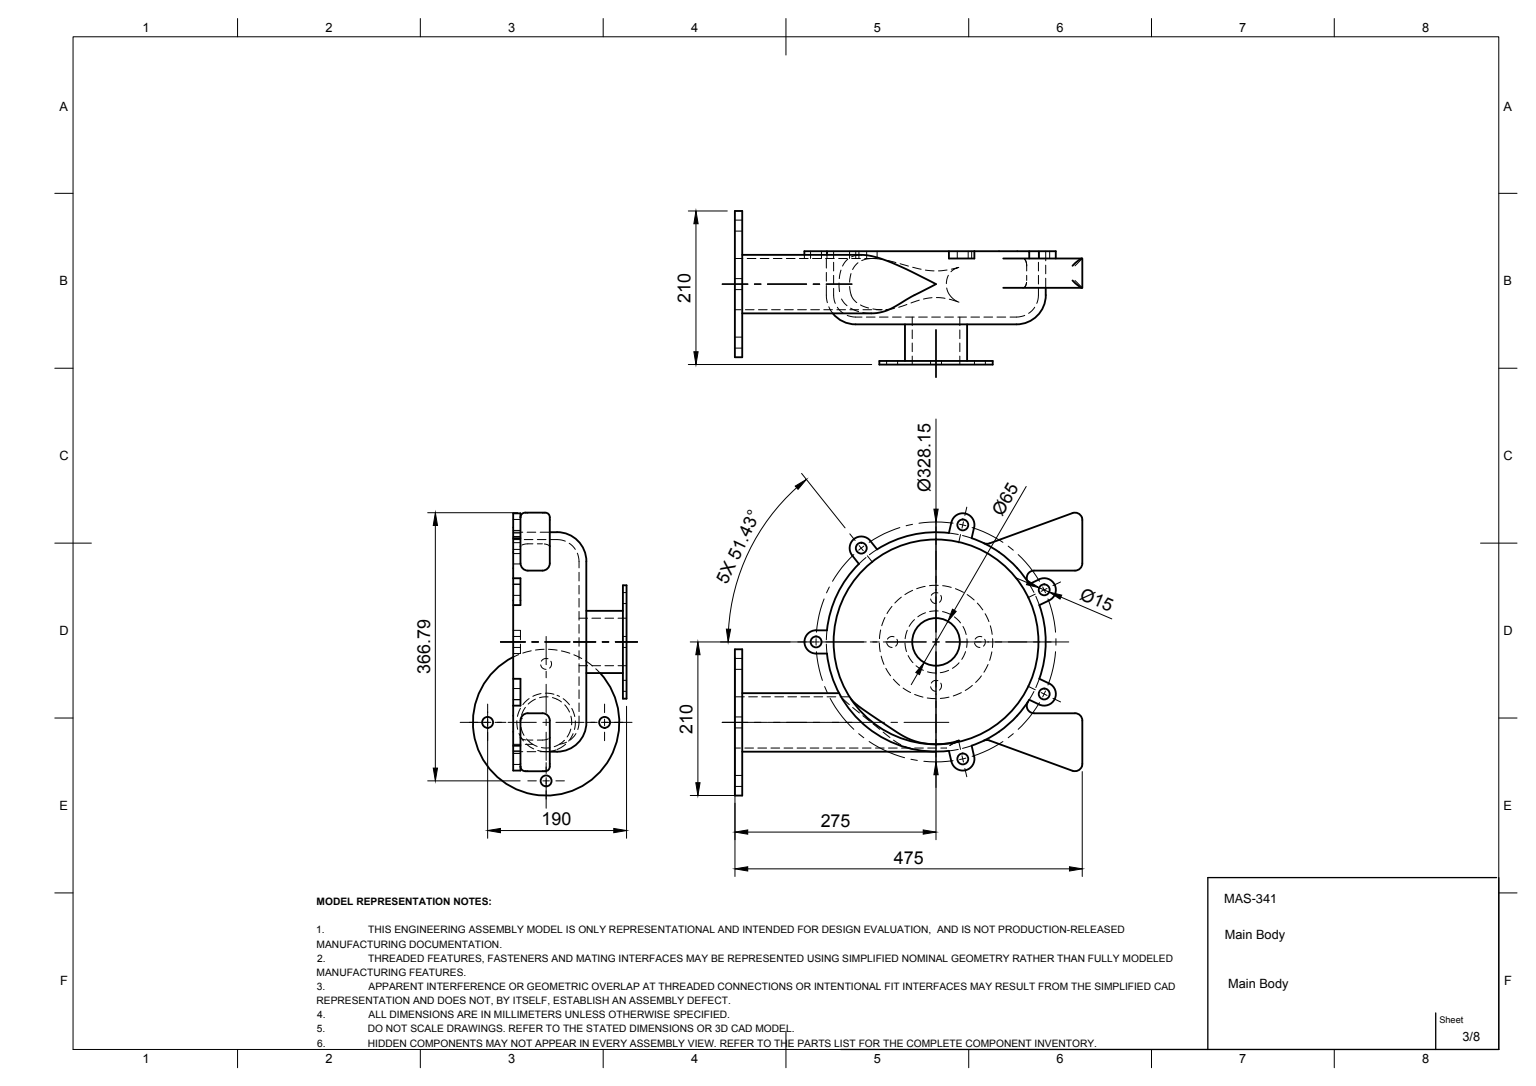
ISO-10303-21;
HEADER;
FILE_DESCRIPTION (('STEP AP214'),
    '1' );
FILE_NAME ('Main Body.step',
    '2026-10-08T00:39:10',
    ( '' ),
    ( '' ),
    'SwSTEP 2.0',
    'SolidWorks 2025',
    '' );
FILE_SCHEMA (( 'AUTOMOTIVE_DESIGN' ));
ENDSEC;

DATA;
#2=CARTESIAN_POINT ( 'NONE',  ( 97.60910239587762760, -133.8115172545202540, 8.514989709614523505 ) ) ;
#5=EDGE_CURVE ( 'NONE', #5734, #13358, #17540, .T. ) ;
#7=DIRECTION ( 'NONE',  ( 0.000000000000000000, 0.000000000000000000, 1.000000000000000000 ) ) ;
#9=CARTESIAN_POINT ( 'NONE',  ( 0.000000000000000000, 0.000000000000000000, 49.99999999999999289 ) ) ;
#16=CARTESIAN_POINT ( 'NONE',  ( 95.93567628220807819, -116.0760901523964179, 30.45195958925782520 ) ) ;
#22=VERTEX_POINT ( 'NONE', #7636 ) ;
#26=CARTESIAN_POINT ( 'NONE',  ( 78.68887634719571622, -147.8252249328912740, 39.99999999999999289 ) ) ;
#29=VECTOR ( 'NONE', #19093, 1000.000000000000000 ) ;
#30=DIRECTION ( 'NONE',  ( 0.000000000000000000, 0.000000000000000000, 1.000000000000000000 ) ) ;
#31=FACE_OUTER_BOUND ( 'NONE', #4493, .T. ) ;
#32=CARTESIAN_POINT ( 'NONE',  ( 130.7934332354521132, -73.44669674648567081, 45.54261232719608188 ) ) ;
#33=CARTESIAN_POINT ( 'NONE',  ( -84.44661573609343463, -123.9709896190455680, 39.82577217277482617 ) ) ;
#38=CARTESIAN_POINT ( 'NONE',  ( -139.9569363493348249, 3.997132000652560802, 23.09995224052206453 ) ) ;
#42=CARTESIAN_POINT ( 'NONE',  ( -133.8587666923834547, -78.85012038918891619, 37.00472930354037260 ) ) ;
#44=ORIENTED_EDGE ( 'NONE', *, *, #7876, .F. ) ;
#51=CARTESIAN_POINT ( 'NONE',  ( -144.9440567817290741, -14.18564734370175628, 2.776575249912347054 ) ) ;
#56=CARTESIAN_POINT ( 'NONE',  ( -95.11181282143326143, 95.73178764297979626, -26.71222966351301409 ) ) ;
#58=DIRECTION ( 'NONE',  ( -0.000000000000000000, -0.000000000000000000, -1.000000000000000000 ) ) ;
#63=CARTESIAN_POINT ( 'NONE',  ( 134.0645693066686874, -77.56608579646832879, 36.26849213499117042 ) ) ;
#64=CARTESIAN_POINT ( 'NONE',  ( -109.9999999999983515, 275.0000000000000000, 92.50000000000004263 ) ) ;
#65=VERTEX_POINT ( 'NONE', #17476 ) ;
#68=ORIENTED_EDGE ( 'NONE', *, *, #8619, .T. ) ;
#70=VECTOR ( 'NONE', #7904, 1000.000000000000000 ) ;
#76=CARTESIAN_POINT ( 'NONE',  ( 152.4599531637113330, -36.50981547336952104, 49.99999999999999289 ) ) ;
#82=CARTESIAN_POINT ( 'NONE',  ( -82.22709333324932857, 122.5189358644918656, -23.80566512433226833 ) ) ;
#83=CARTESIAN_POINT ( 'NONE',  ( -110.0000000000000142, 275.0000000000000000, 5.000000000000000888 ) ) ;
#84=EDGE_CURVE ( 'NONE', #13974, #7495, #15567, .T. ) ;
#86=VECTOR ( 'NONE', #18456, 1000.000000000000000 ) ;
#87=AXIS2_PLACEMENT_3D ( 'NONE', #5255, #2475, #14657 ) ;
#88=LINE ( 'NONE', #6338, #12972 ) ;
#90=CARTESIAN_POINT ( 'NONE',  ( -56.84754764479025368, -154.7316448359455308, 49.99999999999999289 ) ) ;
#102=CARTESIAN_POINT ( 'NONE',  ( 100.3336596192663990, -130.0766330735003180, 3.023488127333376685 ) ) ;
#112=CARTESIAN_POINT ( 'NONE',  ( 96.87131796860539623, -115.7364764686970489, 29.66028648393937317 ) ) ;
#114=DIRECTION ( 'NONE',  ( -3.129754055707530415E-16, 1.000000000000000000, 0.000000000000000000 ) ) ;
#115=CARTESIAN_POINT ( 'NONE',  ( -70.46379820184749576, 132.4194400891323653, -1.343775461033565932 ) ) ;
#117=ORIENTED_EDGE ( 'NONE', *, *, #11334, .T. ) ;
#127=VECTOR ( 'NONE', #6121, 1000.000000000000000 ) ;
#128=ORIENTED_EDGE ( 'NONE', *, *, #9739, .T. ) ;
#130=DIRECTION ( 'NONE',  ( 0.000000000000000000, 1.000000000000000000, 0.000000000000000000 ) ) ;
#132=CARTESIAN_POINT ( 'NONE',  ( -95.59344839194261567, -116.1516065318577233, 31.25619608454541165 ) ) ;
#134=CARTESIAN_POINT ( 'NONE',  ( -140.0000000000000284, 1.714505518806295230E-14, 23.02775637731986436 ) ) ;
#140=CARTESIAN_POINT ( 'NONE',  ( -123.8565975624213849, -84.62454961663081576, 40.61527585688936881 ) ) ;
#147=EDGE_LOOP ( 'NONE', ( #10880, #3979, #3844, #3785, #18936 ) ) ;
#152=CARTESIAN_POINT ( 'NONE',  ( -144.3459975433503359, -14.90824844061875432, 11.80575795572019437 ) ) ;
#156=CARTESIAN_POINT ( 'NONE',  ( -77.50000000000000000, 9.491012693391988181E-15, -105.0000000000000142 ) ) ;
#160=CARTESIAN_POINT ( 'NONE',  ( 104.3997176008718668, -123.8500140569468897, 39.51069475786240304 ) ) ;
#164=CARTESIAN_POINT ( 'NONE',  ( 131.4393841463105730, -72.38802639019482399, 37.47509838629414247 ) ) ;
#165=CARTESIAN_POINT ( 'NONE',  ( -97.49999999999997158, -195.8578643762690206, 4.142135623730952787 ) ) ;
#178=CARTESIAN_POINT ( 'NONE',  ( -85.53020504959707182, -140.9188050298390067, 49.99999999999999289 ) ) ;
#180=CARTESIAN_POINT ( 'NONE',  ( 125.6254798881099362, -81.96796683352708612, -9.529669441935290308 ) ) ;
#183=DIRECTION ( 'NONE',  ( -0.000000000000000000, -1.000000000000000000, -0.000000000000000000 ) ) ;
#189=CARTESIAN_POINT ( 'NONE',  ( 89.20186311087663000, -120.5960167300875980, 45.74363724982469392 ) ) ;
#190=ORIENTED_EDGE ( 'NONE', *, *, #18942, .F. ) ;
#191=CARTESIAN_POINT ( 'NONE',  ( -7.500000000000006217, 164.0736214083062805, 49.99999999999999289 ) ) ;
#196=VECTOR ( 'NONE', #6508, 1000.000000000000000 ) ;
#206=LINE ( 'NONE', #17312, #2056 ) ;
#213=CARTESIAN_POINT ( 'NONE',  ( -71.48370871149657546, 131.8717905529093173, 15.83076793550482542 ) ) ;
#220=EDGE_CURVE ( 'NONE', #5955, #14128, #18233, .T. ) ;
#222=CARTESIAN_POINT ( 'NONE',  ( -139.5020293846663435, 55.14116363050599290, 32.01918336342640004 ) ) ;
#224=FACE_OUTER_BOUND ( 'NONE', #2485, .T. ) ;
#225=LINE ( 'NONE', #20072, #5672 ) ;
#226=CARTESIAN_POINT ( 'NONE',  ( 134.9252074077220129, -65.53799637400003064, 33.62285034463288724 ) ) ;
#228=CARTESIAN_POINT ( 'NONE',  ( -96.81625497257122959, -114.6298681929799557, 36.57121525224014391 ) ) ;
#230=CARTESIAN_POINT ( 'NONE',  ( -90.17913298585699522, -119.8669913176027961, -6.508363994189858559 ) ) ;
#231=DIRECTION ( 'NONE',  ( 0.000000000000000000, 0.000000000000000000, 1.000000000000000000 ) ) ;
#237=EDGE_CURVE ( 'NONE', #5955, #1847, #14266, .T. ) ;
#240=CARTESIAN_POINT ( 'NONE',  ( -133.3512892972259749, -81.69145041113908690, 38.21234876929968038 ) ) ;
#242=EDGE_CURVE ( 'NONE', #7766, #5287, #5764, .T. ) ;
#245=AXIS2_PLACEMENT_3D ( 'NONE', #14497, #6431, #6630 ) ;
#251=CARTESIAN_POINT ( 'NONE',  ( -142.2837698990419710, -17.71062413665211466, 18.52607103759555685 ) ) ;
#260=FACE_OUTER_BOUND ( 'NONE', #11432, .T. ) ;
#265=CARTESIAN_POINT ( 'NONE',  ( 134.2531151303012109, -76.34772591579755385, 35.47645838411665409 ) ) ;
#266=CARTESIAN_POINT ( 'NONE',  ( 132.1955596402976596, -87.17962382538661359, 39.63083459970911804 ) ) ;
#267=ORIENTED_EDGE ( 'NONE', *, *, #4626, .T. ) ;
#269=VERTEX_POINT ( 'NONE', #14956 ) ;
#272=EDGE_CURVE ( 'NONE', #301, #10908, #19490, .T. ) ;
#278=CIRCLE ( 'NONE', #5508, 7.500000000000020428 ) ;
#284=ORIENTED_EDGE ( 'NONE', *, *, #8836, .T. ) ;
#287=EDGE_CURVE ( 'NONE', #13667, #5147, #20127, .T. ) ;
#291=DIRECTION ( 'NONE',  ( -1.000000000000000000, 0.000000000000000000, 0.000000000000000000 ) ) ;
#293=AXIS2_PLACEMENT_3D ( 'NONE', #9235, #1570, #18553 ) ;
#301=VERTEX_POINT ( 'NONE', #13513 ) ;
#303=CARTESIAN_POINT ( 'NONE',  ( 15.91767397667354800, 164.0736214083062805, 39.99999999999999289 ) ) ;
#307=AXIS2_PLACEMENT_3D ( 'NONE', #2543, #16563, #13781 ) ;
#308=CARTESIAN_POINT ( 'NONE',  ( -109.9999999999983515, 275.0000000000000000, 92.50000000000004263 ) ) ;
#309=CARTESIAN_POINT ( 'NONE',  ( -97.49999999999997158, -190.0000000000000000, 10.00000000000000178 ) ) ;
#310=ORIENTED_EDGE ( 'NONE', *, *, #14972, .F. ) ;
#314=CARTESIAN_POINT ( 'NONE',  ( 106.3852469178137170, -120.5001569748608432, 39.95380131650621536 ) ) ;
#317=CARTESIAN_POINT ( 'NONE',  ( -85.08865936083807924, 123.5409191676841374, 36.33575822748944972 ) ) ;
#318=EDGE_LOOP ( 'NONE', ( #10849, #15517, #10410, #10745 ) ) ;
#324=ORIENTED_EDGE ( 'NONE', *, *, #14683, .T. ) ;
#326=CARTESIAN_POINT ( 'NONE',  ( -149.9999999999999716, 1.115331095350416746, 5.575954458838749517 ) ) ;
#330=CARTESIAN_POINT ( 'NONE',  ( 132.6585078626522716, -70.01400725886476550, 42.31265725997803884 ) ) ;
#331=VECTOR ( 'NONE', #5545, 1000.000000000000000 ) ;
#333=CARTESIAN_POINT ( 'NONE',  ( -89.20186311087657316, -120.5960167300876407, -5.743637249824701918 ) ) ;
#346=EDGE_CURVE ( 'NONE', #17320, #3067, #19461, .T. ) ;
#353=CARTESIAN_POINT ( 'NONE',  ( -29.99999999999887379, 265.0000000000000000, 12.49999999999916511 ) ) ;
#356=FACE_OUTER_BOUND ( 'NONE', #14079, .T. ) ;
#358=AXIS2_PLACEMENT_3D ( 'NONE', #19876, #8929, #1155 ) ;
#365=CIRCLE ( 'NONE', #11782, 77.50000000000000000 ) ;
#375=B_SPLINE_CURVE_WITH_KNOTS ( 'NONE', 3,
 ( #12809, #14142, #6181, #4742, #226, #1768, #17536, #3410, #17117, #330, #12398, #9642, #6588, #32, #9545, #19072, #8099, #14247, #3103, #15890, #18860, #4637, #17333, #1869 ),
 .UNSPECIFIED., .F., .F.,
 ( 4, 2, 2, 2, 2, 2, 2, 2, 2, 2, 2, 4 ),
 ( 0.000000000000000000, 0.002185557465519395465, 0.004371114931038790931, 0.008742229862077573188, 0.01311334479311635458, 0.01529890225863574441, 0.01748445972415513250, 0.02185557465519396420, 0.02404113212071339739, 0.02622668958623283059, 0.03059780451727174902, 0.03496891944831063970 ),
 .UNSPECIFIED. ) ;
#380=VERTEX_POINT ( 'NONE', #4526 ) ;
#381=CARTESIAN_POINT ( 'NONE',  ( 133.7324673749508577, -67.93981414779143790, 0.4927691020655204368 ) ) ;
#383=VERTEX_POINT ( 'NONE', #14037 ) ;
#388=EDGE_CURVE ( 'NONE', #16701, #14351, #10960, .T. ) ;
#393=CARTESIAN_POINT ( 'NONE',  ( -141.8714406926361278, -48.70825716237272474, 39.99999999999999289 ) ) ;
#394=VECTOR ( 'NONE', #11693, 1000.000000000000114 ) ;
#395=ORIENTED_EDGE ( 'NONE', *, *, #3158, .T. ) ;
#397=CARTESIAN_POINT ( 'NONE',  ( 0.000000000000000000, 0.000000000000000000, 49.99999999999999289 ) ) ;
#398=EDGE_CURVE ( 'NONE', #9612, #14697, #17220, .T. ) ;
#406=DIRECTION ( 'NONE',  ( -1.000000000000000000, 0.000000000000000000, 0.000000000000000000 ) ) ;
#409=AXIS2_PLACEMENT_3D ( 'NONE', #4331, #19177, #450 ) ;
#410=VECTOR ( 'NONE', #17095, 1000.000000000000000 ) ;
#415=ADVANCED_FACE ( 'NONE', ( #433 ), #17632, .T. ) ;
#418=CARTESIAN_POINT ( 'NONE',  ( -107.4999999999999716, -200.0000000000000000, 40.00000000000000000 ) ) ;
#424=ORIENTED_EDGE ( 'NONE', *, *, #11382, .F. ) ;
#433=FACE_OUTER_BOUND ( 'NONE', #9062, .T. ) ;
#436=FACE_OUTER_BOUND ( 'NONE', #18488, .T. ) ;
#437=CARTESIAN_POINT ( 'NONE',  ( -98.17258311761709422, -133.0662226711790197, 6.375986368445647479 ) ) ;
#438=EDGE_CURVE ( 'NONE', #5218, #9870, #5431, .T. ) ;
#440=CARTESIAN_POINT ( 'NONE',  ( -122.1025966345561073, 68.49760859473882135, 37.84499468909948661 ) ) ;
#447=DIRECTION ( 'NONE',  ( -1.000000000000000000, 0.000000000000000000, 0.000000000000000000 ) ) ;
#450=DIRECTION ( 'NONE',  ( 0.000000000000000000, 0.000000000000000000, -1.000000000000000000 ) ) ;
#455=ORIENTED_EDGE ( 'NONE', *, *, #13971, .F. ) ;
#458=CARTESIAN_POINT ( 'NONE',  ( -189.9999999999988916, 275.0000000000000000, 5.000000000000268230 ) ) ;
#464=CARTESIAN_POINT ( 'NONE',  ( 0.000000000000000000, 0.000000000000000000, -10.00000000000000178 ) ) ;
#471=ORIENTED_EDGE ( 'NONE', *, *, #8214, .T. ) ;
#476=EDGE_LOOP ( 'NONE', ( #2456, #12768 ) ) ;
#483=ORIENTED_EDGE ( 'NONE', *, *, #16283, .F. ) ;
#484=CARTESIAN_POINT ( 'NONE',  ( 134.7540465048387546, -65.88919983460813512, 5.016205221822248816 ) ) ;
#489=AXIS2_PLACEMENT_3D ( 'NONE', #7649, #18713, #18610 ) ;
#494=CARTESIAN_POINT ( 'NONE',  ( -135.7837464099825695, -28.85345328491248651, -18.68477101865893175 ) ) ;
#496=CARTESIAN_POINT ( 'NONE',  ( 93.27226090021298432, -117.4765369300808402, 48.33671567152951098 ) ) ;
#497=ORIENTED_EDGE ( 'NONE', *, *, #17432, .F. ) ;
#505=EDGE_LOOP ( 'NONE', ( #8299, #8837, #2752, #9090 ) ) ;
#510=DIRECTION ( 'NONE',  ( -0.000000000000000000, -0.000000000000000000, -1.000000000000000000 ) ) ;
#513=PRODUCT ( 'Main Body', 'Main Body', '', ( #19350 ) ) ;
#514=DIRECTION ( 'NONE',  ( 1.000000000000000000, 0.000000000000000000, 0.000000000000000000 ) ) ;
#519=CARTESIAN_POINT ( 'NONE',  ( 0.000000000000000000, 164.0736214083062805, 39.99999999999999289 ) ) ;
#527=CARTESIAN_POINT ( 'NONE',  ( -88.95069649744878859, 120.7914063265062055, 39.04816013673605113 ) ) ;
#532=ORIENTED_EDGE ( 'NONE', *, *, #2284, .F. ) ;
#536=CARTESIAN_POINT ( 'NONE',  ( -113.3498877299711864, 98.27513227905838278, 44.89206021334695862 ) ) ;
#540=CARTESIAN_POINT ( 'NONE',  ( -97.52847697650713599, -113.9950050385133693, 2.467650561764177741 ) ) ;
#546=CARTESIAN_POINT ( 'NONE',  ( 159.9599531637113330, -36.50981547336952104, 39.99999999999999289 ) ) ;
#548=EDGE_CURVE ( 'NONE', #12640, #16017, #8706, .T. ) ;
#566=CARTESIAN_POINT ( 'NONE',  ( 140.0000000000000284, 0.000000000000000000, -115.0000000000000142 ) ) ;
#567=PLANE ( 'NONE',  #6525 ) ;
#571=ORIENTED_EDGE ( 'NONE', *, *, #2295, .T. ) ;
#573=VERTEX_POINT ( 'NONE', #17823 ) ;
#575=ORIENTED_EDGE ( 'NONE', *, *, #4277, .F. ) ;
#578=DIRECTION ( 'NONE',  ( 0.9749279121818257288, -0.2225209339563047339, 0.000000000000000000 ) ) ;
#583=ORIENTED_EDGE ( 'NONE', *, *, #19634, .T. ) ;
#584=CARTESIAN_POINT ( 'NONE',  ( -93.38451287766530129, 109.3625709609712544, -31.42891559531335588 ) ) ;
#588=CARTESIAN_POINT ( 'NONE',  ( -136.9468171063203101, -26.51361207507547491, -17.34057338814886862 ) ) ;
#590=CARTESIAN_POINT ( 'NONE',  ( 99.70727046260189752, -112.0668231182905572, 49.97544513886636963 ) ) ;
#592=EDGE_CURVE ( 'NONE', #9122, #5287, #632, .T. ) ;
#602=CARTESIAN_POINT ( 'NONE',  ( -82.33470881469955316, -125.3834122142802272, 33.60191280747055487 ) ) ;
#608=CARTESIAN_POINT ( 'NONE',  ( 104.1558342746901928, -124.2522228486704421, 0.5619391425930568840 ) ) ;
#614=AXIS2_PLACEMENT_3D ( 'NONE', #2103, #14577, #4975 ) ;
#616=DIRECTION ( 'NONE',  ( 0.000000000000000000, 0.000000000000000000, 1.000000000000000000 ) ) ;
#618=CARTESIAN_POINT ( 'NONE',  ( 93.45568245711652366, -117.3306176392091373, 48.42050290853573102 ) ) ;
#620=ADVANCED_FACE ( 'NONE', ( #10231 ), #2366, .T. ) ;
#622=FACE_OUTER_BOUND ( 'NONE', #12847, .T. ) ;
#632=LINE ( 'NONE', #19353, #1191 ) ;
#637=CARTESIAN_POINT ( 'NONE',  ( -95.49560220037844260, -115.9193184531315381, 6.561900623234592445 ) ) ;
#645=AXIS2_PLACEMENT_3D ( 'NONE', #919, #2868, #2668 ) ;
#649=EDGE_CURVE ( 'NONE', #11180, #14061, #3174, .T. ) ;
#654=ADVANCED_FACE ( 'NONE', ( #7666 ), #12466, .F. ) ;
#655=DIRECTION ( 'NONE',  ( -0.000000000000000000, -1.000000000000000000, -0.000000000000000000 ) ) ;
#657=CARTESIAN_POINT ( 'NONE',  ( -126.0064496073183591, -81.39031533630314641, -9.417289231373237257 ) ) ;
#659=CARTESIAN_POINT ( 'NONE',  ( -136.4994460260996902, -31.11111111111110006, -10.83394172763413899 ) ) ;
#663=CARTESIAN_POINT ( 'NONE',  ( -129.0037046021669767, -76.61892870327682203, -0.1306340574592130821 ) ) ;
#664=CARTESIAN_POINT ( 'NONE',  ( 134.6385828715892217, -73.56429320930371318, 7.599106732516738738 ) ) ;
#666=CARTESIAN_POINT ( 'NONE',  ( -176.7850001792984358, -194.3449193228699414, 2.490758961397592675 ) ) ;
#669=ORIENTED_EDGE ( 'NONE', *, *, #5124, .F. ) ;
#672=VECTOR ( 'NONE', #9418, 1000.000000000000000 ) ;
#674=ORIENTED_EDGE ( 'NONE', *, *, #4626, .F. ) ;
#679=LINE ( 'NONE', #6924, #9296 ) ;
#681=ORIENTED_EDGE ( 'NONE', *, *, #13967, .F. ) ;
#686=EDGE_LOOP ( 'NONE', ( #4759, #20168, #5378, #19082, #13161, #7782, #5172, #267, #1533, #7449, #5941, #583, #3735, #5761, #17193, #6714, #16858, #15007, #1728, #12781, #8037, #18671, #16578, #19251, #1715, #18339, #12228, #4895, #11794, #7815, #748, #14906, #395 ) ) ;
#696=DIRECTION ( 'NONE',  ( 0.7818314824680220321, 0.6234898018587433643, 0.000000000000000000 ) ) ;
#700=ORIENTED_EDGE ( 'NONE', *, *, #19231, .F. ) ;
#701=LINE ( 'NONE', #8276, #10766 ) ;
#708=CARTESIAN_POINT ( 'NONE',  ( 103.6579813550140017, -125.0534741538843235, 0.7510394427105699933 ) ) ;
#713=CARTESIAN_POINT ( 'NONE',  ( 97.50000000000001421, -133.9542832461881119, 30.00000000000000000 ) ) ;
#714=CARTESIAN_POINT ( 'NONE',  ( 82.22461745850688430, -125.4556360547411344, 7.112305957179646754 ) ) ;
#722=CARTESIAN_POINT ( 'NONE',  ( 101.0196388379316659, 100.9199429146863167, 49.99999999999999289 ) ) ;
#727=CARTESIAN_POINT ( 'NONE',  ( 96.59911734864401467, -114.8254675080909095, 3.766286132638113848 ) ) ;
#729=CARTESIAN_POINT ( 'NONE',  ( -95.77047472624724378, -116.1200526047209394, 9.227179618507987513 ) ) ;
#733=DIRECTION ( 'NONE',  ( -0.000000000000000000, -0.000000000000000000, -1.000000000000000000 ) ) ;
#737=CARTESIAN_POINT ( 'NONE',  ( -15.91767397667354800, 141.9028892025177413, 49.99999999999999289 ) ) ;
#740=EDGE_CURVE ( 'NONE', #961, #7600, #11543, .T. ) ;
#748=ORIENTED_EDGE ( 'NONE', *, *, #13971, .T. ) ;
#751=CARTESIAN_POINT ( 'NONE',  ( -126.7590367374602494, -80.21250349114244216, -9.076491356015703005 ) ) ;
#752=DIRECTION ( 'NONE',  ( 0.000000000000000000, 0.000000000000000000, 1.000000000000000000 ) ) ;
#753=CIRCLE ( 'NONE', #11206, 7.500000000000006217 ) ;
#755=DIRECTION ( 'NONE',  ( 0.3427509529624095941, 0.9394263059140722794, 0.000000000000000000 ) ) ;
#757=CARTESIAN_POINT ( 'NONE',  ( -77.50000000000000000, 9.491012693391988181E-15, -100.0000000000000000 ) ) ;
#762=EDGE_CURVE ( 'NONE', #18014, #5623, #16769, .T. ) ;
#766=CIRCLE ( 'NONE', #13818, 7.500000000000000000 ) ;
#768=ORIENTED_EDGE ( 'NONE', *, *, #10405, .F. ) ;
#771=AXIS2_PLACEMENT_3D ( 'NONE', #14466, #6901, #11492 ) ;
#776=DIRECTION ( 'NONE',  ( -0.000000000000000000, -0.000000000000000000, -1.000000000000000000 ) ) ;
#777=ORIENTED_EDGE ( 'NONE', *, *, #9922, .T. ) ;
#780=ORIENTED_EDGE ( 'NONE', *, *, #16980, .F. ) ;
#781=PLANE ( 'NONE',  #11393 ) ;
#789=ORIENTED_EDGE ( 'NONE', *, *, #13137, .T. ) ;
#796=VERTEX_POINT ( 'NONE', #3075 ) ;
#799=AXIS2_PLACEMENT_3D ( 'NONE', #5132, #17310, #9715 ) ;
#801=DIRECTION ( 'NONE',  ( -0.000000000000000000, -1.000000000000000000, -0.000000000000000000 ) ) ;
#803=CARTESIAN_POINT ( 'NONE',  ( -130.1901167961280521, -74.50443780700842922, 46.26218360866808865 ) ) ;
#804=CARTESIAN_POINT ( 'NONE',  ( 63.68887634719570912, -147.8252249328912740, 39.99999999999999289 ) ) ;
#808=CARTESIAN_POINT ( 'NONE',  ( -144.1130761623740568, -69.50842595698578918, 49.99999999999999289 ) ) ;
#810=CARTESIAN_POINT ( 'NONE',  ( 82.03125000000005684, -125.5821405433014064, 9.272053618398000907 ) ) ;
#817=VECTOR ( 'NONE', #13786, 999.9999999999998863 ) ;
#823=VECTOR ( 'NONE', #11548, 1000.000000000000000 ) ;
#824=CARTESIAN_POINT ( 'NONE',  ( 95.45795901651801785, -116.1130648478386007, 7.867509371635869719 ) ) ;
#825=CARTESIAN_POINT ( 'NONE',  ( -100.4426743477017965, -129.9257371803582259, 2.884579890773657507 ) ) ;
#827=CARTESIAN_POINT ( 'NONE',  ( -150.0000000000000284, 0.000000000000000000, 49.99999999999999289 ) ) ;
#830=DIRECTION ( 'NONE',  ( 0.000000000000000000, 0.000000000000000000, -1.000000000000000000 ) ) ;
#834=EDGE_LOOP ( 'NONE', ( #11102, #16029, #13341, #7575, #11239, #15936 ) ) ;
#836=DIRECTION ( 'NONE',  ( -0.000000000000000000, -0.000000000000000000, 1.000000000000000000 ) ) ;
#853=CARTESIAN_POINT ( 'NONE',  ( -130.9868171408399462, -91.88282611735539263, 3.469446951953614189E-15 ) ) ;
#855=CARTESIAN_POINT ( 'NONE',  ( 134.6061912685151754, -66.19056267105210623, 4.133867502762946344 ) ) ;
#866=EDGE_LOOP ( 'NONE', ( #10462, #13743, #13664, #7998 ) ) ;
#870=VERTEX_POINT ( 'NONE', #12780 ) ;
#871=ADVANCED_FACE ( 'NONE', ( #15659 ), #3279, .F. ) ;
#881=CARTESIAN_POINT ( 'NONE',  ( 4.189777606611760026E-13, -60.00000000000000000, -105.0000000000000142 ) ) ;
#886=ORIENTED_EDGE ( 'NONE', *, *, #1081, .F. ) ;
#888=DIRECTION ( 'NONE',  ( -0.000000000000000000, -1.000000000000000000, -0.000000000000000000 ) ) ;
#894=CARTESIAN_POINT ( 'NONE',  ( -84.48076729319791411, -123.9477347680102639, 39.88981094656359971 ) ) ;
#897=FACE_OUTER_BOUND ( 'NONE', #6117, .T. ) ;
#899=EDGE_CURVE ( 'NONE', #15648, #18566, #9811, .T. ) ;
#902=CARTESIAN_POINT ( 'NONE',  ( -134.6444961603440618, -66.11310837778573557, 35.67578572572296025 ) ) ;
#909=CARTESIAN_POINT ( 'NONE',  ( 82.17872144123518297, -125.4856950968007396, 7.470559115686841167 ) ) ;
#913=CIRCLE ( 'NONE', #9421, 99.99999999999997158 ) ;
#919=CARTESIAN_POINT ( 'NONE',  ( -107.4999999999999716, -190.0000000000000000, 40.00000000000000000 ) ) ;
#923=CARTESIAN_POINT ( 'NONE',  ( 96.59339607700708541, -114.7676973381603887, -9.527748193600634963 ) ) ;
#928=CARTESIAN_POINT ( 'NONE',  ( -86.48208760716207166, -122.5631135004756658, -3.009211076429890053 ) ) ;
#929=CARTESIAN_POINT ( 'NONE',  ( 107.5000000000000284, -199.9999999999999716, 40.00000000000000000 ) ) ;
#933=CARTESIAN_POINT ( 'NONE',  ( -139.8142396999972163, 1.712230611238718486E-14, -13.33333333333329307 ) ) ;
#935=DIRECTION ( 'NONE',  ( 0.000000000000000000, 0.000000000000000000, -1.000000000000000000 ) ) ;
#949=CIRCLE ( 'NONE', #5870, 15.91767397667354444 ) ;
#953=DIRECTION ( 'NONE',  ( 0.000000000000000000, 0.000000000000000000, 1.000000000000000000 ) ) ;
#954=CARTESIAN_POINT ( 'NONE',  ( 134.5971911056711292, -73.88063391573085426, 7.066933751406428321 ) ) ;
#956=CYLINDRICAL_SURFACE ( 'NONE', #3822, 7.500000000000006217 ) ;
#960=EDGE_CURVE ( 'NONE', #4825, #18093, #17397, .T. ) ;
#961=VERTEX_POINT ( 'NONE', #17797 ) ;
#962=AXIS2_PLACEMENT_3D ( 'NONE', #18141, #4121, #10352 ) ;
#969=ORIENTED_EDGE ( 'NONE', *, *, #14026, .F. ) ;
#970=CARTESIAN_POINT ( 'NONE',  ( 7.500000000000006217, 164.0736214083062805, 49.99999999999999289 ) ) ;
#973=ORIENTED_EDGE ( 'NONE', *, *, #19651, .F. ) ;
#975=CIRCLE ( 'NONE', #5896, 150.0000000000000284 ) ;
#977=CARTESIAN_POINT ( 'NONE',  ( 71.18887634719571622, -147.8252249328912740, 39.99999999999999289 ) ) ;
#983=ORIENTED_EDGE ( 'NONE', *, *, #5166, .F. ) ;
#986=ORIENTED_EDGE ( 'NONE', *, *, #13979, .T. ) ;
#1002=CARTESIAN_POINT ( 'NONE',  ( 77.50000000000000000, 0.000000000000000000, -105.0000000000000142 ) ) ;
#1010=LINE ( 'NONE', #19448, #1921 ) ;
#1015=EDGE_CURVE ( 'NONE', #3673, #7332, #3053, .T. ) ;
#1028=DIRECTION ( 'NONE',  ( -0.000000000000000000, -0.000000000000000000, 1.000000000000000000 ) ) ;
#1032=DIRECTION ( 'NONE',  ( 0.000000000000000000, 0.000000000000000000, 1.000000000000000000 ) ) ;
#1033=EDGE_CURVE ( 'NONE', #6085, #5634, #4169, .T. ) ;
#1038=ADVANCED_FACE ( 'NONE', ( #10705 ), #15108, .T. ) ;
#1039=DIRECTION ( 'NONE',  ( -1.000000000000000000, 0.000000000000000000, 0.000000000000000000 ) ) ;
#1040=ORIENTED_EDGE ( 'NONE', *, *, #237, .F. ) ;
#1041=CARTESIAN_POINT ( 'NONE',  ( 0.000000000000000000, 0.000000000000000000, -49.99999999999999289 ) ) ;
#1047=CARTESIAN_POINT ( 'NONE',  ( -127.6186898578139477, -78.88112642940109254, -0.7766205772862178058 ) ) ;
#1048=CARTESIAN_POINT ( 'NONE',  ( 131.2702496982006153, -90.86622748989321963, -2.335466277633964500E-16 ) ) ;
#1052=CARTESIAN_POINT ( 'NONE',  ( -133.2712073786778433, -68.96827650415615096, 31.07541976963426578 ) ) ;
#1054=MANIFOLD_SOLID_BREP ( 'Fillet3', #7080 ) ;
#1061=ORIENTED_EDGE ( 'NONE', *, *, #13864, .F. ) ;
#1069=LINE ( 'NONE', #4050, #15986 ) ;
#1070=CARTESIAN_POINT ( 'NONE',  ( 120.7779226595531128, 102.2982297021113141, 39.99999999999999289 ) ) ;
#1071=CARTESIAN_POINT ( 'NONE',  ( -42.50000000000000000, 5.204748896376250896E-15, -100.0000000000000000 ) ) ;
#1073=UNCERTAINTY_MEASURE_WITH_UNIT (LENGTH_MEASURE( 1.000000000000000082E-05 ), #7638, 'distance_accuracy_value', 'NONE');
#1074=VECTOR ( 'NONE', #12151, 1000.000000000000114 ) ;
#1075=CARTESIAN_POINT ( 'NONE',  ( 130.6671641404130639, -73.67117004795007063, 45.70932628007447107 ) ) ;
#1081=EDGE_CURVE ( 'NONE', #5634, #13285, #6344, .T. ) ;
#1091=CARTESIAN_POINT ( 'NONE',  ( -42.50000000000000000, 5.204748896376250896E-15, -100.0000000000000000 ) ) ;
#1100=CARTESIAN_POINT ( 'NONE',  ( 0.000000000000000000, 0.000000000000000000, -10.00000000000000178 ) ) ;
#1104=CARTESIAN_POINT ( 'NONE',  ( -133.3655458879726723, -81.62736142943097661, 38.20259313401145107 ) ) ;
#1108=CARTESIAN_POINT ( 'NONE',  ( 133.2435246741110006, -68.89240257401093004, 10.00000000000000178 ) ) ;
#1121=EDGE_CURVE ( 'NONE', #19010, #5530, #7843, .T. ) ;
#1124=CARTESIAN_POINT ( 'NONE',  ( -138.0190090189069849, -24.44405553796960717, -9.999999999999987566 ) ) ;
#1129=TOROIDAL_SURFACE ( 'NONE', #3753, 160.0000000000000284, 10.00000000000000000 ) ;
#1131=CARTESIAN_POINT ( 'NONE',  ( -141.8714406926361278, -48.70825716237271763, 49.99999999999999289 ) ) ;
#1138=EDGE_CURVE ( 'NONE', #15303, #5586, #6629, .T. ) ;
#1140=AXIS2_PLACEMENT_3D ( 'NONE', #7543, #13678, #10302 ) ;
#1144=CARTESIAN_POINT ( 'NONE',  ( 131.4993367897275220, -89.99660315853893167, 0.04843323613514682879 ) ) ;
#1147=EDGE_CURVE ( 'NONE', #16478, #13051, #12872, .T. ) ;
#1151=VERTEX_POINT ( 'NONE', #3451 ) ;
#1152=DIRECTION ( 'NONE',  ( -0.000000000000000000, -1.000000000000000000, -0.000000000000000000 ) ) ;
#1153=CARTESIAN_POINT ( 'NONE',  ( -130.7712900376313598, -73.57687123476972602, 1.577274671842293197 ) ) ;
#1154=CARTESIAN_POINT ( 'NONE',  ( 129.2715203052800632, -76.16417937455307197, 0.08780702205603270472 ) ) ;
#1155=DIRECTION ( 'NONE',  ( -1.000000000000000000, 0.000000000000000000, 0.000000000000000000 ) ) ;
#1157=LINE ( 'NONE', #7207, #5085 ) ;
#1164=ORIENTED_EDGE ( 'NONE', *, *, #4048, .F. ) ;
#1165=ORIENTED_EDGE ( 'NONE', *, *, #5833, .F. ) ;
#1168=EDGE_LOOP ( 'NONE', ( #17349, #1613 ) ) ;
#1172=CARTESIAN_POINT ( 'NONE',  ( -79.44021699520564539, 115.2109178599716017, -12.09771328782125899 ) ) ;
#1173=DIRECTION ( 'NONE',  ( 0.000000000000000000, 0.000000000000000000, -1.000000000000000000 ) ) ;
#1175=LINE ( 'NONE', #14995, #6259 ) ;
#1178=CARTESIAN_POINT ( 'NONE',  ( 125.5756761630927372, -82.07265954316353884, 41.04722885697084678 ) ) ;
#1179=CARTESIAN_POINT ( 'NONE',  ( -176.7850001792985495, -194.3449193228699698, 37.50924103860242553 ) ) ;
#1180=ORIENTED_EDGE ( 'NONE', *, *, #18056, .F. ) ;
#1182=CARTESIAN_POINT ( 'NONE',  ( 166.7850001792985495, -189.9999999999999432, 40.00000000000000000 ) ) ;
#1191=VECTOR ( 'NONE', #16387, 1000.000000000000000 ) ;
#1192=FILL_AREA_STYLE ('',( #15207 ) ) ;
#1193=CARTESIAN_POINT ( 'NONE',  ( -29.99999999999887379, 275.0000000000000000, 4.999999999999158007 ) ) ;
#1194=ORIENTED_EDGE ( 'NONE', *, *, #4603, .T. ) ;
#1197=ORIENTED_EDGE ( 'NONE', *, *, #7928, .T. ) ;
#1199=CARTESIAN_POINT ( 'NONE',  ( -81.46657151846173406, 123.3484521904389339, -23.05424169220087904 ) ) ;
#1203=VERTEX_POINT ( 'NONE', #13139 ) ;
#1206=CARTESIAN_POINT ( 'NONE',  ( -85.14505921096956342, 111.1339209219067925, 29.65373415551709968 ) ) ;
#1208=B_SPLINE_CURVE_WITH_KNOTS ( 'NONE', 3,
 ( #15433, #8979, #12353, #15220, #7254, #3065, #19929, #18612, #6135, #18505, #13892, #20036, #16866, #10412, #12250, #4486, #5722, #2657, #1317, #1104, #19826, #11936, #15026, #9189, #5822, #7653, #1424, #19726 ),
 .UNSPECIFIED., .F., .F.,
 ( 4, 2, 2, 2, 2, 2, 2, 2, 2, 2, 2, 2, 2, 4 ),
 ( 0.000000000000000000, 0.001466376146900913230, 0.002199564220351372772, 0.002932752293801832531, 0.004399128440702757686, 0.005865504587603682408, 0.007331880734504607131, 0.008798256881405530985, 0.01026463302830645831, 0.01173100917520738216, 0.01466376146900919344, 0.01759651376281100299, 0.02052926605661281600, 0.02346201835041462902 ),
 .UNSPECIFIED. ) ;
#1214=CARTESIAN_POINT ( 'NONE',  ( -82.18707601317574074, -125.4802243595265736, 32.59999595717800247 ) ) ;
#1217=CIRCLE ( 'NONE', #4496, 7.500000000000002665 ) ;
#1220=ADVANCED_FACE ( 'NONE', ( #16437, #9987, #19404, #7021, #5198, #11707 ), #5387, .T. ) ;
#1223=ORIENTED_EDGE ( 'NONE', *, *, #14398, .T. ) ;
#1224=CARTESIAN_POINT ( 'NONE',  ( 97.50000000000000000, -115.4778303846449887, 10.00000000000000355 ) ) ;
#1228=CARTESIAN_POINT ( 'NONE',  ( -134.7445384735268590, -31.41486127453163490, -19.78846255602397619 ) ) ;
#1229=PLANE ( 'NONE',  #2766 ) ;
#1230=CIRCLE ( 'NONE', #13637, 7.500000000000001776 ) ;
#1234=CARTESIAN_POINT ( 'NONE',  ( 95.87737486567891665, -116.0928213521003727, 30.55387713521830761 ) ) ;
#1242=CIRCLE ( 'NONE', #18624, 15.91767397667355510 ) ;
#1249=EDGE_LOOP ( 'NONE', ( #14006, #18841 ) ) ;
#1253=CARTESIAN_POINT ( 'NONE',  ( -100.0290433905560974, -111.7820284657242951, 39.61898166952727962 ) ) ;
#1255=FACE_OUTER_BOUND ( 'NONE', #10175, .T. ) ;
#1256=ORIENTED_EDGE ( 'NONE', *, *, #7505, .F. ) ;
#1258=CARTESIAN_POINT ( 'NONE',  ( -134.4925794577901002, -74.66012650512811888, 6.056824688956695013 ) ) ;
#1260=CARTESIAN_POINT ( 'NONE',  ( 133.6471402512195255, -68.10643054410130048, 0.2438139681274874293 ) ) ;
#1262=DIRECTION ( 'NONE',  ( 1.000000000000000000, 0.000000000000000000, 0.000000000000000000 ) ) ;
#1263=CARTESIAN_POINT ( 'NONE',  ( -110.0000000000000142, 0.000000000000000000, 5.000000000000000888 ) ) ;
#1265=DIRECTION ( 'NONE',  ( -1.613511099790691498E-16, 1.000000000000000000, 0.000000000000000000 ) ) ;
#1266=VECTOR ( 'NONE', #16070, 1000.000000000000000 ) ;
#1271=EDGE_CURVE ( 'NONE', #7556, #3875, #679, .T. ) ;
#1275=AXIS2_PLACEMENT_3D ( 'NONE', #8417, #2288, #19366 ) ;
#1277=EDGE_LOOP ( 'NONE', ( #20096, #14289, #14387, #19517 ) ) ;
#1279=DIRECTION ( 'NONE',  ( -0.6718749999999997780, 0.7406645559057084549, 0.000000000000000000 ) ) ;
#1284=CARTESIAN_POINT ( 'NONE',  ( 170.2125097089226244, -199.3942630591406839, 0.000000000000000000 ) ) ;
#1286=EDGE_LOOP ( 'NONE', ( #9182, #2764 ) ) ;
#1294=CIRCLE ( 'NONE', #12387, 15.91767397667355510 ) ;
#1296=ORIENTED_EDGE ( 'NONE', *, *, #6018, .F. ) ;
#1299=ORIENTED_EDGE ( 'NONE', *, *, #10082, .F. ) ;
#1300=VERTEX_POINT ( 'NONE', #5580 ) ;
#1313=CARTESIAN_POINT ( 'NONE',  ( -75.15677698908424986, 129.5154647000477723, -14.68683001631521989 ) ) ;
#1317=CARTESIAN_POINT ( 'NONE',  ( -133.6084294554693770, -80.28749220512220575, 37.65825502569592942 ) ) ;
#1321=DIRECTION ( 'NONE',  ( 0.000000000000000000, 1.000000000000000000, 0.000000000000000000 ) ) ;
#1323=VERTEX_POINT ( 'NONE', #7411 ) ;
#1324=AXIS2_PLACEMENT_3D ( 'NONE', #8681, #14918, #2449 ) ;
#1327=ORIENTED_EDGE ( 'NONE', *, *, #11278, .T. ) ;
#1328=EDGE_CURVE ( 'NONE', #2667, #5218, #13434, .T. ) ;
#1329=DIRECTION ( 'NONE',  ( 0.000000000000000000, 0.000000000000000000, 1.000000000000000000 ) ) ;
#1332=CARTESIAN_POINT ( 'NONE',  ( 96.32595581636887516, -115.9457815549181277, 10.03375122140240627 ) ) ;
#1334=AXIS2_PLACEMENT_3D ( 'NONE', #17984, #8559, #2430 ) ;
#1335=CIRCLE ( 'NONE', #15384, 150.0000000000000284 ) ;
#1336=CARTESIAN_POINT ( 'NONE',  ( -137.6995083356076464, -24.48653385596119847, -14.37849102350654817 ) ) ;
#1339=ADVANCED_FACE ( 'NONE', ( #11901, #13646, #18364, #1378, #7216, #13540 ), #6094, .T. ) ;
#1343=CARTESIAN_POINT ( 'NONE',  ( 82.57283217324942370, -125.2267376009776285, 34.78646775464058294 ) ) ;
#1358=CYLINDRICAL_SURFACE ( 'NONE', #9937, 7.500000000000020428 ) ;
#1366=CARTESIAN_POINT ( 'NONE',  ( 134.4035813917316489, -75.29664220372379191, 5.426846287067242258 ) ) ;
#1367=DIRECTION ( 'NONE',  ( 0.000000000000000000, 0.000000000000000000, 1.000000000000000000 ) ) ;
#1368=FACE_OUTER_BOUND ( 'NONE', #18180, .T. ) ;
#1369=CARTESIAN_POINT ( 'NONE',  ( -134.5311723999394928, -74.37598470588039845, 33.61633749600996879 ) ) ;
#1377=ORIENTED_EDGE ( 'NONE', *, *, #8468, .F. ) ;
#1378=FACE_BOUND ( 'NONE', #16104, .T. ) ;
#1386=CARTESIAN_POINT ( 'NONE',  ( -83.06695335563966864, 111.5579632196524500, -17.35780129461798538 ) ) ;
#1388=CYLINDRICAL_SURFACE ( 'NONE', #4552, 32.50000000000000000 ) ;
#1394=CARTESIAN_POINT ( 'NONE',  ( 131.2732777714562076, -90.85536658133244714, 40.00000000000000000 ) ) ;
#1395=DIRECTION ( 'NONE',  ( -1.000000000000000000, 0.000000000000000000, 0.000000000000000000 ) ) ;
#1399=AXIS2_PLACEMENT_3D ( 'NONE', #2989, #13922, #17212 ) ;
#1415=( BOUNDED_CURVE ( )  B_SPLINE_CURVE ( 3, ( #2820, #16725, #13854, #16632 ),
 .UNSPECIFIED., .F., .F. ) 
 B_SPLINE_CURVE_WITH_KNOTS ( ( 4, 4 ),
 ( 3.141592653589793116, 4.712388980384689674 ),
 .UNSPECIFIED. ) 
 CURVE ( )  GEOMETRIC_REPRESENTATION_ITEM ( )  RATIONAL_B_SPLINE_CURVE ( ( 1.000000000000000000, 0.8047378541243649375, 0.8047378541243649375, 1.000000000000000000 ) ) 
 REPRESENTATION_ITEM ( '' )  );
#1424=CARTESIAN_POINT ( 'NONE',  ( -131.2498835542439508, -90.93927553429134036, 39.99999999999999289 ) ) ;
#1425=CARTESIAN_POINT ( 'NONE',  ( -83.58825350932089293, 112.3093012886738933, 27.97855158061992498 ) ) ;
#1428=FACE_OUTER_BOUND ( 'NONE', #19658, .T. ) ;
#1437=AXIS2_PLACEMENT_3D ( 'NONE', #7897, #130, #6381 ) ;
#1438=CARTESIAN_POINT ( 'NONE',  ( 97.49999999995861799, -115.4778303846967020, 10.07710907076146256 ) ) ;
#1440=VECTOR ( 'NONE', #14395, 1000.000000000000000 ) ;
#1441=CARTESIAN_POINT ( 'NONE',  ( -140.2567302494690011, -18.79374017066554359, -19.65745941995908552 ) ) ;
#1447=CARTESIAN_POINT ( 'NONE',  ( 97.99247315425165539, -133.3057953413762391, 33.10491197978900857 ) ) ;
#1450=DIRECTION ( 'NONE',  ( -0.000000000000000000, -1.000000000000000000, -0.000000000000000000 ) ) ;
#1457=CARTESIAN_POINT ( 'NONE',  ( -97.63534213009850760, -133.7771032679720236, 8.343656291551381443 ) ) ;
#1462=CARTESIAN_POINT ( 'NONE',  ( -100.8144812491492672, -129.3825068912777567, 37.43847687706861649 ) ) ;
#1464=DIRECTION ( 'NONE',  ( 1.000000000000000000, 0.000000000000000000, 0.000000000000000000 ) ) ;
#1467=CARTESIAN_POINT ( 'NONE',  ( -132.5536774537036990, -70.21235394457674772, -2.536984270055062662 ) ) ;
#1468=CARTESIAN_POINT ( 'NONE',  ( 126.7459963399620335, -80.26907437896497299, -1.007255671578283662 ) ) ;
#1471=CARTESIAN_POINT ( 'NONE',  ( -134.4035813917338373, -75.29664220372494299, 34.57315371292968109 ) ) ;
#1483=CARTESIAN_POINT ( 'NONE',  ( -141.8038962792965378, -18.44224925282824756, -9.618166193112273277 ) ) ;
#1489=CARTESIAN_POINT ( 'NONE',  ( -139.8142396999973585, -2.751439320878092509, -13.33333333333314918 ) ) ;
#1492=CARTESIAN_POINT ( 'NONE',  ( -102.5322778132580623, 84.80111478313182261, -29.20113617578324394 ) ) ;
#1498=CARTESIAN_POINT ( 'NONE',  ( 133.2542153457914367, -68.87904111072916180, 40.95291676807742220 ) ) ;
#1500=VECTOR ( 'NONE', #13438, 1000.000000000000000 ) ;
#1502=EDGE_LOOP ( 'NONE', ( #6929, #6599, #13042, #17266 ) ) ;
#1511=DIRECTION ( 'NONE',  ( -1.000000000000000000, 0.000000000000000000, 0.000000000000000000 ) ) ;
#1512=ORIENTED_EDGE ( 'NONE', *, *, #899, .F. ) ;
#1525=CARTESIAN_POINT ( 'NONE',  ( -77.73583826812294717, 116.4358402608469731, 18.59053902802946112 ) ) ;
#1533=ORIENTED_EDGE ( 'NONE', *, *, #12349, .T. ) ;
#1536=CARTESIAN_POINT ( 'NONE',  ( -119.9704660726194447, 76.33180017260909267, -33.75105398353568376 ) ) ;
#1540=CARTESIAN_POINT ( 'NONE',  ( 98.15405843558612276, -133.0926928925950108, 6.371349999020706534 ) ) ;
#1544=CARTESIAN_POINT ( 'NONE',  ( -148.9554720520392834, -17.67108784863415494, 49.99999999999999289 ) ) ;
#1545=FACE_BOUND ( 'NONE', #8932, .T. ) ;
#1550=CARTESIAN_POINT ( 'NONE',  ( 101.9588377999792925, -127.6928792353687641, 38.34752785143055576 ) ) ;
#1561=CARTESIAN_POINT ( 'NONE',  ( 79.05640494598115708, -127.4758205975433043, 49.99999999999999289 ) ) ;
#1562=VERTEX_POINT ( 'NONE', #10884 ) ;
#1568=CARTESIAN_POINT ( 'NONE',  ( -99.15486248080428311, -131.7338018236256119, 35.52123310008073531 ) ) ;
#1570=DIRECTION ( 'NONE',  ( 0.000000000000000000, 0.000000000000000000, -1.000000000000000000 ) ) ;
#1572=FACE_BOUND ( 'NONE', #10667, .T. ) ;
#1573=LINE ( 'NONE', #17231, #70 ) ;
#1576=CARTESIAN_POINT ( 'NONE',  ( -130.0531662534324653, -74.83651286710070849, 39.27204895968475284 ) ) ;
#1577=ORIENTED_EDGE ( 'NONE', *, *, #4142, .T. ) ;
#1578=CARTESIAN_POINT ( 'NONE',  ( 97.50000000000001421, -133.9542832461881119, 10.00000000000000178 ) ) ;
#1582=ORIENTED_EDGE ( 'NONE', *, *, #17137, .F. ) ;
#1583=CARTESIAN_POINT ( 'NONE',  ( -144.0486063771584213, -15.28376807748173682, -3.119549641089998548 ) ) ;
#1589=CARTESIAN_POINT ( 'NONE',  ( -67.50000000000000000, -2.085703952312275003E-13, -100.0000000000000000 ) ) ;
#1590=DIRECTION ( 'NONE',  ( 1.000000000000000000, -0.000000000000000000, -0.000000000000000000 ) ) ;
#1593=ORIENTED_EDGE ( 'NONE', *, *, #649, .T. ) ;
#1594=CARTESIAN_POINT ( 'NONE',  ( -80.58504095603038309, 114.1753459096158565, -13.99979793087933366 ) ) ;
#1597=DIRECTION ( 'NONE',  ( 1.000000000000000000, 0.000000000000000000, 0.000000000000000000 ) ) ;
#1598=DIRECTION ( 'NONE',  ( 0.000000000000000000, 0.000000000000000000, -1.000000000000000000 ) ) ;
#1603=CARTESIAN_POINT ( 'NONE',  ( -122.8001410695374602, -86.14014948502067170, -10.00000000000000178 ) ) ;
#1611=CARTESIAN_POINT ( 'NONE',  ( 107.5000000000000284, -199.9999999999999716, 0.000000000000000000 ) ) ;
#1613=ORIENTED_EDGE ( 'NONE', *, *, #3498, .F. ) ;
#1616=CARTESIAN_POINT ( 'NONE',  ( -97.49999999999995737, -133.9542832461881687, 30.48494313689572977 ) ) ;
#1622=LINE ( 'NONE', #17175, #2585 ) ;
#1624=CARTESIAN_POINT ( 'NONE',  ( -79.97569708437522706, 124.9326907832373053, -21.45256608093599127 ) ) ;
#1626=AXIS2_PLACEMENT_3D ( 'NONE', #11664, #11570, #6779 ) ;
#1627=VECTOR ( 'NONE', #18990, 1000.000000000000000 ) ;
#1628=LINE ( 'NONE', #6639, #7663 ) ;
#1640=ORIENTED_EDGE ( 'NONE', *, *, #7107, .T. ) ;
#1642=EDGE_CURVE ( 'NONE', #3721, #2271, #16487, .T. ) ;
#1645=CARTESIAN_POINT ( 'NONE',  ( 97.50000000000000000, -133.9542832461674777, 9.627394560795542233 ) ) ;
#1651=CARTESIAN_POINT ( 'NONE',  ( -145.8139347833763111, 34.97575719557632823, -12.90182706766672105 ) ) ;
#1655=AXIS2_PLACEMENT_3D ( 'NONE', #6154, #13497, #5743 ) ;
#1656=CARTESIAN_POINT ( 'NONE',  ( 95.64785785032829324, -115.7351073148938099, 34.14437575866686103 ) ) ;
#1661=CARTESIAN_POINT ( 'NONE',  ( -70.66508887821294138, 132.3119617713222738, 12.27828551785295019 ) ) ;
#1664=EDGE_LOOP ( 'NONE', ( #700, #9748, #5019, #14210 ) ) ;
#1666=CARTESIAN_POINT ( 'NONE',  ( -99.75239863728833711, -130.9022835076664819, 3.666872587888030832 ) ) ;
#1673=CARTESIAN_POINT ( 'NONE',  ( -96.05623471149394277, -115.3294058443304522, 35.20016690035954809 ) ) ;
#1675=CARTESIAN_POINT ( 'NONE',  ( -100.7812499999999716, -111.0996833858562809, -10.00000000000000178 ) ) ;
#1680=CARTESIAN_POINT ( 'NONE',  ( -127.3242258594542875, -79.35722205890316161, 40.89109837179960039 ) ) ;
#1683=LINE ( 'NONE', #7814, #9557 ) ;
#1686=ORIENTED_EDGE ( 'NONE', *, *, #17649, .F. ) ;
#1687=EDGE_LOOP ( 'NONE', ( #10284, #14904, #13754, #3544 ) ) ;
#1699=CARTESIAN_POINT ( 'NONE',  ( 132.3557670345053907, -70.70247614045412377, 35.47327301125541510 ) ) ;
#1700=CARTESIAN_POINT ( 'NONE',  ( 132.6188226329610984, -85.30892464212138293, 39.27175784426802352 ) ) ;
#1702=VERTEX_POINT ( 'NONE', #16317 ) ;
#1704=ORIENTED_EDGE ( 'NONE', *, *, #3413, .T. ) ;
#1707=ORIENTED_EDGE ( 'NONE', *, *, #14056, .F. ) ;
#1715=ORIENTED_EDGE ( 'NONE', *, *, #18056, .T. ) ;
#1716=CYLINDRICAL_SURFACE ( 'NONE', #20141, 9.999999999999994671 ) ;
#1721=CARTESIAN_POINT ( 'NONE',  ( 56.84754764479240663, -154.7316448359447634, 49.99999999999999289 ) ) ;
#1722=CARTESIAN_POINT ( 'NONE',  ( -75.72815543956944850, 117.7508209023505970, -2.114875207142446367 ) ) ;
#1728=ORIENTED_EDGE ( 'NONE', *, *, #16609, .T. ) ;
#1730=EDGE_LOOP ( 'NONE', ( #1704, #11388 ) ) ;
#1736=AXIS2_PLACEMENT_3D ( 'NONE', #12948, #13138, #19497 ) ;
#1741=FACE_OUTER_BOUND ( 'NONE', #834, .T. ) ;
#1752=EDGE_CURVE ( 'NONE', #19819, #16530, #16152, .T. ) ;
#1754=CARTESIAN_POINT ( 'NONE',  ( -96.99644974731859293, 114.4709739857757285, 42.93971707143836625 ) ) ;
#1756=ORIENTED_EDGE ( 'NONE', *, *, #272, .T. ) ;
#1761=CARTESIAN_POINT ( 'NONE',  ( -97.77474281578803073, -133.5937942518638124, 7.660502963261819787 ) ) ;
#1762=CARTESIAN_POINT ( 'NONE',  ( -111.7004912049619492, 100.1461745756109138, 44.99999999999997868 ) ) ;
#1768=CARTESIAN_POINT ( 'NONE',  ( 134.6604885881914129, -66.08112487034739502, 35.71876651910825728 ) ) ;
#1771=CARTESIAN_POINT ( 'NONE',  ( -98.78819505924192867, -132.2357222602873605, 34.91288608638632951 ) ) ;
#1774=CARTESIAN_POINT ( 'NONE',  ( 0.000000000000000000, 0.000000000000000000, 0.000000000000000000 ) ) ;
#1780=CARTESIAN_POINT ( 'NONE',  ( -131.4291603288542944, -72.40192386451013817, 37.44902174672004946 ) ) ;
#1788=EDGE_CURVE ( 'NONE', #12640, #10824, #16909, .T. ) ;
#1795=EDGE_CURVE ( 'NONE', #11036, #13843, #13283, .T. ) ;
#1798=CARTESIAN_POINT ( 'NONE',  ( 0.000000000000000000, 0.000000000000000000, 49.99999999999999289 ) ) ;
#1803=CARTESIAN_POINT ( 'NONE',  ( 130.5346569920086779, -73.99347627470881150, 38.71596122396615414 ) ) ;
#1805=CARTESIAN_POINT ( 'NONE',  ( 134.4445132543468446, -75.00751837915895237, 34.30968946414332521 ) ) ;
#1809=ORIENTED_EDGE ( 'NONE', *, *, #3158, .F. ) ;
#1810=LINE ( 'NONE', #8042, #15122 ) ;
#1816=LINE ( 'NONE', #178, #9053 ) ;
#1817=ORIENTED_EDGE ( 'NONE', *, *, #17387, .F. ) ;
#1827=CARTESIAN_POINT ( 'NONE',  ( 0.000000000000000000, 0.000000000000000000, 49.99999999999999289 ) ) ;
#1829=CARTESIAN_POINT ( 'NONE',  ( -134.8030718230775449, -47.09494809331346232, 39.99999999999999289 ) ) ;
#1846=LINE ( 'NONE', #16072, #18111 ) ;
#1847=VERTEX_POINT ( 'NONE', #13622 ) ;
#1851=CARTESIAN_POINT ( 'NONE',  ( -60.00000000000000000, -2.094888803305880013E-13, -105.0000000000000142 ) ) ;
#1852=DIRECTION ( 'NONE',  ( 0.000000000000000000, 0.000000000000000000, 1.000000000000000000 ) ) ;
#1856=PLANE ( 'NONE',  #9087 ) ;
#1857=CARTESIAN_POINT ( 'NONE',  ( -90.95160660477870351, 119.2832880936750399, 40.18161886156921270 ) ) ;
#1858=ORIENTED_EDGE ( 'NONE', *, *, #14026, .T. ) ;
#1859=ORIENTED_EDGE ( 'NONE', *, *, #13152, .T. ) ;
#1867=CARTESIAN_POINT ( 'NONE',  ( -189.9999999999988916, 275.0000000000000000, 5.000000000000268230 ) ) ;
#1869=CARTESIAN_POINT ( 'NONE',  ( 122.8001410695374744, -86.14014948502065749, 49.99999999999999289 ) ) ;
#1871=CARTESIAN_POINT ( 'NONE',  ( -93.27226090021295590, -117.4765369300808828, -8.336715671529505656 ) ) ;
#1878=CARTESIAN_POINT ( 'NONE',  ( -122.8001410695374886, -86.14014948502064328, 50.00000000000000000 ) ) ;
#1881=CARTESIAN_POINT ( 'NONE',  ( -138.9607784057693323, 13.84518047783050321, -14.65874628096230836 ) ) ;
#1904=CARTESIAN_POINT ( 'NONE',  ( 133.7753978164260786, -79.32938232249655641, 37.22355218228292273 ) ) ;
#1914=ADVANCED_FACE ( 'NONE', ( #6459 ), #9617, .F. ) ;
#1917=CARTESIAN_POINT ( 'NONE',  ( -110.0000000000000142, 275.0000000000000000, 5.000000000000000888 ) ) ;
#1921=VECTOR ( 'NONE', #5432, 1000.000000000000000 ) ;
#1925=CARTESIAN_POINT ( 'NONE',  ( 128.2293354902420788, -77.84035270136641316, -8.157851372385163558 ) ) ;
#1928=CARTESIAN_POINT ( 'NONE',  ( -108.3191475787680957, 90.65673307763522359, -34.99999999999998579 ) ) ;
#1955=CARTESIAN_POINT ( 'NONE',  ( 0.000000000000000000, 0.000000000000000000, 50.00000000000000000 ) ) ;
#1963=DIRECTION ( 'NONE',  ( 0.000000000000000000, 1.000000000000000000, 0.000000000000000000 ) ) ;
#1964=CARTESIAN_POINT ( 'NONE',  ( -74.41710797946193168, 130.2395184813107960, 23.29328984172064310 ) ) ;
#1966=AXIS2_PLACEMENT_3D ( 'NONE', #4709, #2970, #9200 ) ;
#1967=VECTOR ( 'NONE', #4023, 1000.000000000000000 ) ;
#1979=EDGE_CURVE ( 'NONE', #16478, #7342, #8378, .T. ) ;
#1981=CARTESIAN_POINT ( 'NONE',  ( -121.1286015293791394, 70.20561501501187252, 38.18765959548887423 ) ) ;
#1987=CARTESIAN_POINT ( 'NONE',  ( -110.0000000000000142, 0.000000000000000000, 39.99999999999997868 ) ) ;
#1989=CARTESIAN_POINT ( 'NONE',  ( 60.00000000000000711, 6.284666409917639535E-13, -105.0000000000000142 ) ) ;
#1991=ADVANCED_FACE ( 'NONE', ( #1741 ), #3380, .T. ) ;
#2000=DIRECTION ( 'NONE',  ( 0.000000000000000000, 0.000000000000000000, 1.000000000000000000 ) ) ;
#2006=CARTESIAN_POINT ( 'NONE',  ( 103.6585128263305222, -125.0478522927852225, 39.23652335784740330 ) ) ;
#2022=LINE ( 'NONE', #8150, #9900 ) ;
#2026=DIRECTION ( 'NONE',  ( -1.000000000000000000, 2.775557561562888984E-15, 0.000000000000000000 ) ) ;
#2029=VERTEX_POINT ( 'NONE', #929 ) ;
#2042=ORIENTED_EDGE ( 'NONE', *, *, #19006, .T. ) ;
#2043=EDGE_LOOP ( 'NONE', ( #19758, #18949 ) ) ;
#2054=FACE_OUTER_BOUND ( 'NONE', #10517, .T. ) ;
#2055=CIRCLE ( 'NONE', #9879, 7.500000000000008882 ) ;
#2056=VECTOR ( 'NONE', #6463, 1000.000000000000000 ) ;
#2061=CARTESIAN_POINT ( 'NONE',  ( 63.68887634719570912, -147.8252249328912740, 39.99999999999999289 ) ) ;
#2064=CARTESIAN_POINT ( 'NONE',  ( 0.000000000000000000, 0.000000000000000000, -39.99999999999999289 ) ) ;
#2068=CARTESIAN_POINT ( 'NONE',  ( -70.79267019417842732, 132.2446714760112059, -3.125962082761043703 ) ) ;
#2081=CARTESIAN_POINT ( 'NONE',  ( -85.14104117559512019, -123.4951580371804170, -1.036462382361432288 ) ) ;
#2083=CARTESIAN_POINT ( 'NONE',  ( -140.0000000000000284, 1.714505518806295230E-14, 23.02775637731986436 ) ) ;
#2084=SHAPE_REPRESENTATION ( 'Main Body', ( #18639 ), #15396 ) ;
#2085=DIRECTION ( 'NONE',  ( 0.000000000000000000, 0.000000000000000000, -1.000000000000000000 ) ) ;
#2087=CARTESIAN_POINT ( 'NONE',  ( -163.5019688434124419, -20.99123081650240863, 39.99999999999999289 ) ) ;
#2088=DIRECTION ( 'NONE',  ( 0.000000000000000000, 0.000000000000000000, -1.000000000000000000 ) ) ;
#2091=CARTESIAN_POINT ( 'NONE',  ( -139.1660152614074093, 12.14097363381727668, -14.35026434167516918 ) ) ;
#2092=AXIS2_PLACEMENT_3D ( 'NONE', #19183, #655, #3920 ) ;
#2096=ORIENTED_EDGE ( 'NONE', *, *, #8530, .T. ) ;
#2097=DIRECTION ( 'NONE',  ( 0.000000000000000000, 0.000000000000000000, 1.000000000000000000 ) ) ;
#2098=CARTESIAN_POINT ( 'NONE',  ( -132.4160198941376336, -70.47193775266624982, -2.820813203610496700 ) ) ;
#2100=AXIS2_PLACEMENT_3D ( 'NONE', #5154, #16091, #11379 ) ;
#2101=DIRECTION ( 'NONE',  ( 0.000000000000000000, 0.000000000000000000, 1.000000000000000000 ) ) ;
#2103=CARTESIAN_POINT ( 'NONE',  ( 0.000000000000000000, 164.0736214083062805, 39.99999999999999289 ) ) ;
#2105=CARTESIAN_POINT ( 'NONE',  ( 67.50000000000000000, 6.284666409917639535E-13, -105.0000000000000142 ) ) ;
#2107=CARTESIAN_POINT ( 'NONE',  ( 98.50852301078391804, -132.6154683359945352, 34.39645643909215522 ) ) ;
#2108=CARTESIAN_POINT ( 'NONE',  ( 7.500000000000001776, 60.00000000000000000, -105.0000000000000142 ) ) ;
#2111=ORIENTED_EDGE ( 'NONE', *, *, #17400, .F. ) ;
#2126=CIRCLE ( 'NONE', #16820, 10.00000000000000178 ) ;
#2127=CARTESIAN_POINT ( 'NONE',  ( -56.84754764479025368, -154.7316448359455308, 39.99999999999999289 ) ) ;
#2130=DIRECTION ( 'NONE',  ( 0.000000000000000000, 0.000000000000000000, 1.000000000000000000 ) ) ;
#2135=DIRECTION ( 'NONE',  ( -1.000000000000000000, 8.881784197001250351E-16, 0.000000000000000000 ) ) ;
#2137=CARTESIAN_POINT ( 'NONE',  ( 93.80830170559224257, -117.0490297264385191, 48.57545654425775439 ) ) ;
#2139=ADVANCED_FACE ( 'NONE', ( #9996, #6542 ), #12763, .T. ) ;
#2150=CARTESIAN_POINT ( 'NONE',  ( -82.03124999999995737, -125.5821405433014348, 30.72794638160199554 ) ) ;
#2152=DIRECTION ( 'NONE',  ( -1.000000000000000000, 0.000000000000000000, 0.000000000000000000 ) ) ;
#2157=CARTESIAN_POINT ( 'NONE',  ( 98.17567701213377518, -133.0624052623788316, 6.362069460218656936 ) ) ;
#2158=VECTOR ( 'NONE', #8073, 1000.000000000000000 ) ;
#2161=ORIENTED_EDGE ( 'NONE', *, *, #5553, .T. ) ;
#2164=CARTESIAN_POINT ( 'NONE',  ( 87.50000000000004263, -133.9542832461881119, 49.99999999999999289 ) ) ;
#2167=DIRECTION ( 'NONE',  ( 0.000000000000000000, 0.000000000000000000, 1.000000000000000000 ) ) ;
#2173=VERTEX_POINT ( 'NONE', #6834 ) ;
#2179=CARTESIAN_POINT ( 'NONE',  ( -120.3490144071938346, 89.54138470860034715, 43.64576342102566286 ) ) ;
#2181=FACE_OUTER_BOUND ( 'NONE', #2915, .T. ) ;
#2183=CARTESIAN_POINT ( 'NONE',  ( -83.29234334534424988, -124.7495837542614225, 2.751972736812206222 ) ) ;
#2186=CARTESIAN_POINT ( 'NONE',  ( -82.17818763663338189, -125.4865065810072622, 7.120596377982462144 ) ) ;
#2188=FACE_OUTER_BOUND ( 'NONE', #14598, .T. ) ;
#2190=CARTESIAN_POINT ( 'NONE',  ( -122.8001410695374886, -86.14014948502065749, 39.99999999999999289 ) ) ;
#2191=ORIENTED_EDGE ( 'NONE', *, *, #5529, .T. ) ;
#2193=CARTESIAN_POINT ( 'NONE',  ( -137.1282911591921732, 23.88247324827570139, -17.14358333410968882 ) ) ;
#2194=EDGE_LOOP ( 'NONE', ( #1180, #7572, #11325, #1194, #10826, #17173, #5243, #19202, #7135, #18239, #14187, #9679, #17719, #19543 ) ) ;
#2218=ORIENTED_EDGE ( 'NONE', *, *, #5166, .T. ) ;
#2233=CARTESIAN_POINT ( 'NONE',  ( -137.5516093427428359, -25.39430756190310845, -16.59029861066365541 ) ) ;
#2235=CARTESIAN_POINT ( 'NONE',  ( 0.000000000000000000, 0.000000000000000000, -10.00000000000000178 ) ) ;
#2237=CARTESIAN_POINT ( 'NONE',  ( 0.000000000000000000, 0.000000000000000000, -100.0000000000000000 ) ) ;
#2238=ORIENTED_EDGE ( 'NONE', *, *, #13967, .T. ) ;
#2242=VECTOR ( 'NONE', #4721, 1000.000000000000000 ) ;
#2243=CYLINDRICAL_SURFACE ( 'NONE', #12165, 99.99999999999997158 ) ;
#2247=CARTESIAN_POINT ( 'NONE',  ( -87.35350281426663344, -121.9411179691607146, 43.97512093379468467 ) ) ;
#2250=ORIENTED_EDGE ( 'NONE', *, *, #5654, .F. ) ;
#2253=CARTESIAN_POINT ( 'NONE',  ( 105.6231002115457329, -121.8324894761443886, 0.1248293295803034469 ) ) ;
#2270=B_SPLINE_CURVE_WITH_KNOTS ( 'NONE', 3,
 ( #6853, #3585, #2253, #608, #708, #9817, #6950, #5319, #12981, #5229, #11454, #19336, #16172, #7054, #13171, #2157, #19438, #8381, #5420, #2448, #11647, #3877, #10122, #16369 ),
 .UNSPECIFIED., .F., .F.,
 ( 4, 2, 2, 2, 2, 2, 2, 2, 2, 2, 2, 4 ),
 ( 0.000000000000000000, 0.005718059174761300212, 0.008577088762141958991, 0.01143611834952262124, 0.01286563314321295150, 0.01429514793690328175, 0.01715417752428397696, 0.01858369231797430202, 0.02001320711166462707, 0.02072796450850978092, 0.02144272190535493477, 0.02287223669904524595 ),
 .UNSPECIFIED. ) ;
#2271=VERTEX_POINT ( 'NONE', #15194 ) ;
#2274=CIRCLE ( 'NONE', #9114, 32.50000000000000000 ) ;
#2280=CARTESIAN_POINT ( 'NONE',  ( -96.05955731895396355, -115.3262050113649906, 4.792200876788737851 ) ) ;
#2284=EDGE_CURVE ( 'NONE', #7600, #961, #10802, .T. ) ;
#2288=DIRECTION ( 'NONE',  ( 0.000000000000000000, 0.000000000000000000, -1.000000000000000000 ) ) ;
#2295=EDGE_CURVE ( 'NONE', #12285, #13478, #18672, .T. ) ;
#2298=CIRCLE ( 'NONE', #4922, 160.0000000000000284 ) ;
#2300=CARTESIAN_POINT ( 'NONE',  ( -134.4038851132261527, -66.60439670040145188, 2.956331823707739836 ) ) ;
#2306=CARTESIAN_POINT ( 'NONE',  ( -125.9311142016074427, -81.50627728740086297, -9.445171272693709597 ) ) ;
#2307=CARTESIAN_POINT ( 'NONE',  ( 132.8875376985348851, -69.70168330571937076, 6.384740227332618367 ) ) ;
#2311=ORIENTED_EDGE ( 'NONE', *, *, #8527, .F. ) ;
#2312=AXIS2_PLACEMENT_3D ( 'NONE', #2757, #13686, #18408 ) ;
#2319=CARTESIAN_POINT ( 'NONE',  ( 156.4179374840099683, -52.02840013023883614, 39.99999999999999289 ) ) ;
#2324=CIRCLE ( 'NONE', #3933, 150.0000000000000284 ) ;
#2328=DIRECTION ( 'NONE',  ( -0.000000000000000000, 0.000000000000000000, -1.000000000000000000 ) ) ;
#2333=CARTESIAN_POINT ( 'NONE',  ( 138.2024300533213932, 89.85329105948596862, 49.99999999999999289 ) ) ;
#2336=CARTESIAN_POINT ( 'NONE',  ( -110.0000000000000142, 265.0000000000000000, -94.99999999999997158 ) ) ;
#2337=ORIENTED_EDGE ( 'NONE', *, *, #2535, .T. ) ;
#2339=ORIENTED_EDGE ( 'NONE', *, *, #17111, .T. ) ;
#2340=DIRECTION ( 'NONE',  ( 0.000000000000000000, 0.000000000000000000, -1.000000000000000000 ) ) ;
#2342=DIRECTION ( 'NONE',  ( -0.6234898018587431423, 0.7818314824680221431, 0.000000000000000000 ) ) ;
#2344=CARTESIAN_POINT ( 'NONE',  ( 0.000000000000000000, 0.000000000000000000, -9.999999999999994671 ) ) ;
#2345=LINE ( 'NONE', #8576, #18466 ) ;
#2357=ORIENTED_EDGE ( 'NONE', *, *, #10357, .F. ) ;
#2361=EDGE_CURVE ( 'NONE', #5750, #5755, #1175, .T. ) ;
#2366=PLANE ( 'NONE',  #7726 ) ;
#2370=CARTESIAN_POINT ( 'NONE',  ( 95.44734317237649179, -116.0775604631400881, 7.549685134005517106 ) ) ;
#2371=CARTESIAN_POINT ( 'NONE',  ( -96.60517994341971360, -114.8199649187100562, 3.756337634281994742 ) ) ;
#2379=FACE_OUTER_BOUND ( 'NONE', #18234, .T. ) ;
#2384=AXIS2_PLACEMENT_3D ( 'NONE', #19470, #1032, #13817 ) ;
#2401=CARTESIAN_POINT ( 'NONE',  ( -122.8001410695374886, -86.14014948502065749, -9.999999999999998224 ) ) ;
#2403=CARTESIAN_POINT ( 'NONE',  ( 132.5080654097352237, -70.41765848030621555, 4.966168250035042142 ) ) ;
#2404=VECTOR ( 'NONE', #8646, 1000.000000000000000 ) ;
#2410=CIRCLE ( 'NONE', #7623, 30.00000000000000000 ) ;
#2421=DIRECTION ( 'NONE',  ( -0.2225209339563047617, -0.9749279121818258398, 0.000000000000000000 ) ) ;
#2424=DIRECTION ( 'NONE',  ( -0.000000000000000000, -0.000000000000000000, 1.000000000000000000 ) ) ;
#2430=DIRECTION ( 'NONE',  ( 1.000000000000000000, 0.000000000000000000, 0.000000000000000000 ) ) ;
#2431=DIRECTION ( 'NONE',  ( -0.000000000000000000, -0.000000000000000000, -1.000000000000000000 ) ) ;
#2444=CARTESIAN_POINT ( 'NONE',  ( -110.0000000000000142, 165.0000000000000000, 5.000000000000000888 ) ) ;
#2448=CARTESIAN_POINT ( 'NONE',  ( 97.67856431661355998, -133.7203759155860894, 8.104337610931111158 ) ) ;
#2449=DIRECTION ( 'NONE',  ( -1.000000000000000000, 0.000000000000000000, 0.000000000000000000 ) ) ;
#2450=LINE ( 'NONE', #7249, #2780 ) ;
#2456=ORIENTED_EDGE ( 'NONE', *, *, #3733, .T. ) ;
#2457=CARTESIAN_POINT ( 'NONE',  ( 150.0000000000000284, 1.836970198721029747E-14, 49.99999999999999289 ) ) ;
#2458=PLANE ( 'NONE',  #6966 ) ;
#2471=CARTESIAN_POINT ( 'NONE',  ( -137.5777631771917413, -26.05850252028229264, 26.56366211542366784 ) ) ;
#2475=DIRECTION ( 'NONE',  ( 0.000000000000000000, 0.000000000000000000, 1.000000000000000000 ) ) ;
#2481=LINE ( 'NONE', #16309, #16284 ) ;
#2485=EDGE_LOOP ( 'NONE', ( #17362, #1686, #13782, #10159 ) ) ;
#2490=CIRCLE ( 'NONE', #13918, 7.500000000000006217 ) ;
#2492=CARTESIAN_POINT ( 'NONE',  ( -97.49999999999997158, -200.0000000000000000, 40.00000000000000000 ) ) ;
#2495=FACE_OUTER_BOUND ( 'NONE', #15231, .T. ) ;
#2502=CARTESIAN_POINT ( 'NONE',  ( -134.7221128596263782, -65.95429948960607192, 35.15983169740453462 ) ) ;
#2503=VERTEX_POINT ( 'NONE', #4455 ) ;
#2505=EDGE_LOOP ( 'NONE', ( #15875, #17494, #284, #19923 ) ) ;
#2508=ORIENTED_EDGE ( 'NONE', *, *, #3271, .T. ) ;
#2512=CARTESIAN_POINT ( 'NONE',  ( -139.0134832045226290, -23.59969680251337820, 24.57866847611368755 ) ) ;
#2528=CARTESIAN_POINT ( 'NONE',  ( 123.3142212418662922, -85.40728428760859003, 40.34936862486454601 ) ) ;
#2535=EDGE_CURVE ( 'NONE', #14190, #3818, #13623, .T. ) ;
#2541=CARTESIAN_POINT ( 'NONE',  ( -86.50547518363038080, -122.5441694604242571, 42.98359700323086940 ) ) ;
#2542=CYLINDRICAL_SURFACE ( 'NONE', #15883, 39.99999999999997868 ) ;
#2543=CARTESIAN_POINT ( 'NONE',  ( -144.1130761623740568, -69.50842595698580340, 10.00000000000000178 ) ) ;
#2545=CARTESIAN_POINT ( 'NONE',  ( -130.7962991791398792, -73.43504534872147360, 45.49776675456224950 ) ) ;
#2547=EDGE_CURVE ( 'NONE', #3721, #8371, #3538, .T. ) ;
#2551=CARTESIAN_POINT ( 'NONE',  ( 82.03125000000004263, -125.5821405433013780, 10.00000000000000178 ) ) ;
#2558=FACE_BOUND ( 'NONE', #1286, .T. ) ;
#2565=CIRCLE ( 'NONE', #11390, 7.500000000000020428 ) ;
#2566=CARTESIAN_POINT ( 'NONE',  ( 103.5848300920814751, -125.1657093462233945, 0.7932558400431272139 ) ) ;
#2567=CARTESIAN_POINT ( 'NONE',  ( -99.73778183779744211, -112.0462389701484511, -10.00000000039103298 ) ) ;
#2569=AXIS2_PLACEMENT_3D ( 'NONE', #7492, #8182, #10554 ) ;
#2571=CARTESIAN_POINT ( 'NONE',  ( -135.3256110043510034, -31.31229190813938956, -18.21647407188902434 ) ) ;
#2576=LINE ( 'NONE', #8807, #10203 ) ;
#2579=ORIENTED_EDGE ( 'NONE', *, *, #3781, .T. ) ;
#2583=ORIENTED_EDGE ( 'NONE', *, *, #11704, .F. ) ;
#2585=VECTOR ( 'NONE', #18915, 1000.000000000000000 ) ;
#2587=ORIENTED_EDGE ( 'NONE', *, *, #5242, .T. ) ;
#2588=ORIENTED_EDGE ( 'NONE', *, *, #1138, .F. ) ;
#2595=CARTESIAN_POINT ( 'NONE',  ( -96.59339607701299713, -114.7676973381553296, 49.52774819360320890 ) ) ;
#2598=AXIS2_PLACEMENT_3D ( 'NONE', #15886, #17430, #3405 ) ;
#2601=FACE_OUTER_BOUND ( 'NONE', #13233, .T. ) ;
#2616=EDGE_CURVE ( 'NONE', #19796, #2833, #1217, .T. ) ;
#2619=VERTEX_POINT ( 'NONE', #2108 ) ;
#2626=CARTESIAN_POINT ( 'NONE',  ( -134.7188131032332876, -72.93593548660989256, 9.503886819007655973 ) ) ;
#2631=CARTESIAN_POINT ( 'NONE',  ( 132.7526696464367149, -84.67545766722484757, 39.11277240342198525 ) ) ;
#2643=ADVANCED_FACE ( 'NONE', ( #260 ), #14478, .F. ) ;
#2644=CARTESIAN_POINT ( 'NONE',  ( 166.7850001792985495, -189.9999999999999432, 0.000000000000000000 ) ) ;
#2645=PRESENTATION_STYLE_ASSIGNMENT (( #16656 ) ) ;
#2648=DIRECTION ( 'NONE',  ( 0.2225209339563044841, 0.9749279121818258398, 0.000000000000000000 ) ) ;
#2654=ORIENTED_EDGE ( 'NONE', *, *, #5991, .T. ) ;
#2657=CARTESIAN_POINT ( 'NONE',  ( -133.6865796038707117, -79.84358686291113827, 37.46324078528252954 ) ) ;
#2659=EDGE_LOOP ( 'NONE', ( #7483, #6678 ) ) ;
#2667=VERTEX_POINT ( 'NONE', #19679 ) ;
#2668=DIRECTION ( 'NONE',  ( -1.000000000000000000, 0.000000000000000000, 0.000000000000000000 ) ) ;
#2671=CARTESIAN_POINT ( 'NONE',  ( 93.44030642264493736, -117.3428525121075268, -8.413488319981127006 ) ) ;
#2672=CARTESIAN_POINT ( 'NONE',  ( -106.9434821670503339, -119.5159909196298997, -6.573008631163750622E-15 ) ) ;
#2674=CARTESIAN_POINT ( 'NONE',  ( -136.3130597734152047, -31.14279861364121871, -13.33873441683735983 ) ) ;
#2677=CARTESIAN_POINT ( 'NONE',  ( 128.2779226595531270, 102.2982297021113141, 39.99999999999999289 ) ) ;
#2678=CARTESIAN_POINT ( 'NONE',  ( 0.000000000000000000, 0.000000000000000000, 49.99999999999999289 ) ) ;
#2688=ORIENTED_EDGE ( 'NONE', *, *, #1121, .T. ) ;
#2689=CARTESIAN_POINT ( 'NONE',  ( 134.5348546532065654, -74.34984901039663896, 6.412720522032803849 ) ) ;
#2692=DIRECTION ( 'NONE',  ( 0.000000000000000000, 0.000000000000000000, 1.000000000000000000 ) ) ;
#2697=CARTESIAN_POINT ( 'NONE',  ( -135.0821395827941842, -65.21370709267439736, 8.503067959630589812 ) ) ;
#2698=CARTESIAN_POINT ( 'NONE',  ( 134.1895921339707911, -76.75826352744203973, 4.256527938263594990 ) ) ;
#2704=ORIENTED_EDGE ( 'NONE', *, *, #6449, .T. ) ;
#2708=ORIENTED_EDGE ( 'NONE', *, *, #9270, .T. ) ;
#2716=ORIENTED_EDGE ( 'NONE', *, *, #1795, .T. ) ;
#2717=AXIS2_PLACEMENT_3D ( 'NONE', #8569, #16157, #8370 ) ;
#2721=CARTESIAN_POINT ( 'NONE',  ( -78.89303534320342237, 115.6558536819018030, -11.08742706010982104 ) ) ;
#2735=VERTEX_POINT ( 'NONE', #18246 ) ;
#2739=VECTOR ( 'NONE', #13777, 1000.000000000000227 ) ;
#2741=ORIENTED_EDGE ( 'NONE', *, *, #11500, .F. ) ;
#2744=FACE_OUTER_BOUND ( 'NONE', #2969, .T. ) ;
#2747=CARTESIAN_POINT ( 'NONE',  ( -140.0000000000000284, 1.714505518806295230E-14, 23.02775637731986436 ) ) ;
#2749=CARTESIAN_POINT ( 'NONE',  ( -133.7324673749508577, -67.93981414779142369, 39.50723089793449816 ) ) ;
#2752=ORIENTED_EDGE ( 'NONE', *, *, #9416, .T. ) ;
#2753=EDGE_CURVE ( 'NONE', #11036, #9322, #8832, .T. ) ;
#2757=CARTESIAN_POINT ( 'NONE',  ( 71.18887634719571622, -147.8252249328912740, 39.99999999999999289 ) ) ;
#2760=ADVANCED_FACE ( 'NONE', ( #16619 ), #956, .F. ) ;
#2764=ORIENTED_EDGE ( 'NONE', *, *, #4402, .T. ) ;
#2765=CARTESIAN_POINT ( 'NONE',  ( -98.15405843558684751, -133.0926928925743198, 33.62865000098088331 ) ) ;
#2766=AXIS2_PLACEMENT_3D ( 'NONE', #9, #2980, #4405 ) ;
#2767=ORIENTED_EDGE ( 'NONE', *, *, #762, .F. ) ;
#2768=FACE_OUTER_BOUND ( 'NONE', #14640, .T. ) ;
#2780=VECTOR ( 'NONE', #11649, 999.9999999999998863 ) ;
#2791=EDGE_LOOP ( 'NONE', ( #11971, #10201, #5018, #8038 ) ) ;
#2805=CARTESIAN_POINT ( 'NONE',  ( -132.5095042660450986, -70.41495930836687478, 4.970722503819324345 ) ) ;
#2806=CARTESIAN_POINT ( 'NONE',  ( 131.8028587768798161, -71.61967917965999675, -4.009458607015777609 ) ) ;
#2809=DIRECTION ( 'NONE',  ( -0.000000000000000000, -1.000000000000000000, -0.000000000000000000 ) ) ;
#2810=DIRECTION ( 'NONE',  ( 1.000000000000000000, 0.000000000000000000, 0.000000000000000000 ) ) ;
#2815=AXIS2_PLACEMENT_3D ( 'NONE', #9154, #12110, #4345 ) ;
#2818=B_SPLINE_CURVE_WITH_KNOTS ( 'NONE', 3,
 ( #12812, #12606, #4854, #14149, #17339, #15996, #19171, #11283, #14254, #11385, #15895 ),
 .UNSPECIFIED., .F., .F.,
 ( 4, 2, 1, 2, 2, 4 ),
 ( -7.745966853365171458E-05, 0.001996111220376526555, 0.004069682109286705367, 0.008216823887107061256, 0.01651110744274777303, 0.03309967455402919312 ),
 .UNSPECIFIED. ) ;
#2820=CARTESIAN_POINT ( 'NONE',  ( -107.4999999999999716, -200.0000000000000000, 40.00000000000000000 ) ) ;
#2825=CARTESIAN_POINT ( 'NONE',  ( -83.39030327046282309, 111.1915035958187019, -17.74126483281444777 ) ) ;
#2827=CARTESIAN_POINT ( 'NONE',  ( -132.6188226329609847, -85.30892464212142556, 0.7282421557319730399 ) ) ;
#2831=CARTESIAN_POINT ( 'NONE',  ( 126.4587173007283667, -80.71184697945604114, 41.01728415539461992 ) ) ;
#2833=VERTEX_POINT ( 'NONE', #16816 ) ;
#2839=ORIENTED_EDGE ( 'NONE', *, *, #5666, .T. ) ;
#2847=VERTEX_POINT ( 'NONE', #16920 ) ;
#2851=VECTOR ( 'NONE', #13377, 1000.000000000000000 ) ;
#2852=FACE_BOUND ( 'NONE', #12231, .T. ) ;
#2858=ORIENTED_EDGE ( 'NONE', *, *, #10082, .T. ) ;
#2863=VERTEX_POINT ( 'NONE', #20083 ) ;
#2866=AXIS2_PLACEMENT_3D ( 'NONE', #5902, #18376, #15818 ) ;
#2868=DIRECTION ( 'NONE',  ( 0.000000000000000000, 0.000000000000000000, -1.000000000000000000 ) ) ;
#2872=CARTESIAN_POINT ( 'NONE',  ( 84.12762954502645130, -124.1876770196613222, 0.8036315111169505254 ) ) ;
#2873=CARTESIAN_POINT ( 'NONE',  ( -100.7812499999999716, -111.0996833858562951, -6.938893903907228378E-15 ) ) ;
#2876=CARTESIAN_POINT ( 'NONE',  ( -141.6670312114224828, -18.66040080199755380, -10.97841296083584517 ) ) ;
#2878=DIRECTION ( 'NONE',  ( -0.6718749999999991118, -0.7406645559057090100, -6.938893903907223447E-16 ) ) ;
#2879=CARTESIAN_POINT ( 'NONE',  ( 0.000000000000000000, 0.000000000000000000, 49.99999999999999289 ) ) ;
#2881=CARTESIAN_POINT ( 'NONE',  ( 84.96040761327756741, -123.6194689893705174, 40.73966003348574816 ) ) ;
#2883=EDGE_CURVE ( 'NONE', #14190, #3030, #20188, .T. ) ;
#2898=ADVANCED_FACE ( 'NONE', ( #12409 ), #15378, .F. ) ;
#2901=CARTESIAN_POINT ( 'NONE',  ( -77.50000000000000000, 9.491012693391988181E-15, -105.0000000000000142 ) ) ;
#2906=CARTESIAN_POINT ( 'NONE',  ( 132.3196846491737233, -70.65764850137227882, -3.065492718625203228 ) ) ;
#2907=LINE ( 'NONE', #15377, #10157 ) ;
#2910=CARTESIAN_POINT ( 'NONE',  ( -134.4924637689158260, -74.66092226662962617, 33.94378522399878761 ) ) ;
#2912=ORIENTED_EDGE ( 'NONE', *, *, #19137, .T. ) ;
#2914=DIRECTION ( 'NONE',  ( 0.000000000000000000, 0.000000000000000000, 1.000000000000000000 ) ) ;
#2915=EDGE_LOOP ( 'NONE', ( #4623, #8268, #6882, #17161 ) ) ;
#2919=ADVANCED_FACE ( 'NONE', ( #1368 ), #5979, .F. ) ;
#2920=CIRCLE ( 'NONE', #1626, 7.500000000000002665 ) ;
#2939=ORIENTED_EDGE ( 'NONE', *, *, #346, .F. ) ;
#2945=ORIENTED_EDGE ( 'NONE', *, *, #9252, .F. ) ;
#2952=VECTOR ( 'NONE', #733, 1000.000000000000000 ) ;
#2955=EDGE_LOOP ( 'NONE', ( #13923, #13203, #10488, #8012 ) ) ;
#2956=FACE_BOUND ( 'NONE', #2043, .T. ) ;
#2957=CARTESIAN_POINT ( 'NONE',  ( 0.000000000000000000, 0.000000000000000000, 39.99999999999999289 ) ) ;
#2958=FACE_OUTER_BOUND ( 'NONE', #18422, .T. ) ;
#2959=DIRECTION ( 'NONE',  ( 0.000000000000000000, 0.000000000000000000, 1.000000000000000000 ) ) ;
#2960=CARTESIAN_POINT ( 'NONE',  ( -134.8030718230775449, -47.09494809331346232, 39.99999999999999289 ) ) ;
#2961=CARTESIAN_POINT ( 'NONE',  ( -105.6803803075390107, 91.83969138069829796, 39.74985483127044006 ) ) ;
#2964=FACE_OUTER_BOUND ( 'NONE', #9152, .T. ) ;
#2966=CIRCLE ( 'NONE', #9823, 40.00000000000000000 ) ;
#2969=EDGE_LOOP ( 'NONE', ( #6399, #16106, #14925, #16093 ) ) ;
#2970=DIRECTION ( 'NONE',  ( -0.000000000000000000, -0.000000000000000000, -1.000000000000000000 ) ) ;
#2972=VERTEX_POINT ( 'NONE', #4436 ) ;
#2973=CARTESIAN_POINT ( 'NONE',  ( 86.28560748592117591, -122.6989046848860596, -2.704177608915436792 ) ) ;
#2978=DIRECTION ( 'NONE',  ( 0.000000000000000000, 0.000000000000000000, 1.000000000000000000 ) ) ;
#2980=DIRECTION ( 'NONE',  ( 0.000000000000000000, 0.000000000000000000, 1.000000000000000000 ) ) ;
#2981=ORIENTED_EDGE ( 'NONE', *, *, #18155, .T. ) ;
#2985=CARTESIAN_POINT ( 'NONE',  ( 82.84981732089829620, -125.0436758660689094, 35.85664428374888502 ) ) ;
#2989=CARTESIAN_POINT ( 'NONE',  ( 87.50000000000002842, -133.9542832461881119, 10.00000000000000178 ) ) ;
#2991=VERTEX_POINT ( 'NONE', #6593 ) ;
#2992=EDGE_CURVE ( 'NONE', #18071, #18093, #3952, .T. ) ;
#2997=CARTESIAN_POINT ( 'NONE',  ( -97.83161216922238168, -133.5187961265288550, 7.436012734232853028 ) ) ;
#3004=CARTESIAN_POINT ( 'NONE',  ( -88.01533840461537750, -121.4634816193508300, 44.65227205411735412 ) ) ;
#3008=CARTESIAN_POINT ( 'NONE',  ( -132.7769743428863194, -69.91161917917753499, 5.893941834771159627 ) ) ;
#3009=CARTESIAN_POINT ( 'NONE',  ( 131.8276101104381155, -71.67687255337031615, 3.301485790455078728 ) ) ;
#3012=CARTESIAN_POINT ( 'NONE',  ( -132.2954651231983405, -86.73864221001061026, 39.54657277217020805 ) ) ;
#3016=EDGE_CURVE ( 'NONE', #13254, #5912, #15388, .T. ) ;
#3017=EDGE_CURVE ( 'NONE', #6900, #12395, #365, .T. ) ;
#3019=VERTEX_POINT ( 'NONE', #19173 ) ;
#3021=B_SPLINE_CURVE_WITH_KNOTS ( 'NONE', 3,
 ( #3531, #13118, #3632, #16016, #17751, #11302, #659, #17559 ),
 .UNSPECIFIED., .F., .F.,
 ( 4, 2, 2, 4 ),
 ( 0.000000000000000000, 0.004946988332758800802, 0.007420482499138205540, 0.009893976665517610278 ),
 .UNSPECIFIED. ) ;
#3026=ORIENTED_EDGE ( 'NONE', *, *, #6286, .F. ) ;
#3027=AXIS2_PLACEMENT_3D ( 'NONE', #11859, #830, #3807 ) ;
#3028=CARTESIAN_POINT ( 'NONE',  ( -139.7162331485264986, -5.470663635007961823, -13.49539711827200250 ) ) ;
#3030=VERTEX_POINT ( 'NONE', #8010 ) ;
#3031=CARTESIAN_POINT ( 'NONE',  ( -92.41014453654959482, 99.55326438240551568, -25.26926237334177472 ) ) ;
#3043=AXIS2_PLACEMENT_3D ( 'NONE', #15054, #5649, #6989 ) ;
#3047=ORIENTED_EDGE ( 'NONE', *, *, #14000, .F. ) ;
#3049=ORIENTED_EDGE ( 'NONE', *, *, #10587, .F. ) ;
#3051=TOROIDAL_SURFACE ( 'NONE', #12510, 160.0000000000000284, 10.00000000000000000 ) ;
#3053=LINE ( 'NONE', #9177, #2739 ) ;
#3062=CYLINDRICAL_SURFACE ( 'NONE', #489, 9.999999999999994671 ) ;
#3063=CARTESIAN_POINT ( 'NONE',  ( -29.99999999999887379, 265.0000000000000000, -2.500000000000847766 ) ) ;
#3065=CARTESIAN_POINT ( 'NONE',  ( -134.6416478978700297, -73.54075392783711607, 32.36000221440195190 ) ) ;
#3066=CARTESIAN_POINT ( 'NONE',  ( -76.84700801462552988, 117.0241645140891364, 16.25045822160150166 ) ) ;
#3067=VERTEX_POINT ( 'NONE', #5063 ) ;
#3069=( GEOMETRIC_REPRESENTATION_CONTEXT ( 3 ) GLOBAL_UNCERTAINTY_ASSIGNED_CONTEXT ( ( #1073 ) ) GLOBAL_UNIT_ASSIGNED_CONTEXT ( ( #7638, #18491, #13564 ) ) REPRESENTATION_CONTEXT ( 'NONE', 'WORKASPACE' ) );
#3074=DIRECTION ( 'NONE',  ( 0.000000000000000000, 0.000000000000000000, 1.000000000000000000 ) ) ;
#3075=CARTESIAN_POINT ( 'NONE',  ( 167.4599531637113330, -36.50981547336952104, 39.99999999999999289 ) ) ;
#3078=CARTESIAN_POINT ( 'NONE',  ( 82.03125000007472067, -125.5821405432526205, 9.254789121596214585 ) ) ;
#3082=DIRECTION ( 'NONE',  ( 0.000000000000000000, 0.000000000000000000, 1.000000000000000000 ) ) ;
#3087=CARTESIAN_POINT ( 'NONE',  ( 98.78543727593098822, -132.2400759706155782, 34.91745822596744375 ) ) ;
#3097=DIRECTION ( 'NONE',  ( 0.2225209339563050392, 0.9749279121818257288, -0.000000000000000000 ) ) ;
#3100=CIRCLE ( 'NONE', #8366, 7.500000000000003553 ) ;
#3103=CARTESIAN_POINT ( 'NONE',  ( 127.8482905096654747, -78.45565238711300537, 48.39782711105171131 ) ) ;
#3105=CARTESIAN_POINT ( 'NONE',  ( -95.76651288691110153, -116.1232671447739335, 30.76217253845484834 ) ) ;
#3109=EDGE_CURVE ( 'NONE', #11373, #4416, #14256, .T. ) ;
#3111=CARTESIAN_POINT ( 'NONE',  ( -135.1060089021507906, -65.16414933482950289, 9.250158916602527981 ) ) ;
#3112=CARTESIAN_POINT ( 'NONE',  ( 123.3088579007138748, -85.41493018851996055, -0.3457237010573973590 ) ) ;
#3115=CARTESIAN_POINT ( 'NONE',  ( -129.0008258634001379, -76.61840651136952829, 40.10093462088531169 ) ) ;
#3117=LINE ( 'NONE', #12203, #86 ) ;
#3128=EDGE_CURVE ( 'NONE', #20118, #5750, #18937, .T. ) ;
#3150=CARTESIAN_POINT ( 'NONE',  ( -101.1837452960046022, -128.8430157189652618, 37.75944112220433624 ) ) ;
#3158=EDGE_CURVE ( 'NONE', #5389, #12640, #3712, .T. ) ;
#3159=EDGE_CURVE ( 'NONE', #3030, #15236, #5353, .T. ) ;
#3162=CARTESIAN_POINT ( 'NONE',  ( -77.82371257323825375, 127.0966514542041779, -18.77062444076983283 ) ) ;
#3163=DIRECTION ( 'NONE',  ( -1.000000000000000000, 0.000000000000000000, 0.000000000000000000 ) ) ;
#3167=CARTESIAN_POINT ( 'NONE',  ( -75.89859996291112054, 117.6422707177539735, 13.05450749028729795 ) ) ;
#3171=CIRCLE ( 'NONE', #15227, 9.999999999999996447 ) ;
#3172=ORIENTED_EDGE ( 'NONE', *, *, #7876, .T. ) ;
#3174=CIRCLE ( 'NONE', #14599, 7.500000000000000000 ) ;
#3176=CARTESIAN_POINT ( 'NONE',  ( -118.4694476160224781, 78.16069504672601909, -34.09644551253335010 ) ) ;
#3177=DIRECTION ( 'NONE',  ( 1.000000000000000000, 0.000000000000000000, 0.000000000000000000 ) ) ;
#3179=ADVANCED_FACE ( 'NONE', ( #2379 ), #10241, .F. ) ;
#3180=CARTESIAN_POINT ( 'NONE',  ( 96.25732604711784290, -115.9704170962574352, 9.968274243565256043 ) ) ;
#3189=CARTESIAN_POINT ( 'NONE',  ( 85.70335357680444588, -123.1056148428117183, 41.89337921544904475 ) ) ;
#3200=CARTESIAN_POINT ( 'NONE',  ( -107.4999999999999858, -118.5063289449133777, 0.000000000000000000 ) ) ;
#3205=CARTESIAN_POINT ( 'NONE',  ( -82.18957362175343917, -125.4791168306735329, 7.014959006335095282 ) ) ;
#3207=CARTESIAN_POINT ( 'NONE',  ( -91.89277925369268019, -118.5585056022070063, 47.62084010467887651 ) ) ;
#3209=CARTESIAN_POINT ( 'NONE',  ( -138.6697530361317945, 19.64131382463628839, 25.10535822172604270 ) ) ;
#3210=DIRECTION ( 'NONE',  ( 0.000000000000000000, 0.000000000000000000, 1.000000000000000000 ) ) ;
#3213=CARTESIAN_POINT ( 'NONE',  ( -132.4144148200023778, -86.21736781321662590, 39.45061808899835398 ) ) ;
#3226=EDGE_CURVE ( 'NONE', #10982, #16530, #10746, .T. ) ;
#3236=CARTESIAN_POINT ( 'NONE',  ( 134.6900874600792122, -73.16343714251466679, 31.49281596304311748 ) ) ;
#3238=CARTESIAN_POINT ( 'NONE',  ( 133.6841479863219888, -79.85751371701381629, 37.46951788548890505 ) ) ;
#3239=ORIENTED_EDGE ( 'NONE', *, *, #7352, .F. ) ;
#3250=ORIENTED_EDGE ( 'NONE', *, *, #17244, .F. ) ;
#3257=CARTESIAN_POINT ( 'NONE',  ( 128.9113527779074673, -76.70395394680461720, -7.603355451428101652 ) ) ;
#3259=EDGE_CURVE ( 'NONE', #3019, #3346, #2576, .T. ) ;
#3260=VERTEX_POINT ( 'NONE', #10434 ) ;
#3262=CARTESIAN_POINT ( 'NONE',  ( -110.0000000000000142, 275.0000000000000000, -67.49999999999997158 ) ) ;
#3265=DIRECTION ( 'NONE',  ( 1.000000000000000000, 0.000000000000000000, 0.000000000000000000 ) ) ;
#3266=DIRECTION ( 'NONE',  ( 0.4338837391175654479, -0.9009688679024155933, 0.000000000000000000 ) ) ;
#3270=ORIENTED_EDGE ( 'NONE', *, *, #13126, .F. ) ;
#3271=EDGE_CURVE ( 'NONE', #573, #15878, #18059, .T. ) ;
#3279=CYLINDRICAL_SURFACE ( 'NONE', #10565, 7.500000000000007105 ) ;
#3293=CARTESIAN_POINT ( 'NONE',  ( 82.18957362173902936, -125.4791168306830258, 32.98504099366878961 ) ) ;
#3295=FACE_OUTER_BOUND ( 'NONE', #6584, .T. ) ;
#3299=ORIENTED_EDGE ( 'NONE', *, *, #8527, .T. ) ;
#3303=ADVANCED_FACE ( 'NONE', ( #12276, #7677 ), #20161, .F. ) ;
#3304=DIRECTION ( 'NONE',  ( -0.9749279121818257288, 0.2225209339563050392, 0.000000000000000000 ) ) ;
#3311=CARTESIAN_POINT ( 'NONE',  ( -87.34436178610755519, -121.9468435064291612, 43.95302374537314449 ) ) ;
#3313=CARTESIAN_POINT ( 'NONE',  ( -119.1059459284890778, 73.60494313202988792, 38.81136714554597233 ) ) ;
#3318=CARTESIAN_POINT ( 'NONE',  ( -134.1895921339651920, -76.75826352743507641, 35.74347206174024905 ) ) ;
#3325=ORIENTED_EDGE ( 'NONE', *, *, #287, .F. ) ;
#3326=CARTESIAN_POINT ( 'NONE',  ( -144.8005054862046848, -14.35567093075204248, 8.862053436824973929 ) ) ;
#3332=CARTESIAN_POINT ( 'NONE',  ( 118.3534152657848608, 114.7431683447366595, 39.99999999999999289 ) ) ;
#3333=CARTESIAN_POINT ( 'NONE',  ( 98.69444885161529157, -132.3639744934813507, 34.75573401544776431 ) ) ;
#3336=CARTESIAN_POINT ( 'NONE',  ( 134.4925794577852685, -74.66012650511407855, 33.94317531104282892 ) ) ;
#3340=ORIENTED_EDGE ( 'NONE', *, *, #19364, .F. ) ;
#3346=VERTEX_POINT ( 'NONE', #1131 ) ;
#3348=CARTESIAN_POINT ( 'NONE',  ( -104.1558342746901218, -124.2522228486704421, 39.43806085740693135 ) ) ;
#3364=LINE ( 'NONE', #8060, #13066 ) ;
#3365=CARTESIAN_POINT ( 'NONE',  ( -75.16204133714633429, 118.1133591082685683, 1.232491660827630842 ) ) ;
#3372=CARTESIAN_POINT ( 'NONE',  ( 97.50000000000002842, -199.9999999999999716, 40.00000000000000000 ) ) ;
#3376=CIRCLE ( 'NONE', #17452, 7.500000000000020428 ) ;
#3377=ORIENTED_EDGE ( 'NONE', *, *, #4414, .F. ) ;
#3378=VECTOR ( 'NONE', #7689, 1000.000000000000000 ) ;
#3380=CYLINDRICAL_SURFACE ( 'NONE', #6596, 10.00000000000000888 ) ;
#3385=FACE_OUTER_BOUND ( 'NONE', #17886, .T. ) ;
#3390=DIRECTION ( 'NONE',  ( 1.000000000000000000, 0.000000000000000000, 0.000000000000000000 ) ) ;
#3392=CARTESIAN_POINT ( 'NONE',  ( 98.69108797088914287, -112.9688971639519934, 49.90760263315277712 ) ) ;
#3394=( BOUNDED_SURFACE ( )  B_SPLINE_SURFACE ( 3, 2, ( 
 ( #4296, #19743, #10139 ),
 ( #5440, #5636, #16489 ),
 ( #4091, #5740, #14934 ),
 ( #923, #7179, #11761 ),
 ( #16684, #18212, #16782 ),
 ( #19547, #7364, #13595 ),
 ( #2671, #727, #2566 ),
 ( #8800, #7075, #13393 ),
 ( #15042, #14746, #11667 ),
 ( #16391, #17928, #5540 ),
 ( #19840, #12057, #18320 ),
 ( #10523, #13289, #8506 ),
 ( #3900, #2370, #8604 ),
 ( #14839, #824, #16882 ),
 ( #10626, #14114, #102 ),
 ( #4607, #9098, #7462 ),
 ( #2973, #4713, #9311 ),
 ( #14011, #18631, #20152 ),
 ( #15661, #15237, #18836 ),
 ( #18424, #15340, #4399 ),
 ( #10733, #12369, #18521 ),
 ( #2872, #3180, #20051 ),
 ( #19944, #1332, #9203 ),
 ( #6353, #10830, #1540 ),
 ( #17089, #7564, #9413 ),
 ( #13806, #10938, #15554 ),
 ( #6256, #12572, #4501 ),
 ( #13702, #4821, #2 ),
 ( #6049, #12269, #16988 ),
 ( #7871, #18731, #15449 ),
 ( #3078, #1438, #1645 ),
 ( #7669, #1224, #11041 ) ),
 .UNSPECIFIED., .F., .F., .F. ) 
 B_SPLINE_SURFACE_WITH_KNOTS ( ( 4, 2, 2, 2, 2, 2, 2, 2, 2, 2, 2, 2, 2, 2, 2, 4 ),
 ( 3, 3 ),
 ( 0.02531008572351750585, 0.02976618726483498678, 0.03422228880615246771, 0.03645033957681120818, 0.03867839034746994864, 0.04313449188878743651, 0.04424851727411681368, 0.04536254265944618391, 0.04759059343010492438, 0.04981864420076366484, 0.05093266958609303507, 0.05204669497142240531, 0.05650279651273988624, 0.05761682189806925647, 0.05873084728339862670, 0.06095889805405736717 ),
 ( 0.000000000000000000, 1.000000000000000000 ),
 .UNSPECIFIED. ) 
 GEOMETRIC_REPRESENTATION_ITEM ( )  RATIONAL_B_SPLINE_SURFACE ( (
 ( 1.000000000000000000, 0.7071067811865475727, 1.000000000000000000),
 ( 1.000000000000000000, 0.6938858163890799791, 1.000000000000000000),
 ( 1.000000000000000000, 0.6806631602001719239, 1.000000000000000000),
 ( 1.000000000000000000, 0.6542661407885864699, 1.000000000000000000),
 ( 1.000000000000000000, 0.6410910482669636146, 1.000000000000000000),
 ( 1.000000000000000000, 0.6214215355382751715, 1.000000000000000000),
 ( 1.000000000000000000, 0.6148567640637033760, 1.000000000000000000),
 ( 1.000000000000000000, 0.6019746658714538734, 1.000000000000000000),
 ( 1.000000000000000000, 0.5956402134851142005, 1.000000000000000000),
 ( 1.000000000000000000, 0.5769855966611233677, 1.000000000000000000),
 ( 1.000000000000000000, 0.5650096313354644462, 1.000000000000000000),
 ( 1.000000000000000000, 0.5507648555196259510, 1.000000000000000000),
 ( 1.000000000000000000, 0.5479490128870576626, 1.000000000000000000),
 ( 1.000000000000000000, 0.5424554856653802659, 1.000000000000000000),
 ( 1.000000000000000000, 0.5397704441656565599, 1.000000000000000000),
 ( 1.000000000000000000, 0.5319045985432593326, 1.000000000000000000),
 ( 1.000000000000000000, 0.5269125948470546605, 1.000000000000000000),
 ( 1.000000000000000000, 0.5174644824775621599, 1.000000000000000000),
 ( 1.000000000000000000, 0.5130081457584921845, 1.000000000000000000),
 ( 1.000000000000000000, 0.5067628861632251791, 1.000000000000000000),
 ( 1.000000000000000000, 0.5047490957320777127, 1.000000000000000000),
 ( 1.000000000000000000, 0.5009263418717799787, 1.000000000000000000),
 ( 1.000000000000000000, 0.4991119735066631979, 1.000000000000000000),
 ( 1.000000000000000000, 0.4905251103114823819, 1.000000000000000000),
 ( 1.000000000000000000, 0.4851887169567591918, 1.000000000000000000),
 ( 1.000000000000000000, 0.4806071066594930219, 1.000000000000000000),
 ( 1.000000000000000000, 0.4797938356041033248, 1.000000000000000000),
 ( 1.000000000000000000, 0.4784048377102336214, 1.000000000000000000),
 ( 1.000000000000000000, 0.4778282137467559920, 1.000000000000000000),
 ( 1.000000000000000000, 0.4764456491719189501, 1.000000000000000000),
 ( 1.000000000000000000, 0.4759864261384231243, 1.000000000000000000),
 ( 1.000000000000000000, 0.4759858191164941243, 1.000000000000000000) ) ) 
 REPRESENTATION_ITEM ( '' )  SURFACE ( )  );
#3395=CARTESIAN_POINT ( 'NONE',  ( 15.91767397667354800, 164.0736214083062805, 39.99999999999999289 ) ) ;
#3396=CARTESIAN_POINT ( 'NONE',  ( -104.9326538737192323, 107.1912678330463677, 44.68324212414002261 ) ) ;
#3399=EDGE_LOOP ( 'NONE', ( #2716, #2111, #12208, #14666 ) ) ;
#3402=SHAPE_DEFINITION_REPRESENTATION ( #12918, #2084 ) ;
#3405=DIRECTION ( 'NONE',  ( 1.000000000000000000, 0.000000000000000000, 0.000000000000000000 ) ) ;
#3406=CARTESIAN_POINT ( 'NONE',  ( -121.0878816972190322, 88.53962377493060387, 43.43999758500223862 ) ) ;
#3410=CARTESIAN_POINT ( 'NONE',  ( 133.7387326730402322, -67.93012127445985016, 39.56577003862501840 ) ) ;
#3411=EDGE_CURVE ( 'NONE', #12392, #19032, #9419, .T. ) ;
#3412=EDGE_CURVE ( 'NONE', #13701, #5147, #9425, .T. ) ;
#3413=EDGE_CURVE ( 'NONE', #13701, #11033, #4863, .T. ) ;
#3414=CARTESIAN_POINT ( 'NONE',  ( -122.5787829483134601, 67.64166609452395562, 37.66536492912700851 ) ) ;
#3419=DIRECTION ( 'NONE',  ( 0.000000000000000000, 0.000000000000000000, -1.000000000000000000 ) ) ;
#3420=ORIENTED_EDGE ( 'NONE', *, *, #8373, .T. ) ;
#3424=VERTEX_POINT ( 'NONE', #11256 ) ;
#3428=DIRECTION ( 'NONE',  ( -1.000000000000000000, 0.000000000000000000, 0.000000000000000000 ) ) ;
#3433=CARTESIAN_POINT ( 'NONE',  ( 0.000000000000000000, 164.0736214083062805, 39.99999999999999289 ) ) ;
#3434=CARTESIAN_POINT ( 'NONE',  ( 98.02151343901461189, -133.2674925500989218, 33.21951988572780579 ) ) ;
#3435=AXIS2_PLACEMENT_3D ( 'NONE', #5026, #4929, #14326 ) ;
#3441=CARTESIAN_POINT ( 'NONE',  ( 134.5752827950141750, -74.04736996659980264, 33.19974057736502004 ) ) ;
#3447=VERTEX_POINT ( 'NONE', #418 ) ;
#3449=AXIS2_PLACEMENT_3D ( 'NONE', #8700, #11952, #5838 ) ;
#3451=CARTESIAN_POINT ( 'NONE',  ( -97.49999999999998579, -133.9542832461881687, 10.00000000000000178 ) ) ;
#3454=CARTESIAN_POINT ( 'NONE',  ( 131.9327818480801682, -71.37991627326495347, -3.783672495338017860 ) ) ;
#3456=ORIENTED_EDGE ( 'NONE', *, *, #3471, .T. ) ;
#3464=CIRCLE ( 'NONE', #14881, 10.00000000000000888 ) ;
#3465=CARTESIAN_POINT ( 'NONE',  ( 86.48208760716208587, -122.5631135004755805, 43.00921107642988517 ) ) ;
#3466=ORIENTED_EDGE ( 'NONE', *, *, #9851, .F. ) ;
#3469=ORIENTED_EDGE ( 'NONE', *, *, #15106, .F. ) ;
#3470=FACE_OUTER_BOUND ( 'NONE', #6199, .T. ) ;
#3471=EDGE_CURVE ( 'NONE', #10476, #12392, #14336, .T. ) ;
#3479=CARTESIAN_POINT ( 'NONE',  ( -110.0000000000000142, 275.0000000000000000, -75.00000000000000000 ) ) ;
#3483=LINE ( 'NONE', #1544, #16344 ) ;
#3485=VERTEX_POINT ( 'NONE', #18844 ) ;
#3487=DIRECTION ( 'NONE',  ( 0.000000000000000000, 0.000000000000000000, 1.000000000000000000 ) ) ;
#3498=EDGE_CURVE ( 'NONE', #14660, #18649, #16015, .T. ) ;
#3499=ORIENTED_EDGE ( 'NONE', *, *, #960, .F. ) ;
#3501=DIRECTION ( 'NONE',  ( 0.000000000000000000, 0.000000000000000000, 1.000000000000000000 ) ) ;
#3502=ORIENTED_EDGE ( 'NONE', *, *, #9739, .F. ) ;
#3507=( BOUNDED_CURVE ( )  B_SPLINE_CURVE ( 3, ( #10898, #12019, #165, #12639 ),
 .UNSPECIFIED., .F., .F. ) 
 B_SPLINE_CURVE_WITH_KNOTS ( ( 4, 4 ),
 ( 0.000000000000000000, 1.570796326794896558 ),
 .UNSPECIFIED. ) 
 CURVE ( )  GEOMETRIC_REPRESENTATION_ITEM ( )  RATIONAL_B_SPLINE_CURVE ( ( 1.000000000000000000, 0.8047378541243649375, 0.8047378541243649375, 1.000000000000000000 ) ) 
 REPRESENTATION_ITEM ( '' )  );
#3513=DIRECTION ( 'NONE',  ( -0.9009688679024155933, -0.4338837391175654479, 0.000000000000000000 ) ) ;
#3516=EDGE_LOOP ( 'NONE', ( #12107, #19283, #9218, #5758 ) ) ;
#3518=ORIENTED_EDGE ( 'NONE', *, *, #13615, .F. ) ;
#3522=ORIENTED_EDGE ( 'NONE', *, *, #5242, .F. ) ;
#3523=EDGE_CURVE ( 'NONE', #15303, #3260, #19297, .T. ) ;
#3525=VECTOR ( 'NONE', #17883, 1000.000000000000000 ) ;
#3531=CARTESIAN_POINT ( 'NONE',  ( -134.7652707650784407, -31.41120252075685215, -19.73219286542039441 ) ) ;
#3538=LINE ( 'NONE', #14382, #6471 ) ;
#3540=ORIENTED_EDGE ( 'NONE', *, *, #19008, .F. ) ;
#3544=ORIENTED_EDGE ( 'NONE', *, *, #12605, .T. ) ;
#3552=ADVANCED_FACE ( 'NONE', ( #6958 ), #16476, .F. ) ;
#3560=ORIENTED_EDGE ( 'NONE', *, *, #9396, .F. ) ;
#3561=FACE_OUTER_BOUND ( 'NONE', #18777, .T. ) ;
#3565=CARTESIAN_POINT ( 'NONE',  ( -141.6227766016837961, -18.73072656238141320, -9.999999999999985789 ) ) ;
#3566=FACE_OUTER_BOUND ( 'NONE', #14809, .T. ) ;
#3573=ORIENTED_EDGE ( 'NONE', *, *, #19996, .F. ) ;
#3579=ORIENTED_EDGE ( 'NONE', *, *, #20008, .T. ) ;
#3580=FACE_OUTER_BOUND ( 'NONE', #13716, .T. ) ;
#3583=CIRCLE ( 'NONE', #8162, 7.500000000000008882 ) ;
#3585=CARTESIAN_POINT ( 'NONE',  ( 106.5749805965075012, -120.1845445602442339, 7.623296525288700586E-17 ) ) ;
#3589=CARTESIAN_POINT ( 'NONE',  ( 4.189777606611760026E-13, -60.00000000000000000, -105.0000000000000142 ) ) ;
#3593=CARTESIAN_POINT ( 'NONE',  ( 99.34007343273268020, -112.3954413154693839, 39.16393061809239384 ) ) ;
#3596=CARTESIAN_POINT ( 'NONE',  ( -108.7690249705941596, 103.3081676305584864, 44.99999999999997868 ) ) ;
#3603=CARTESIAN_POINT ( 'NONE',  ( -149.6019236298159569, 11.14724313840852155, 10.74694859380678302 ) ) ;
#3607=CARTESIAN_POINT ( 'NONE',  ( -95.54911406155835607, -115.6381493485951069, -9.242025372095096003 ) ) ;
#3609=CIRCLE ( 'NONE', #15362, 7.500000000000001776 ) ;
#3613=FACE_BOUND ( 'NONE', #6450, .T. ) ;
#3614=EDGE_CURVE ( 'NONE', #14025, #17652, #14159, .T. ) ;
#3619=CARTESIAN_POINT ( 'NONE',  ( 0.000000000000000000, 0.000000000000000000, -100.0000000000000000 ) ) ;
#3623=CARTESIAN_POINT ( 'NONE',  ( -132.9093122671970093, 36.24889438955336374, -21.52074723781268872 ) ) ;
#3632=CARTESIAN_POINT ( 'NONE',  ( -135.7697856077824667, -31.23579568862577815, -16.57641459956559515 ) ) ;
#3633=CYLINDRICAL_SURFACE ( 'NONE', #614, 7.500000000000006217 ) ;
#3634=AXIS2_PLACEMENT_3D ( 'NONE', #9694, #17487, #19023 ) ;
#3640=DIRECTION ( 'NONE',  ( -0.000000000000000000, -0.000000000000000000, 1.000000000000000000 ) ) ;
#3641=EDGE_CURVE ( 'NONE', #6330, #6851, #3609, .T. ) ;
#3643=CARTESIAN_POINT ( 'NONE',  ( 130.9868171408399746, -91.88282611735537841, 40.00000000000000000 ) ) ;
#3645=ORIENTED_EDGE ( 'NONE', *, *, #8360, .F. ) ;
#3649=EDGE_CURVE ( 'NONE', #2972, #5912, #1208, .T. ) ;
#3659=DIRECTION ( 'NONE',  ( 1.613511099790691498E-16, -1.000000000000000000, 0.000000000000000000 ) ) ;
#3664=CARTESIAN_POINT ( 'NONE',  ( -134.5971911056698502, -73.88063391572673311, 32.93306624859282294 ) ) ;
#3665=CARTESIAN_POINT ( 'NONE',  ( -136.6495813276215472, -27.08701270267532024, -17.69344187970681403 ) ) ;
#3667=CARTESIAN_POINT ( 'NONE',  ( -76.10696272933056150, 117.5065231191640009, -3.774081802667871521 ) ) ;
#3670=LINE ( 'NONE', #11631, #12177 ) ;
#3673=VERTEX_POINT ( 'NONE', #4179 ) ;
#3677=CARTESIAN_POINT ( 'NONE',  ( -89.19226148815702970, -120.6070458769191589, 45.77850350706554394 ) ) ;
#3682=AXIS2_PLACEMENT_3D ( 'NONE', #14608, #13060, #5304 ) ;
#3688=CARTESIAN_POINT ( 'NONE',  ( 86.50547518363042343, -122.5441694604242429, -2.983597003230881839 ) ) ;
#3689=CARTESIAN_POINT ( 'NONE',  ( 100.0291087223604762, -111.7819692016171302, 39.61901476276965894 ) ) ;
#3690=EDGE_CURVE ( 'NONE', #5360, #5032, #15123, .T. ) ;
#3692=CARTESIAN_POINT ( 'NONE',  ( 71.18887634719571622, -147.8252249328912740, 39.99999999999999289 ) ) ;
#3693=CARTESIAN_POINT ( 'NONE',  ( -107.5112643209296976, 104.6166421110821432, 44.94337129641210993 ) ) ;
#3698=AXIS2_PLACEMENT_3D ( 'NONE', #7089, #4006, #5453 ) ;
#3701=CARTESIAN_POINT ( 'NONE',  ( -143.3909699111413545, 44.26766431025286153, 27.15461939389479085 ) ) ;
#3706=CARTESIAN_POINT ( 'NONE',  ( -84.44144489237834250, -123.9750712224044236, 0.1650835480906647224 ) ) ;
#3708=CARTESIAN_POINT ( 'NONE',  ( -138.4462077254157748, -20.96029677485602960, 25.40435766516374017 ) ) ;
#3711=( LENGTH_UNIT ( ) NAMED_UNIT ( * ) SI_UNIT ( .MILLI., .METRE. ) );
#3712=LINE ( 'NONE', #737, #15318 ) ;
#3714=ADVANCED_FACE ( 'NONE', ( #17075 ), #7446, .T. ) ;
#3721=VERTEX_POINT ( 'NONE', #12043 ) ;
#3724=CARTESIAN_POINT ( 'NONE',  ( -109.9999999999983515, 275.0000000000000000, 77.50000000000000000 ) ) ;
#3727=PLANE ( 'NONE',  #6176 ) ;
#3728=CYLINDRICAL_SURFACE ( 'NONE', #3772, 7.500000000000007105 ) ;
#3731=CARTESIAN_POINT ( 'NONE',  ( 102.6608643076873335, -126.6195776799898312, 38.76864583652064766 ) ) ;
#3733=EDGE_CURVE ( 'NONE', #7708, #7514, #7842, .T. ) ;
#3735=ORIENTED_EDGE ( 'NONE', *, *, #3742, .T. ) ;
#3740=ADVANCED_FACE ( 'NONE', ( #9083 ), #11128, .F. ) ;
#3742=EDGE_CURVE ( 'NONE', #4464, #14482, #17389, .T. ) ;
#3745=CARTESIAN_POINT ( 'NONE',  ( 156.4179374840099683, -52.02840013023883614, 39.99999999999999289 ) ) ;
#3747=AXIS2_PLACEMENT_3D ( 'NONE', #15837, #15785, #6483 ) ;
#3749=CARTESIAN_POINT ( 'NONE',  ( 79.05640494598117129, -127.4758205975433327, 49.99999999999999289 ) ) ;
#3753=AXIS2_PLACEMENT_3D ( 'NONE', #18055, #4031, #12092 ) ;
#3759=ORIENTED_EDGE ( 'NONE', *, *, #16980, .T. ) ;
#3767=ADVANCED_FACE ( 'NONE', ( #12867 ), #9698, .T. ) ;
#3772=AXIS2_PLACEMENT_3D ( 'NONE', #11787, #8830, #10070 ) ;
#3775=CARTESIAN_POINT ( 'NONE',  ( 134.1130761623740568, -69.50842595698583182, 49.99999999999999289 ) ) ;
#3776=AXIS2_PLACEMENT_3D ( 'NONE', #6481, #19070, #11273 ) ;
#3780=DIRECTION ( 'NONE',  ( 1.000000000000000000, 0.000000000000000000, 0.000000000000000000 ) ) ;
#3781=EDGE_CURVE ( 'NONE', #7108, #17239, #3364, .T. ) ;
#3785=ORIENTED_EDGE ( 'NONE', *, *, #15653, .T. ) ;
#3800=CARTESIAN_POINT ( 'NONE',  ( -84.96040761327874691, -123.6194689893696932, -0.7396600334858707271 ) ) ;
#3804=DIRECTION ( 'NONE',  ( 0.000000000000000000, -1.000000000000000000, -1.734723475976808080E-16 ) ) ;
#3805=DIRECTION ( 'NONE',  ( -0.000000000000000000, 1.000000000000000000, -0.000000000000000000 ) ) ;
#3806=VECTOR ( 'NONE', #20069, 1000.000000000000000 ) ;
#3807=DIRECTION ( 'NONE',  ( -1.000000000000000000, 0.000000000000000000, 0.000000000000000000 ) ) ;
#3809=DIRECTION ( 'NONE',  ( 0.000000000000000000, 0.000000000000000000, -1.000000000000000000 ) ) ;
#3812=AXIS2_PLACEMENT_3D ( 'NONE', #14386, #6616, #8035 ) ;
#3818=VERTEX_POINT ( 'NONE', #6240 ) ;
#3820=AXIS2_PLACEMENT_3D ( 'NONE', #5233, #8386, #11458 ) ;
#3821=CARTESIAN_POINT ( 'NONE',  ( -128.8937720816053627, -76.72575536401159013, -7.584633839317217685 ) ) ;
#3822=AXIS2_PLACEMENT_3D ( 'NONE', #13226, #17961, #5570 ) ;
#3825=ORIENTED_EDGE ( 'NONE', *, *, #3853, .F. ) ;
#3826=DIRECTION ( 'NONE',  ( 0.000000000000000000, 0.000000000000000000, 1.000000000000000000 ) ) ;
#3827=CARTESIAN_POINT ( 'NONE',  ( -131.7825524766324179, -71.64958008132045109, -3.998968123500318939 ) ) ;
#3828=CARTESIAN_POINT ( 'NONE',  ( 135.1060089022256818, -65.16414933467422088, 10.00000000000000888 ) ) ;
#3829=DIRECTION ( 'NONE',  ( -0.000000000000000000, -0.000000000000000000, -1.000000000000000000 ) ) ;
#3833=CIRCLE ( 'NONE', #6468, 150.0000000000000284 ) ;
#3839=ORIENTED_EDGE ( 'NONE', *, *, #12097, .F. ) ;
#3844=ORIENTED_EDGE ( 'NONE', *, *, #16132, .F. ) ;
#3845=CARTESIAN_POINT ( 'NONE',  ( -52.50000000000000000, -2.094888803305880013E-13, -100.0000000000000000 ) ) ;
#3846=LINE ( 'NONE', #2127, #8144 ) ;
#3847=AXIS2_PLACEMENT_3D ( 'NONE', #4446, #10677, #9151 ) ;
#3848=ORIENTED_EDGE ( 'NONE', *, *, #10883, .F. ) ;
#3849=CARTESIAN_POINT ( 'NONE',  ( 0.000000000000000000, 0.000000000000000000, 0.000000000000000000 ) ) ;
#3853=EDGE_CURVE ( 'NONE', #3346, #18071, #975, .T. ) ;
#3857=CARTESIAN_POINT ( 'NONE',  ( 0.000000000000000000, 60.00000000000000000, -105.0000000000000142 ) ) ;
#3875=VERTEX_POINT ( 'NONE', #2333 ) ;
#3877=CARTESIAN_POINT ( 'NONE',  ( 97.53506906366369833, -133.9085396777615244, 9.038951145123888864 ) ) ;
#3879=VECTOR ( 'NONE', #9498, 1000.000000000000000 ) ;
#3881=CARTESIAN_POINT ( 'NONE',  ( -71.18887634719365565, -147.8252249328922687, 39.99999999999999289 ) ) ;
#3882=VECTOR ( 'NONE', #9667, 1000.000000000000000 ) ;
#3883=ORIENTED_EDGE ( 'NONE', *, *, #14261, .F. ) ;
#3885=CARTESIAN_POINT ( 'NONE',  ( 97.50000000000002842, -199.9999999999999716, 30.00000000000000000 ) ) ;
#3887=CARTESIAN_POINT ( 'NONE',  ( 96.48429163929537822, -114.8598460512868513, -9.502487710326173342 ) ) ;
#3892=DIRECTION ( 'NONE',  ( 0.2225209339563050392, 0.9749279121818257288, 0.000000000000000000 ) ) ;
#3895=CIRCLE ( 'NONE', #5535, 150.0000000000000284 ) ;
#3900=CARTESIAN_POINT ( 'NONE',  ( 88.01533840461537750, -121.4634816193508300, -4.652272054116179945 ) ) ;
#3901=CARTESIAN_POINT ( 'NONE',  ( -89.41572940476631004, -120.4415366094358149, -5.961443665946996262 ) ) ;
#3902=CARTESIAN_POINT ( 'NONE',  ( -82.79607015190578068, -125.0792639210693267, 4.334714214550138500 ) ) ;
#3917=AXIS2_PLACEMENT_3D ( 'NONE', #13013, #3513, #11386 ) ;
#3919=AXIS2_PLACEMENT_3D ( 'NONE', #12195, #9027, #7592 ) ;
#3920=DIRECTION ( 'NONE',  ( 0.000000000000000000, 0.000000000000000000, -1.000000000000000000 ) ) ;
#3923=DIRECTION ( 'NONE',  ( 0.9009688679024221436, -0.4338837391175519032, 0.000000000000000000 ) ) ;
#3924=CARTESIAN_POINT ( 'NONE',  ( 85.53020504959901871, -140.9188050298377846, 39.99999999999999289 ) ) ;
#3926=DIRECTION ( 'NONE',  ( 0.9394263059140722794, -0.3427509529624095941, 0.000000000000000000 ) ) ;
#3927=CARTESIAN_POINT ( 'NONE',  ( -130.0420013710532601, -74.85033908744654241, 0.7491723846298292688 ) ) ;
#3928=CARTESIAN_POINT ( 'NONE',  ( 134.7188131035565277, -72.93593548749576883, 9.237785135033714567 ) ) ;
#3933=AXIS2_PLACEMENT_3D ( 'NONE', #10022, #16273, #16071 ) ;
#3937=DIRECTION ( 'NONE',  ( 0.000000000000000000, 0.000000000000000000, 1.000000000000000000 ) ) ;
#3944=CIRCLE ( 'NONE', #19631, 9.999999999999994671 ) ;
#3952=CIRCLE ( 'NONE', #7227, 150.0000000000000284 ) ;
#3953=CARTESIAN_POINT ( 'NONE',  ( -140.5398538968364051, -20.43888546547794505, -12.13436485393500419 ) ) ;
#3962=ORIENTED_EDGE ( 'NONE', *, *, #11279, .T. ) ;
#3963=DIRECTION ( 'NONE',  ( -0.000000000000000000, -0.000000000000000000, -1.000000000000000000 ) ) ;
#3970=CARTESIAN_POINT ( 'NONE',  ( -134.2425157119612891, -66.92593549375912687, 37.65294690872419636 ) ) ;
#3971=LINE ( 'NONE', #3775, #1266 ) ;
#3977=CARTESIAN_POINT ( 'NONE',  ( 84.48076729319797096, -123.9477347680102497, 0.1101890534364035890 ) ) ;
#3978=CYLINDRICAL_SURFACE ( 'NONE', #9888, 7.500000000000006217 ) ;
#3979=ORIENTED_EDGE ( 'NONE', *, *, #18502, .F. ) ;
#3981=DIRECTION ( 'NONE',  ( 1.000000000000000000, 0.000000000000000000, 0.000000000000000000 ) ) ;
#3993=CARTESIAN_POINT ( 'NONE',  ( -86.68385341649090492, -122.4206889339686484, -3.257968381067569474 ) ) ;
#3997=CARTESIAN_POINT ( 'NONE',  ( 167.4599531637113330, -36.50981547336952104, 49.99999999999999289 ) ) ;
#4000=LINE ( 'NONE', #7082, #331 ) ;
#4006=DIRECTION ( 'NONE',  ( 0.3427509529624096496, 0.9394263059140723904, 0.000000000000000000 ) ) ;
#4010=EDGE_LOOP ( 'NONE', ( #768, #5381, #14928, #5925 ) ) ;
#4013=DIRECTION ( 'NONE',  ( 0.000000000000000000, 0.000000000000000000, 1.000000000000000000 ) ) ;
#4015=ADVANCED_FACE ( 'NONE', ( #3566 ), #9799, .F. ) ;
#4016=EDGE_CURVE ( 'NONE', #5755, #13097, #6935, .T. ) ;
#4017=CARTESIAN_POINT ( 'NONE',  ( 134.7188131032333445, -72.93593548660993520, 30.00000000000000000 ) ) ;
#4023=DIRECTION ( 'NONE',  ( 0.000000000000000000, 0.000000000000000000, 1.000000000000000000 ) ) ;
#4026=CARTESIAN_POINT ( 'NONE',  ( -124.9958490024057198, -82.94424249022438289, -0.9643169688603490108 ) ) ;
#4028=AXIS2_PLACEMENT_3D ( 'NONE', #17970, #3937, #16432 ) ;
#4029=DIRECTION ( 'NONE',  ( -1.000000000000000000, 0.000000000000000000, 0.000000000000000000 ) ) ;
#4031=DIRECTION ( 'NONE',  ( -0.000000000000000000, -0.000000000000000000, -1.000000000000000000 ) ) ;
#4032=ORIENTED_EDGE ( 'NONE', *, *, #9117, .F. ) ;
#4033=EDGE_CURVE ( 'NONE', #7965, #14351, #3117, .T. ) ;
#4041=DIRECTION ( 'NONE',  ( 1.224646799147353207E-16, 1.000000000000000000, -0.000000000000000000 ) ) ;
#4045=ORIENTED_EDGE ( 'NONE', *, *, #16863, .F. ) ;
#4046=CARTESIAN_POINT ( 'NONE',  ( -67.50000000000000000, -2.085703952312275003E-13, -105.0000000000000142 ) ) ;
#4047=CARTESIAN_POINT ( 'NONE',  ( -110.0000000000000142, 265.0000000000000000, 5.000000000000000888 ) ) ;
#4048=EDGE_CURVE ( 'NONE', #19359, #12474, #9036, .T. ) ;
#4049=ORIENTED_EDGE ( 'NONE', *, *, #18884, .T. ) ;
#4050=CARTESIAN_POINT ( 'NONE',  ( 181.0783081749256951, -199.9999999999999716, 40.00000000000000000 ) ) ;
#4057=DIRECTION ( 'NONE',  ( 0.000000000000000000, 0.000000000000000000, 1.000000000000000000 ) ) ;
#4060=ORIENTED_EDGE ( 'NONE', *, *, #12257, .T. ) ;
#4062=VERTEX_POINT ( 'NONE', #1578 ) ;
#4065=CARTESIAN_POINT ( 'NONE',  ( -84.01517049618257715, -124.2637720100346002, 38.96058320792450047 ) ) ;
#4066=LINE ( 'NONE', #18189, #14871 ) ;
#4067=DIRECTION ( 'NONE',  ( 0.000000000000000000, 0.000000000000000000, 1.000000000000000000 ) ) ;
#4070=DIRECTION ( 'NONE',  ( -0.7406645559057083439, 0.6718749999999998890, 0.000000000000000000 ) ) ;
#4073=DIRECTION ( 'NONE',  ( -1.000000000000000000, 0.000000000000000000, 0.000000000000000000 ) ) ;
#4076=CARTESIAN_POINT ( 'NONE',  ( 84.01517049618261979, -124.2637720100345717, 1.039416792075506635 ) ) ;
#4085=ORIENTED_EDGE ( 'NONE', *, *, #388, .T. ) ;
#4091=CARTESIAN_POINT ( 'NONE',  ( 98.69083902877214598, -112.9691409624333573, -9.907675691193132295 ) ) ;
#4093=EDGE_CURVE ( 'NONE', #301, #18014, #1683, .T. ) ;
#4099=SHAPE_REPRESENTATION_RELATIONSHIP ( 'NONE' , 'NONE' ,  #2084, #13837 ) ;
#4102=CIRCLE ( 'NONE', #13902, 10.00000000000000888 ) ;
#4104=ADVANCED_FACE ( 'NONE', ( #13740 ), #10777, .F. ) ;
#4106=CYLINDRICAL_SURFACE ( 'NONE', #3698, 9.999999999999994671 ) ;
#4107=ADVANCED_FACE ( 'NONE', ( #19982 ), #13844, .T. ) ;
#4120=CARTESIAN_POINT ( 'NONE',  ( -98.69083902876617742, -112.9691409624384733, 49.90767569119055480 ) ) ;
#4121=DIRECTION ( 'NONE',  ( 0.000000000000000000, 0.000000000000000000, -1.000000000000000000 ) ) ;
#4123=DIRECTION ( 'NONE',  ( 0.3427509529624101492, -0.9394263059140720573, -0.000000000000000000 ) ) ;
#4124=CARTESIAN_POINT ( 'NONE',  ( -132.2990932590211628, -86.73761849284356629, 0.4401276754358985355 ) ) ;
#4126=CARTESIAN_POINT ( 'NONE',  ( 134.5311723999374465, -74.37598470587731470, 6.383662503987586945 ) ) ;
#4137=ADVANCED_FACE ( 'NONE', ( #6395 ), #7601, .T. ) ;
#4140=AXIS2_PLACEMENT_3D ( 'NONE', #2879, #13604, #9106 ) ;
#4142=EDGE_CURVE ( 'NONE', #3424, #15773, #16334, .T. ) ;
#4148=ORIENTED_EDGE ( 'NONE', *, *, #6993, .F. ) ;
#4151=CARTESIAN_POINT ( 'NONE',  ( -133.1916981995337892, -82.53555109165357351, 1.486209767972074047 ) ) ;
#4153=CIRCLE ( 'NONE', #10688, 7.500000000000006217 ) ;
#4169=LINE ( 'NONE', #16852, #127 ) ;
#4172=CYLINDRICAL_SURFACE ( 'NONE', #11904, 7.500000000000001776 ) ;
#4174=CARTESIAN_POINT ( 'NONE',  ( -125.6254798881099362, -81.96796683352710033, 49.52966944193529741 ) ) ;
#4179=CARTESIAN_POINT ( 'NONE',  ( -148.9554720520392834, -17.67108784863416560, 39.99999999999999289 ) ) ;
#4182=VERTEX_POINT ( 'NONE', #9556 ) ;
#4187=ORIENTED_EDGE ( 'NONE', *, *, #9409, .T. ) ;
#4192=DIRECTION ( 'NONE',  ( 1.000000000000000000, 0.000000000000000000, 0.000000000000000000 ) ) ;
#4196=CARTESIAN_POINT ( 'NONE',  ( 118.3534152657848608, 114.7431683447366595, 39.99999999999999289 ) ) ;
#4206=EDGE_LOOP ( 'NONE', ( #3848, #19881, #18876, #2939, #7895 ) ) ;
#4217=CARTESIAN_POINT ( 'NONE',  ( 134.0425641885189805, -77.70550467234687630, 3.648054164520854847 ) ) ;
#4221=PLANE ( 'NONE',  #7792 ) ;
#4229=CARTESIAN_POINT ( 'NONE',  ( -134.2531151303053036, -76.34772591580372136, 4.523541615885667611 ) ) ;
#4231=CARTESIAN_POINT ( 'NONE',  ( -174.2942412179009466, -197.9050378206823098, 1.885337547879245069E-14 ) ) ;
#4233=CARTESIAN_POINT ( 'NONE',  ( 97.50000000000002842, -189.9999999999999716, 30.00000000000000000 ) ) ;
#4236=ADVANCED_FACE ( 'NONE', ( #16005 ), #6495, .F. ) ;
#4244=EDGE_CURVE ( 'NONE', #11053, #269, #2055, .T. ) ;
#4250=VECTOR ( 'NONE', #4592, 1000.000000000000000 ) ;
#4277=EDGE_CURVE ( 'NONE', #2619, #6330, #10245, .T. ) ;
#4284=CARTESIAN_POINT ( 'NONE',  ( -79.51226524016391295, 115.2339015673091041, 22.26257494144193672 ) ) ;
#4286=DIRECTION ( 'NONE',  ( 0.9009688679024221436, -0.4338837391175519032, 0.000000000000000000 ) ) ;
#4296=CARTESIAN_POINT ( 'NONE',  ( 100.7812500000000284, -111.0996833858562667, -10.00000000000000355 ) ) ;
#4313=ORIENTED_EDGE ( 'NONE', *, *, #12979, .T. ) ;
#4315=CARTESIAN_POINT ( 'NONE',  ( 132.6218665116185207, -85.29503539049812844, 0.7312914155056859933 ) ) ;
#4323=CARTESIAN_POINT ( 'NONE',  ( -133.0788080491334142, -69.33756331725891187, 7.374420170790281226 ) ) ;
#4324=CARTESIAN_POINT ( 'NONE',  ( 133.8587666923837105, -78.85012038918880251, 2.995270696459912063 ) ) ;
#4326=AXIS2_PLACEMENT_3D ( 'NONE', #17810, #16074, #3780 ) ;
#4329=CARTESIAN_POINT ( 'NONE',  ( -134.6385828715869479, -73.56429320929808569, 32.40089326748427112 ) ) ;
#4331=CARTESIAN_POINT ( 'NONE',  ( -110.0000000000000142, 275.0000000000000000, 5.000000000000000888 ) ) ;
#4337=CIRCLE ( 'NONE', #2384, 15.91767397667355510 ) ;
#4340=CARTESIAN_POINT ( 'NONE',  ( -140.6610699913552764, -20.33010010770880172, 21.89506024342324153 ) ) ;
#4341=CARTESIAN_POINT ( 'NONE',  ( -110.0000000000000142, 165.0000000000000000, 44.99999999999998579 ) ) ;
#4343=ORIENTED_EDGE ( 'NONE', *, *, #18502, .T. ) ;
#4345=DIRECTION ( 'NONE',  ( 0.8186676071302501079, 0.5742676632334704490, -6.938893903907233308E-16 ) ) ;
#4346=DIRECTION ( 'NONE',  ( 0.000000000000000000, 0.000000000000000000, 1.000000000000000000 ) ) ;
#4351=CARTESIAN_POINT ( 'NONE',  ( -134.7088667886416999, -73.01552020433989298, 9.022702824945225686 ) ) ;
#4355=CARTESIAN_POINT ( 'NONE',  ( 125.9311142016122034, -81.50627728739362965, 49.44517127269371315 ) ) ;
#4361=EDGE_LOOP ( 'NONE', ( #10250, #8749 ) ) ;
#4363=ORIENTED_EDGE ( 'NONE', *, *, #9279, .T. ) ;
#4372=VERTEX_POINT ( 'NONE', #10154 ) ;
#4384=CARTESIAN_POINT ( 'NONE',  ( -108.9451041445662014, 87.93000889276720500, 39.98824025397081527 ) ) ;
#4389=EDGE_CURVE ( 'NONE', #11232, #2972, #9240, .T. ) ;
#4390=ADVANCED_FACE ( 'NONE', ( #16310 ), #4106, .T. ) ;
#4393=CARTESIAN_POINT ( 'NONE',  ( -97.26553299953361886, -115.5756973141631931, 29.67990786120111224 ) ) ;
#4394=AXIS2_PLACEMENT_3D ( 'NONE', #7878, #3082, #12169 ) ;
#4399=CARTESIAN_POINT ( 'NONE',  ( 98.87769906228768946, -132.1136377592460747, 4.931739911029251466 ) ) ;
#4402=EDGE_CURVE ( 'NONE', #10476, #796, #13803, .T. ) ;
#4403=CARTESIAN_POINT ( 'NONE',  ( -137.9787687278481201, -24.44938394645547675, -11.76118810246814306 ) ) ;
#4405=DIRECTION ( 'NONE',  ( 1.000000000000000000, 0.000000000000000000, -0.000000000000000000 ) ) ;
#4410=CARTESIAN_POINT ( 'NONE',  ( 97.37676942331995633, -115.5300780475686935, 29.69431357006366312 ) ) ;
#4414=EDGE_CURVE ( 'NONE', #18388, #11005, #4337, .T. ) ;
#4416=VERTEX_POINT ( 'NONE', #9216 ) ;
#4421=EDGE_LOOP ( 'NONE', ( #11608, #2096, #19039, #5820, #10199 ) ) ;
#4433=CARTESIAN_POINT ( 'NONE',  ( 134.4267602304456091, -75.13220794378300127, 5.582054549155156309 ) ) ;
#4436=CARTESIAN_POINT ( 'NONE',  ( -134.7188131032333445, -72.93593548660989256, 30.00000000000000000 ) ) ;
#4437=CARTESIAN_POINT ( 'NONE',  ( -132.7564094051443249, -84.67399327756427851, 39.12603430846659336 ) ) ;
#4438=ORIENTED_EDGE ( 'NONE', *, *, #17387, .T. ) ;
#4443=ORIENTED_EDGE ( 'NONE', *, *, #398, .T. ) ;
#4446=CARTESIAN_POINT ( 'NONE',  ( -110.0000000000000142, 0.000000000000000000, 5.000000000000000888 ) ) ;
#4447=VERTEX_POINT ( 'NONE', #18648 ) ;
#4448=CARTESIAN_POINT ( 'NONE',  ( -139.8142396999972163, 1.712230611238718486E-14, -13.33333333333329307 ) ) ;
#4455=CARTESIAN_POINT ( 'NONE',  ( 140.0000000000000000, 0.000000000000000000, -9.999999999999987566 ) ) ;
#4458=CARTESIAN_POINT ( 'NONE',  ( 128.7737027234268510, -76.92703321535536531, 47.68818876599771528 ) ) ;
#4460=ORIENTED_EDGE ( 'NONE', *, *, #15009, .F. ) ;
#4461=CIRCLE ( 'NONE', #3820, 150.0000000000000284 ) ;
#4464=VERTEX_POINT ( 'NONE', #15569 ) ;
#4471=DIRECTION ( 'NONE',  ( -0.9009688679024212554, 0.4338837391175534575, 0.000000000000000000 ) ) ;
#4474=LINE ( 'NONE', #6124, #10002 ) ;
#4478=EDGE_CURVE ( 'NONE', #5530, #5045, #11832, .T. ) ;
#4479=VECTOR ( 'NONE', #17853, 1000.000000000000000 ) ;
#4482=EDGE_CURVE ( 'NONE', #14025, #4062, #15115, .T. ) ;
#4486=CARTESIAN_POINT ( 'NONE',  ( -133.9068821628478929, -78.54443609883628596, 36.82575673622204704 ) ) ;
#4488=EDGE_LOOP ( 'NONE', ( #5982, #886 ) ) ;
#4493=EDGE_LOOP ( 'NONE', ( #8545, #12749, #13580, #10268 ) ) ;
#4495=CARTESIAN_POINT ( 'NONE',  ( -97.52076053070028649, -133.9271890290945350, 30.74418362133967619 ) ) ;
#4496=AXIS2_PLACEMENT_3D ( 'NONE', #11200, #14279, #13039 ) ;
#4498=CARTESIAN_POINT ( 'NONE',  ( -123.9152654547992825, 71.52026188392119366, -32.55817170788386505 ) ) ;
#4501=CARTESIAN_POINT ( 'NONE',  ( 97.67167802517904818, -133.7293924297389935, 8.145492481267311291 ) ) ;
#4503=EDGE_CURVE ( 'NONE', #17764, #8819, #6167, .T. ) ;
#4510=FACE_OUTER_BOUND ( 'NONE', #5505, .T. ) ;
#4512=CARTESIAN_POINT ( 'NONE',  ( 97.50000000000001421, -115.4778303846449887, 30.00000000000000000 ) ) ;
#4524=CARTESIAN_POINT ( 'NONE',  ( -99.98080768883880864, -130.5801677638305023, 3.398603488195621303 ) ) ;
#4525=CIRCLE ( 'NONE', #6156, 150.0000000000000284 ) ;
#4526=CARTESIAN_POINT ( 'NONE',  ( -170.2125097089225960, -199.3942630591408260, 40.00000000000000000 ) ) ;
#4527=ORIENTED_EDGE ( 'NONE', *, *, #7720, .F. ) ;
#4528=CARTESIAN_POINT ( 'NONE',  ( -107.4999999999999858, -118.5063289449133777, 0.000000000000000000 ) ) ;
#4531=CARTESIAN_POINT ( 'NONE',  ( -93.96728894855066017, -116.9213660262001611, 48.64206144702517065 ) ) ;
#4537=CARTESIAN_POINT ( 'NONE',  ( -134.1862644405548508, -67.03876562297297426, 2.113649378061198458 ) ) ;
#4538=CARTESIAN_POINT ( 'NONE',  ( 133.2581445365297839, -82.18041427990311831, 1.616105938608680903 ) ) ;
#4539=CARTESIAN_POINT ( 'NONE',  ( 71.18887634719571622, -147.8252249328912740, 39.99999999999999289 ) ) ;
#4542=CARTESIAN_POINT ( 'NONE',  ( -125.5830613944035861, -82.05591916722895007, 41.02171822117688293 ) ) ;
#4543=AXIS2_PLACEMENT_3D ( 'NONE', #10811, #20229, #9181 ) ;
#4551=VERTEX_POINT ( 'NONE', #7784 ) ;
#4552=AXIS2_PLACEMENT_3D ( 'NONE', #1798, #7620, #12318 ) ;
#4553=CARTESIAN_POINT ( 'NONE',  ( -143.6483359526046968, -15.80165949809716075, 14.64470287550839522 ) ) ;
#4560=EDGE_LOOP ( 'NONE', ( #19741, #11591, #8740, #15213 ) ) ;
#4561=CARTESIAN_POINT ( 'NONE',  ( -84.36291539053216582, 110.0674672679312636, -18.84752057685613025 ) ) ;
#4566=CARTESIAN_POINT ( 'NONE',  ( 134.1862644405590856, -67.03876562296453301, 37.88635062194084924 ) ) ;
#4579=DIRECTION ( 'NONE',  ( 0.000000000000000000, 0.000000000000000000, 1.000000000000000000 ) ) ;
#4581=FACE_OUTER_BOUND ( 'NONE', #4010, .T. ) ;
#4585=DIRECTION ( 'NONE',  ( 0.000000000000000000, 0.000000000000000000, 1.000000000000000000 ) ) ;
#4592=DIRECTION ( 'NONE',  ( 0.9749279121818227312, 0.2225209339563182231, -0.000000000000000000 ) ) ;
#4593=LINE ( 'NONE', #18982, #19373 ) ;
#4595=DIRECTION ( 'NONE',  ( -1.000000000000000000, 0.000000000000000000, 0.000000000000000000 ) ) ;
#4603=EDGE_CURVE ( 'NONE', #10224, #5218, #10959, .T. ) ;
#4604=CARTESIAN_POINT ( 'NONE',  ( -116.4638672662962193, 80.60801470281606385, -34.47751397565569675 ) ) ;
#4605=DIRECTION ( 'NONE',  ( -1.000000000000000000, -3.320906611023727849E-16, 0.000000000000000000 ) ) ;
#4607=CARTESIAN_POINT ( 'NONE',  ( 86.69744916219704578, -122.4084679129025659, -3.219996018902601342 ) ) ;
#4613=FACE_BOUND ( 'NONE', #11525, .T. ) ;
#4618=CARTESIAN_POINT ( 'NONE',  ( 97.83472796452251430, -133.5146506974446652, 32.57231315946213357 ) ) ;
#4623=ORIENTED_EDGE ( 'NONE', *, *, #6993, .T. ) ;
#4626=EDGE_CURVE ( 'NONE', #18093, #17792, #13468, .T. ) ;
#4631=DIRECTION ( 'NONE',  ( 0.000000000000000000, 0.000000000000000000, 1.000000000000000000 ) ) ;
#4637=CARTESIAN_POINT ( 'NONE',  ( 124.4460166144179425, -83.75677717049840965, 49.87899788059623063 ) ) ;
#4638=CARTESIAN_POINT ( 'NONE',  ( -95.64660831657310780, -115.7365562161970587, 34.13915741641437762 ) ) ;
#4639=DIRECTION ( 'NONE',  ( 0.000000000000000000, 0.000000000000000000, 1.000000000000000000 ) ) ;
#4640=LINE ( 'NONE', #9713, #7465 ) ;
#4644=CARTESIAN_POINT ( 'NONE',  ( 123.6072353705854141, -84.98956761793972703, -9.999999999628117919 ) ) ;
#4647=CARTESIAN_POINT ( 'NONE',  ( -129.2715203052800916, -76.16417937454788500, 39.91219297793836063 ) ) ;
#4650=CIRCLE ( 'NONE', #9558, 7.500000000000012434 ) ;
#4652=EDGE_CURVE ( 'NONE', #13930, #3067, #6865, .T. ) ;
#4655=ADVANCED_FACE ( 'NONE', ( #622, #2558 ), #2458, .T. ) ;
#4658=CARTESIAN_POINT ( 'NONE',  ( -144.8974563261294861, -14.24083055819320087, 7.862900427932681069 ) ) ;
#4661=LINE ( 'NONE', #9662, #11043 ) ;
#4664=CARTESIAN_POINT ( 'NONE',  ( -79.05640494597939494, -127.4758205975444412, 39.99999999999999289 ) ) ;
#4668=B_SPLINE_CURVE_WITH_KNOTS ( 'NONE', 3,
 ( #6236, #12450, #18711, #1313, #4695, #4799, #20029, #3162, #9393, #15639, #1624, #1199, #82, #14094, #12554, #11022, #7442, #17383, #584, #6832, #4906, #14307, #9792, #17781, #17687, #13056, #1928, #9497 ),
 .UNSPECIFIED., .F., .F.,
 ( 4, 2, 2, 2, 2, 2, 2, 2, 2, 2, 2, 2, 2, 4 ),
 ( 2.166383432107200764E-07, 0.004056336319593734953, 0.008112456000844259218, 0.01014051584146950270, 0.01216857568209474792, 0.01622469536334526785, 0.02028081504459578258, 0.02433693472584630077, 0.03244917408834733369, 0.04056141345084836314, 0.04461753313209888827, 0.04867365281334941340, 0.05678589217585046367, 0.06489813153835151394 ),
 .UNSPECIFIED. ) ;
#4674=CARTESIAN_POINT ( 'NONE',  ( 132.5536774537058591, -70.21235394457261236, 42.53698427006028027 ) ) ;
#4677=ORIENTED_EDGE ( 'NONE', *, *, #17006, .F. ) ;
#4678=AXIS2_PLACEMENT_3D ( 'NONE', #14852, #19657, #6891 ) ;
#4680=VERTEX_POINT ( 'NONE', #11844 ) ;
#4690=B_SPLINE_CURVE_WITH_KNOTS ( 'NONE', 3,
 ( #12962, #14205, #590, #9503, #12767, #14510, #16150, #2137, #496, #17287, #9801, #14609, #17490, #189, #6444, #6740, #3465, #18824, #6837, #11231, #19223, #12665, #5210, #11439, #9699, #17694, #9601, #19026, #15948, #8167 ),
 .UNSPECIFIED., .F., .F.,
 ( 4, 2, 2, 2, 2, 2, 2, 2, 2, 2, 2, 2, 2, 2, 4 ),
 ( 0.000000000000000000, 0.002170930610089417522, 0.004341861220178835044, 0.008683722440357699579, 0.01085465305044713488, 0.01302558366053657019, 0.01519651427062600549, 0.01736744488071544079, 0.02170930610089430099, 0.02388023671098372935, 0.02605116732107315772, 0.02822209793116258608, 0.02930756323620730200, 0.03039302854125202139, 0.03473488976143086771 ),
 .UNSPECIFIED. ) ;
#4695=CARTESIAN_POINT ( 'NONE',  ( -75.78723542615585984, 128.9816322699055888, -15.76009018109207993 ) ) ;
#4699=CIRCLE ( 'NONE', #12523, 9.999999999999996447 ) ;
#4700=DIRECTION ( 'NONE',  ( 0.000000000000000000, 0.000000000000000000, 1.000000000000000000 ) ) ;
#4701=CARTESIAN_POINT ( 'NONE',  ( -88.41331621464559021, 108.5600746955366844, 32.58608401720460535 ) ) ;
#4706=ORIENTED_EDGE ( 'NONE', *, *, #13979, .F. ) ;
#4709=CARTESIAN_POINT ( 'NONE',  ( -166.7850001792984926, -190.0000000000000284, 0.000000000000000000 ) ) ;
#4710=DIRECTION ( 'NONE',  ( 1.000000000000000000, 0.000000000000000000, 0.000000000000000000 ) ) ;
#4711=ORIENTED_EDGE ( 'NONE', *, *, #8554, .T. ) ;
#4713=CARTESIAN_POINT ( 'NONE',  ( 95.59344839195293275, -116.1516065318577091, 8.743803915443725927 ) ) ;
#4717=EDGE_LOOP ( 'NONE', ( #3047, #7884, #5946, #8234 ) ) ;
#4719=CARTESIAN_POINT ( 'NONE',  ( -97.49999999999997158, -190.0000000000000000, 40.00000000000000000 ) ) ;
#4720=DIRECTION ( 'NONE',  ( 0.000000000000000000, 0.000000000000000000, 1.000000000000000000 ) ) ;
#4721=DIRECTION ( 'NONE',  ( -0.000000000000000000, -1.000000000000000000, -0.000000000000000000 ) ) ;
#4722=CARTESIAN_POINT ( 'NONE',  ( 82.95463716431549983, -124.9741831325246579, 36.20982395953856070 ) ) ;
#4726=ORIENTED_EDGE ( 'NONE', *, *, #13573, .T. ) ;
#4728=B_SPLINE_CURVE_WITH_KNOTS ( 'NONE', 3,
 ( #19799, #5694, #7319, #19697, #12116, #2827, #13657, #4151, #13757, #18271, #10378, #18374, #11911, #15298, #18169, #10190, #6002, #14891, #16641, #16447, #11808, #4351, #2626, #8853 ),
 .UNSPECIFIED., .F., .F.,
 ( 4, 2, 2, 2, 2, 2, 2, 2, 2, 2, 2, 4 ),
 ( 0.000000000000000000, 0.002919511036912186049, 0.005839022073824372099, 0.008758533110736557714, 0.01167804414764874420, 0.01313779966610484351, 0.01459755518456094629, 0.01751706622147310849, 0.01897682173992918872, 0.02043657725838527242, 0.02189633277684135612, 0.02335608829529743635 ),
 .UNSPECIFIED. ) ;
#4735=DIRECTION ( 'NONE',  ( 0.000000000000000000, 0.000000000000000000, 1.000000000000000000 ) ) ;
#4742=CARTESIAN_POINT ( 'NONE',  ( 134.9931224044436817, -65.39776452395021522, 32.90319768524037158 ) ) ;
#4743=CARTESIAN_POINT ( 'NONE',  ( -98.87769906228751893, -132.1136377592408735, 35.06826008897053271 ) ) ;
#4745=LINE ( 'NONE', #15693, #8691 ) ;
#4746=CARTESIAN_POINT ( 'NONE',  ( -139.6619321461413961, 9.919133126256308941, 23.58131293488760249 ) ) ;
#4752=CARTESIAN_POINT ( 'NONE',  ( -130.0495322079418372, -74.74954793754226046, 46.42469753870267368 ) ) ;
#4759=ORIENTED_EDGE ( 'NONE', *, *, #548, .T. ) ;
#4762=CARTESIAN_POINT ( 'NONE',  ( -143.5145034128292707, -15.97856208114589016, 15.09934064724655833 ) ) ;
#4768=FACE_OUTER_BOUND ( 'NONE', #13643, .T. ) ;
#4771=DIRECTION ( 'NONE',  ( 0.000000000000000000, 0.000000000000000000, 1.000000000000000000 ) ) ;
#4778=CARTESIAN_POINT ( 'NONE',  ( 134.5315346870376629, -74.37329574991311176, 33.61297800067708152 ) ) ;
#4790=CARTESIAN_POINT ( 'NONE',  ( -98.70372244599820988, -132.3513910121202741, 34.77299687110840409 ) ) ;
#4794=CARTESIAN_POINT ( 'NONE',  ( -166.7850001792984926, -190.0000000000000284, 40.00000000000000000 ) ) ;
#4796=VECTOR ( 'NONE', #18764, 1000.000000000000000 ) ;
#4799=CARTESIAN_POINT ( 'NONE',  ( -76.78599263319790680, 128.0787319494822896, -17.29805744153746616 ) ) ;
#4800=DIRECTION ( 'NONE',  ( -0.3427509529624096496, -0.9394263059140723904, 0.000000000000000000 ) ) ;
#4801=ADVANCED_FACE ( 'NONE', ( #2964 ), #13690, .T. ) ;
#4805=FACE_OUTER_BOUND ( 'NONE', #1687, .T. ) ;
#4821=CARTESIAN_POINT ( 'NONE',  ( 97.34896704141638679, -115.5410409672066692, 10.27529861476682527 ) ) ;
#4825=VERTEX_POINT ( 'NONE', #17346 ) ;
#4829=CARTESIAN_POINT ( 'NONE',  ( 97.50000000000001421, -133.9542832455803989, 30.75506667725924714 ) ) ;
#4832=( BOUNDED_CURVE ( )  B_SPLINE_CURVE ( 3, ( #6109, #1179, #12120, #15513 ),
 .UNSPECIFIED., .F., .F. ) 
 B_SPLINE_CURVE_WITH_KNOTS ( ( 4, 4 ),
 ( 1.920639998745670596, 3.141592653589794004 ),
 .UNSPECIFIED. ) 
 CURVE ( )  GEOMETRIC_REPRESENTATION_ITEM ( )  RATIONAL_B_SPLINE_CURVE ( ( 1.000000000000000000, 0.8795833682608492632, 0.8795833682608492632, 1.000000000000000000 ) ) 
 REPRESENTATION_ITEM ( '' )  );
#4835=CARTESIAN_POINT ( 'NONE',  ( -82.03494826539123608, 125.5818021290787669, 33.61186608239164997 ) ) ;
#4839=ORIENTED_EDGE ( 'NONE', *, *, #13152, .F. ) ;
#4846=CARTESIAN_POINT ( 'NONE',  ( -107.4999999999999716, -200.0000000000000000, 0.000000000000000000 ) ) ;
#4847=CARTESIAN_POINT ( 'NONE',  ( -97.49999999999997158, -133.9542832461881972, 9.999999999999996447 ) ) ;
#4850=CARTESIAN_POINT ( 'NONE',  ( -95.44734317237906396, -116.0775604631401450, 32.45031486599465609 ) ) ;
#4852=CARTESIAN_POINT ( 'NONE',  ( -139.7878999548352965, 7.953874699751952271, 23.37681481726362875 ) ) ;
#4854=CARTESIAN_POINT ( 'NONE',  ( -149.9962010962228476, 1.232532946391591056, 4.363522735748509795 ) ) ;
#4857=CARTESIAN_POINT ( 'NONE',  ( -123.6072353705779250, -84.98956761795039938, 49.99999999963072383 ) ) ;
#4859=VERTEX_POINT ( 'NONE', #17078 ) ;
#4860=B_SPLINE_CURVE_WITH_KNOTS ( 'NONE', 3,
 ( #4978, #6410, #17463, #11096, #17359, #15817, #5278, #3434, #17758, #2107, #3333, #6811, #13038, #19294, #18996, #9671, #9771, #11505, #3731, #16022, #2006, #9972, #160, #15918, #14381, #12631 ),
 .UNSPECIFIED., .F., .F.,
 ( 4, 2, 2, 2, 2, 2, 2, 2, 2, 2, 2, 2, 4 ),
 ( 0.000000000000000000, 0.001429785831555268043, 0.002144678747332922665, 0.002859571663110577287, 0.004289357494665905178, 0.005719143326221231768, 0.007148929157776559226, 0.008578714989331886684, 0.01143828665244248435, 0.01429785831555308029, 0.01572764414710837999, 0.01715742997866371439, 0.02287657330488496871 ),
 .UNSPECIFIED. ) ;
#4861=CARTESIAN_POINT ( 'NONE',  ( -159.9599531637108782, -36.50981547337168109, 39.99999999999999289 ) ) ;
#4863=CIRCLE ( 'NONE', #7450, 99.99999999999997158 ) ;
#4872=CARTESIAN_POINT ( 'NONE',  ( 0.000000000000000000, 164.0736214083062805, 39.99999999999999289 ) ) ;
#4873=VECTOR ( 'NONE', #11877, 1000.000000000000000 ) ;
#4874=CARTESIAN_POINT ( 'NONE',  ( -150.0000000000000000, 0.000000000000000000, 5.000000000000011546 ) ) ;
#4875=TOROIDAL_SURFACE ( 'NONE', #9753, 110.0000000000000142, 30.00000000000000000 ) ;
#4876=TOROIDAL_SURFACE ( 'NONE', #14348, 110.0000000000000142, 40.00000000000000000 ) ;
#4883=EDGE_CURVE ( 'NONE', #15236, #2173, #16674, .T. ) ;
#4884=ORIENTED_EDGE ( 'NONE', *, *, #6362, .F. ) ;
#4885=CARTESIAN_POINT ( 'NONE',  ( 134.9140359355661758, -65.56103033673134917, 33.73225304246028600 ) ) ;
#4889=ORIENTED_EDGE ( 'NONE', *, *, #2361, .F. ) ;
#4895=ORIENTED_EDGE ( 'NONE', *, *, #11106, .T. ) ;
#4899=CARTESIAN_POINT ( 'NONE',  ( -102.6638558517306166, -126.6149147318370041, 38.77018177895282491 ) ) ;
#4900=CARTESIAN_POINT ( 'NONE',  ( 7.500000000000006217, 164.0736214083062805, 39.99999999999999289 ) ) ;
#4903=CARTESIAN_POINT ( 'NONE',  ( 133.3341203894445641, -68.71829099011287667, -0.6771230101111865851 ) ) ;
#4906=CARTESIAN_POINT ( 'NONE',  ( -96.67593751107419564, 105.2677311041483392, -32.72576864185690226 ) ) ;
#4913=CARTESIAN_POINT ( 'NONE',  ( -75.02042969003670692, 118.2029424473213197, 2.920782463702978671 ) ) ;
#4915=DIRECTION ( 'NONE',  ( 0.000000000000000000, 0.000000000000000000, -1.000000000000000000 ) ) ;
#4922=AXIS2_PLACEMENT_3D ( 'NONE', #18947, #11045, #8183 ) ;
#4925=CARTESIAN_POINT ( 'NONE',  ( -135.9903138276601737, 55.59603877235524294, -25.41015113300352368 ) ) ;
#4929=DIRECTION ( 'NONE',  ( 0.000000000000000000, 0.000000000000000000, 1.000000000000000000 ) ) ;
#4938=CIRCLE ( 'NONE', #9509, 7.500000000000007105 ) ;
#4939=CARTESIAN_POINT ( 'NONE',  ( 99.73778183779745632, -112.0462389701484511, 50.00000000040667203 ) ) ;
#4942=CARTESIAN_POINT ( 'NONE',  ( -70.84156478054282502, 132.2175582643460245, 13.17469413506393217 ) ) ;
#4950=EDGE_LOOP ( 'NONE', ( #3759, #1197, #17031, #7888 ) ) ;
#4951=AXIS2_PLACEMENT_3D ( 'NONE', #4539, #6081, #10871 ) ;
#4956=CARTESIAN_POINT ( 'NONE',  ( -102.7594822686546507, -126.4624059756590810, 38.81042005228335512 ) ) ;
#4957=DIRECTION ( 'NONE',  ( -0.7818314824680221431, -0.6234898018587431423, 0.000000000000000000 ) ) ;
#4959=CARTESIAN_POINT ( 'NONE',  ( -189.9999999999988916, 275.0000000000000000, 5.000000000000268230 ) ) ;
#4962=DIRECTION ( 'NONE',  ( -1.000000000000000000, 0.000000000000000000, 0.000000000000000000 ) ) ;
#4963=ORIENTED_EDGE ( 'NONE', *, *, #10236, .F. ) ;
#4965=CARTESIAN_POINT ( 'NONE',  ( -125.0787927518813518, 50.79647550709884030, -26.58908968555560648 ) ) ;
#4968=ORIENTED_EDGE ( 'NONE', *, *, #11278, .F. ) ;
#4972=LINE ( 'NONE', #7919, #196 ) ;
#4974=ORIENTED_EDGE ( 'NONE', *, *, #11538, .T. ) ;
#4975=DIRECTION ( 'NONE',  ( 1.000000000000000000, 0.000000000000000000, 0.000000000000000000 ) ) ;
#4977=DIRECTION ( 'NONE',  ( -1.000000000000000000, 0.000000000000000000, 0.000000000000000000 ) ) ;
#4978=CARTESIAN_POINT ( 'NONE',  ( 97.50000000000001421, -133.9542832461881119, 30.00000000000000000 ) ) ;
#4982=CARTESIAN_POINT ( 'NONE',  ( 134.7188131032333729, -72.93593548660993520, 30.00000000000000000 ) ) ;
#4991=ORIENTED_EDGE ( 'NONE', *, *, #10034, .F. ) ;
#4994=DIRECTION ( 'NONE',  ( 0.3427509529624095941, 0.9394263059140722794, -0.000000000000000000 ) ) ;
#4999=CARTESIAN_POINT ( 'NONE',  ( -130.9868171408399462, -91.88282611735539263, -10.00000000000000355 ) ) ;
#5001=AXIS2_PLACEMENT_3D ( 'NONE', #2064, #5036, #12688 ) ;
#5007=EDGE_CURVE ( 'NONE', #16722, #3030, #18028, .T. ) ;
#5011=CARTESIAN_POINT ( 'NONE',  ( -159.9599531637108782, -36.50981547337168109, 39.99999999999999289 ) ) ;
#5012=CARTESIAN_POINT ( 'NONE',  ( -75.49180387445471752, 117.9024752767885786, -0.8621022543900443980 ) ) ;
#5017=VECTOR ( 'NONE', #16848, 1000.000000000000000 ) ;
#5018=ORIENTED_EDGE ( 'NONE', *, *, #5379, .T. ) ;
#5019=ORIENTED_EDGE ( 'NONE', *, *, #19885, .T. ) ;
#5020=DIRECTION ( 'NONE',  ( -0.000000000000000000, -0.000000000000000000, 1.000000000000000000 ) ) ;
#5024=ORIENTED_EDGE ( 'NONE', *, *, #12344, .F. ) ;
#5026=CARTESIAN_POINT ( 'NONE',  ( 159.9599531637113330, -36.50981547336952104, 39.99999999999999289 ) ) ;
#5032=VERTEX_POINT ( 'NONE', #393 ) ;
#5036=DIRECTION ( 'NONE',  ( -0.000000000000000000, -0.000000000000000000, -1.000000000000000000 ) ) ;
#5037=CARTESIAN_POINT ( 'NONE',  ( 103.8725996235405518, -124.7053175801592602, 39.32360563185468294 ) ) ;
#5041=CARTESIAN_POINT ( 'NONE',  ( -70.05487284751588106, 132.6360328284314392, 7.773882658412580859 ) ) ;
#5042=AXIS2_PLACEMENT_3D ( 'NONE', #2237, #8664, #11537 ) ;
#5045=VERTEX_POINT ( 'NONE', #191 ) ;
#5050=EDGE_CURVE ( 'NONE', #4182, #4447, #766, .T. ) ;
#5051=CARTESIAN_POINT ( 'NONE',  ( -149.7511488714461620, 8.920208118124556051, 9.601641421770001017 ) ) ;
#5053=STYLED_ITEM ( 'NONE', ( #2645 ), #1054 ) ;
#5061=CIRCLE ( 'NONE', #799, 30.00000000000000000 ) ;
#5063=CARTESIAN_POINT ( 'NONE',  ( -176.7850001792984926, -190.0000000000000284, 6.572490470375933036 ) ) ;
#5064=FACE_OUTER_BOUND ( 'NONE', #11938, .T. ) ;
#5066=CARTESIAN_POINT ( 'NONE',  ( -117.6617105120774625, 62.20691784305332561, -29.20604482175252414 ) ) ;
#5076=DIRECTION ( 'NONE',  ( -0.2225209339563195554, 0.9749279121818223981, 0.000000000000000000 ) ) ;
#5085=VECTOR ( 'NONE', #1265, 1000.000000000000000 ) ;
#5093=ORIENTED_EDGE ( 'NONE', *, *, #15855, .T. ) ;
#5100=CARTESIAN_POINT ( 'NONE',  ( 123.6373235125731469, -84.94667440144652915, -10.00000000000000000 ) ) ;
#5103=CARTESIAN_POINT ( 'NONE',  ( -29.99999999999887379, 265.0000000000000000, 4.999999999999158007 ) ) ;
#5110=CARTESIAN_POINT ( 'NONE',  ( -74.99285178184982215, 118.2204394347531604, 5.472170298398729926 ) ) ;
#5118=AXIS2_PLACEMENT_3D ( 'NONE', #15478, #9128, #1464 ) ;
#5124=EDGE_CURVE ( 'NONE', #11258, #7556, #3670, .T. ) ;
#5125=CARTESIAN_POINT ( 'NONE',  ( 163.5019688434126977, -20.99123081650019529, 39.99999999999999289 ) ) ;
#5128=DIRECTION ( 'NONE',  ( 0.000000000000000000, 0.000000000000000000, -1.000000000000000000 ) ) ;
#5132=CARTESIAN_POINT ( 'NONE',  ( 110.0000000000000142, 0.000000000000000000, -9.999999999999994671 ) ) ;
#5134=FACE_OUTER_BOUND ( 'NONE', #8850, .T. ) ;
#5137=CARTESIAN_POINT ( 'NONE',  ( 98.08728810296497613, -113.5042871117747865, 38.12342019507656232 ) ) ;
#5146=CIRCLE ( 'NONE', #14930, 15.91767397667354800 ) ;
#5147=VERTEX_POINT ( 'NONE', #2336 ) ;
#5151=CARTESIAN_POINT ( 'NONE',  ( -132.7010181243791465, 70.09019636137327325, 38.03942095735952478 ) ) ;
#5154=CARTESIAN_POINT ( 'NONE',  ( 133.2435246741110006, -68.89240257401093004, 40.00000000000000000 ) ) ;
#5155=CARTESIAN_POINT ( 'NONE',  ( -92.41621553527373578, -118.1510961661445407, -7.909716053491956167 ) ) ;
#5157=CARTESIAN_POINT ( 'NONE',  ( 0.000000000000000000, 0.000000000000000000, -100.0000000000000000 ) ) ;
#5165=EDGE_LOOP ( 'NONE', ( #7138, #8339, #15488, #6548 ) ) ;
#5166=EDGE_CURVE ( 'NONE', #11868, #8819, #3376, .T. ) ;
#5167=CARTESIAN_POINT ( 'NONE',  ( -126.3908400843113924, 48.63710208285993275, -25.92855131512484590 ) ) ;
#5170=EDGE_LOOP ( 'NONE', ( #117, #2587, #2839, #14519, #9757, #16747 ) ) ;
#5172=ORIENTED_EDGE ( 'NONE', *, *, #2992, .T. ) ;
#5174=DIRECTION ( 'NONE',  ( -0.000000000000000000, -0.000000000000000000, 1.000000000000000000 ) ) ;
#5175=EDGE_CURVE ( 'NONE', #10874, #7342, #13830, .T. ) ;
#5176=CARTESIAN_POINT ( 'NONE',  ( -134.9931224044436249, -65.39776452395025785, 7.096802314759633745 ) ) ;
#5186=CIRCLE ( 'NONE', #6816, 15.91767397667354444 ) ;
#5192=EDGE_LOOP ( 'NONE', ( #10183, #18156 ) ) ;
#5198=FACE_BOUND ( 'NONE', #17469, .T. ) ;
#5201=CARTESIAN_POINT ( 'NONE',  ( 130.7962991791399077, -73.43504534872144518, -5.497766754562231739 ) ) ;
#5202=DIRECTION ( 'NONE',  ( 0.000000000000000000, 0.000000000000000000, 1.000000000000000000 ) ) ;
#5210=CARTESIAN_POINT ( 'NONE',  ( 83.21341172527402819, -124.8022162803316348, 37.02557696701107659 ) ) ;
#5211=VECTOR ( 'NONE', #16139, 1000.000000000000000 ) ;
#5218=VERTEX_POINT ( 'NONE', #17697 ) ;
#5229=CARTESIAN_POINT ( 'NONE',  ( 100.6969204557048414, -129.5542747642291772, 2.663644724477163717 ) ) ;
#5233=CARTESIAN_POINT ( 'NONE',  ( 0.000000000000000000, 0.000000000000000000, 49.99999999999999289 ) ) ;
#5237=EDGE_CURVE ( 'NONE', #10908, #301, #11224, .T. ) ;
#5239=CARTESIAN_POINT ( 'NONE',  ( -102.9658523914788617, 109.0818325198187893, 44.38238497178959108 ) ) ;
#5242=EDGE_CURVE ( 'NONE', #14660, #15773, #2410, .T. ) ;
#5243=ORIENTED_EDGE ( 'NONE', *, *, #548, .F. ) ;
#5245=CARTESIAN_POINT ( 'NONE',  ( -15.91767397667354800, 141.9028892025177413, 39.99999999999999289 ) ) ;
#5249=CARTESIAN_POINT ( 'NONE',  ( -99.98138848894345188, -130.5820681961508853, 3.371015809596708657 ) ) ;
#5253=VECTOR ( 'NONE', #2978, 1000.000000000000000 ) ;
#5255=CARTESIAN_POINT ( 'NONE',  ( 0.000000000000000000, 0.000000000000000000, -10.00000000000000178 ) ) ;
#5258=LINE ( 'NONE', #1987, #14555 ) ;
#5262=EDGE_CURVE ( 'NONE', #14061, #11180, #6005, .T. ) ;
#5266=ORIENTED_EDGE ( 'NONE', *, *, #1033, .T. ) ;
#5271=LINE ( 'NONE', #12930, #14031 ) ;
#5274=CARTESIAN_POINT ( 'NONE',  ( -133.3574802752804658, -81.67441013338864764, 1.778968245714176666 ) ) ;
#5276=CARTESIAN_POINT ( 'NONE',  ( -86.01343624116279329, 31.38211805825948630, 40.00000000000000000 ) ) ;
#5278=CARTESIAN_POINT ( 'NONE',  ( 97.83161216922243852, -133.5187961265288266, 32.56398726576716740 ) ) ;
#5287=VERTEX_POINT ( 'NONE', #6010 ) ;
#5290=LINE ( 'NONE', #11513, #19704 ) ;
#5291=ORIENTED_EDGE ( 'NONE', *, *, #12661, .T. ) ;
#5296=FACE_OUTER_BOUND ( 'NONE', #15970, .T. ) ;
#5299=CARTESIAN_POINT ( 'NONE',  ( -107.4999999999999716, -200.0000000000000000, 10.00000000000000178 ) ) ;
#5303=CARTESIAN_POINT ( 'NONE',  ( -138.7698490687724586, -23.27885928005511218, -14.95860281343817633 ) ) ;
#5304=DIRECTION ( 'NONE',  ( -1.000000000000000000, 0.000000000000000000, 0.000000000000000000 ) ) ;
#5310=EDGE_CURVE ( 'NONE', #6137, #13930, #16824, .T. ) ;
#5315=CARTESIAN_POINT ( 'NONE',  ( -91.69207598197974107, -118.7138234487252930, 47.50433883429951720 ) ) ;
#5318=CARTESIAN_POINT ( 'NONE',  ( -78.68887634719366986, -147.8252249328922687, 39.99999999999999289 ) ) ;
#5319=CARTESIAN_POINT ( 'NONE',  ( 101.4288913641181864, -128.4806265586112488, 2.048058698311194803 ) ) ;
#5321=CIRCLE ( 'NONE', #3027, 9.999999999999994671 ) ;
#5322=DIRECTION ( 'NONE',  ( -0.2225209339563047894, -0.9749279121818258398, 0.000000000000000000 ) ) ;
#5324=EDGE_LOOP ( 'NONE', ( #10540, #15253, #1165, #4889 ) ) ;
#5327=VECTOR ( 'NONE', #1852, 1000.000000000000000 ) ;
#5329=CARTESIAN_POINT ( 'NONE',  ( 100.7812500000000142, -111.0996833858562667, 50.00000000000000000 ) ) ;
#5334=ORIENTED_EDGE ( 'NONE', *, *, #11927, .T. ) ;
#5346=CARTESIAN_POINT ( 'NONE',  ( -95.64785785032820797, -115.7351073149044822, 5.855624241335786628 ) ) ;
#5353=LINE ( 'NONE', #5448, #14356 ) ;
#5360=VERTEX_POINT ( 'NONE', #5802 ) ;
#5367=EDGE_CURVE ( 'NONE', #14347, #16722, #4102, .T. ) ;
#5373=CARTESIAN_POINT ( 'NONE',  ( -132.6415777375414393, -85.19230204982613941, 0.7648825228462121650 ) ) ;
#5376=CARTESIAN_POINT ( 'NONE',  ( 0.000000000000000000, 60.00000000000000000, -105.0000000000000142 ) ) ;
#5378=ORIENTED_EDGE ( 'NONE', *, *, #10581, .T. ) ;
#5379=EDGE_CURVE ( 'NONE', #17491, #13285, #18049, .T. ) ;
#5380=ORIENTED_EDGE ( 'NONE', *, *, #6758, .F. ) ;
#5381=ORIENTED_EDGE ( 'NONE', *, *, #6004, .F. ) ;
#5385=EDGE_LOOP ( 'NONE', ( #8767, #17595, #10131, #14161 ) ) ;
#5387=PLANE ( 'NONE',  #5701 ) ;
#5389=VERTEX_POINT ( 'NONE', #9969 ) ;
#5390=EDGE_CURVE ( 'NONE', #17491, #6085, #7051, .T. ) ;
#5392=LINE ( 'NONE', #4046, #19784 ) ;
#5395=EDGE_LOOP ( 'NONE', ( #18813, #13481, #5680, #8239, #4884 ) ) ;
#5413=ADVANCED_FACE ( 'NONE', ( #2495 ), #3728, .F. ) ;
#5419=CARTESIAN_POINT ( 'NONE',  ( -126.7720928841325474, -80.18313274224119880, 49.03856716278833972 ) ) ;
#5420=CARTESIAN_POINT ( 'NONE',  ( 97.77735676332858361, -133.5903492488113500, 7.649607847903932445 ) ) ;
#5421=TOROIDAL_SURFACE ( 'NONE', #17510, 110.0000000000000142, 30.00000000000000000 ) ;
#5422=ADVANCED_FACE ( 'NONE', ( #13420 ), #17499, .F. ) ;
#5428=DIRECTION ( 'NONE',  ( -1.000000000000000000, 0.000000000000000000, 0.000000000000000000 ) ) ;
#5431=B_SPLINE_CURVE_WITH_KNOTS ( 'NONE', 3,
 ( #16190, #1762, #536, #17431, #11270, #2179, #3406, #8301, #19067, #17724, #9733, #19157, #5151, #12804, #7997, #13001, #14243, #222, #14547, #12903, #3701, #6479, #12701, #18964, #11376, #14447, #16087, #3603, #5051, #8095, #6583, #9637, #326, #15887 ),
 .UNSPECIFIED., .F., .F.,
 ( 4, 2, 2, 2, 2, 2, 2, 2, 2, 2, 2, 2, 2, 2, 2, 2, 4 ),
 ( 0.08723304891271140005, 0.09476463103839000146, 0.1022962131640685890, 0.1060620042269078966, 0.1098277952897471904, 0.1173593774154258196, 0.1324225416667830502, 0.1399541237924616655, 0.1437199148553010009, 0.1474857059181403085, 0.1625488701694974836, 0.1776120344208546864, 0.1851436165465332739, 0.1926751986722118892, 0.2002067807978905045, 0.2039725718607297567, 0.2077383629235690921 ),
 .UNSPECIFIED. ) ;
#5432=DIRECTION ( 'NONE',  ( -0.9749279121818257288, 0.2225209339563050392, -0.000000000000000000 ) ) ;
#5440=CARTESIAN_POINT ( 'NONE',  ( 99.73767742489731347, -112.0463336856532521, -10.00000000004823519 ) ) ;
#5441=CARTESIAN_POINT ( 'NONE',  ( -95.50801338651713479, -116.1654322105520265, 8.498518821464802642 ) ) ;
#5448=CARTESIAN_POINT ( 'NONE',  ( 176.1792632384392334, -186.5724904703758682, 40.00000000000000000 ) ) ;
#5453=DIRECTION ( 'NONE',  ( -0.9394263059140725014, 0.3427509529624092055, 0.000000000000000000 ) ) ;
#5457=VERTEX_POINT ( 'NONE', #19977 ) ;
#5462=DIRECTION ( 'NONE',  ( -0.9749279121818257288, 0.2225209339563050392, -0.000000000000000000 ) ) ;
#5466=CARTESIAN_POINT ( 'NONE',  ( -123.6158562626643516, -84.97727779989590147, -9.999999999476957058 ) ) ;
#5467=CARTESIAN_POINT ( 'NONE',  ( 132.7096788433826191, -70.03826381905518872, 5.661456724840400412 ) ) ;
#5468=CARTESIAN_POINT ( 'NONE',  ( 135.1060089022256534, -65.16414933467420667, 49.99999999999999289 ) ) ;
#5488=CIRCLE ( 'NONE', #16925, 7.500000000000006217 ) ;
#5499=ADVANCED_FACE ( 'NONE', ( #1572, #7807, #19774, #3613, #8103, #11073 ), #10971, .F. ) ;
#5505=EDGE_LOOP ( 'NONE', ( #18357, #12771, #3377, #681, #669 ) ) ;
#5508=AXIS2_PLACEMENT_3D ( 'NONE', #7885, #1963, #9428 ) ;
#5509=EDGE_LOOP ( 'NONE', ( #4060, #17213 ) ) ;
#5510=CARTESIAN_POINT ( 'NONE',  ( -134.7652707650784407, -31.41120252075685215, -19.73219286542039441 ) ) ;
#5516=CARTESIAN_POINT ( 'NONE',  ( -133.1207282269168388, -69.13111487717780790, 41.23326533417627360 ) ) ;
#5522=ORIENTED_EDGE ( 'NONE', *, *, #13615, .T. ) ;
#5524=CARTESIAN_POINT ( 'NONE',  ( 85.34080972464066406, -123.3578596465555677, -1.367079200094239333 ) ) ;
#5526=VERTEX_POINT ( 'NONE', #15792 ) ;
#5529=EDGE_CURVE ( 'NONE', #5526, #4551, #11607, .T. ) ;
#5530=VERTEX_POINT ( 'NONE', #970 ) ;
#5531=ADVANCED_FACE ( 'NONE', ( #5296 ), #18069, .T. ) ;
#5534=EDGE_CURVE ( 'NONE', #13478, #2029, #13052, .T. ) ;
#5535=AXIS2_PLACEMENT_3D ( 'NONE', #464, #9971, #14680 ) ;
#5540=CARTESIAN_POINT ( 'NONE',  ( 101.9549241234500983, -127.6987521375408079, 1.655170884984768165 ) ) ;
#5541=CARTESIAN_POINT ( 'NONE',  ( -93.45568245712546229, -117.3306176392020888, -8.420502908542239595 ) ) ;
#5542=CARTESIAN_POINT ( 'NONE',  ( -84.30790708731534266, -124.0658650269852501, 0.4226591875635389295 ) ) ;
#5545=DIRECTION ( 'NONE',  ( -0.000000000000000000, -0.000000000000000000, -1.000000000000000000 ) ) ;
#5546=CARTESIAN_POINT ( 'NONE',  ( -60.00000000000000000, -2.094888803305880013E-13, -105.0000000000000142 ) ) ;
#5551=DIRECTION ( 'NONE',  ( -1.000000000000000000, 0.000000000000000000, 0.000000000000000000 ) ) ;
#5553=EDGE_CURVE ( 'NONE', #3260, #5786, #5392, .T. ) ;
#5554=ORIENTED_EDGE ( 'NONE', *, *, #2992, .F. ) ;
#5560=CARTESIAN_POINT ( 'NONE',  ( 134.6687524777004228, -73.33058021821595673, 8.085668793728526538 ) ) ;
#5561=CARTESIAN_POINT ( 'NONE',  ( -131.9010376021428783, -71.43117396976207090, -3.793297712624513540 ) ) ;
#5566=LINE ( 'NONE', #11885, #13034 ) ;
#5567=CARTESIAN_POINT ( 'NONE',  ( -128.7737027234273626, -76.92703321535461214, -7.688188765993792195 ) ) ;
#5568=CARTESIAN_POINT ( 'NONE',  ( 134.1858200530627983, -67.03963421358798769, 2.112429552066504179 ) ) ;
#5569=FACE_OUTER_BOUND ( 'NONE', #12440, .T. ) ;
#5570=DIRECTION ( 'NONE',  ( 0.000000000000000000, 0.000000000000000000, -1.000000000000000000 ) ) ;
#5578=VERTEX_POINT ( 'NONE', #11803 ) ;
#5580=CARTESIAN_POINT ( 'NONE',  ( 78.68887634719571622, -147.8252249328912740, 49.99999999999999289 ) ) ;
#5584=FACE_OUTER_BOUND ( 'NONE', #6798, .T. ) ;
#5586=VERTEX_POINT ( 'NONE', #3845 ) ;
#5588=ADVANCED_FACE ( 'NONE', ( #5584 ), #10282, .F. ) ;
#5589=DIRECTION ( 'NONE',  ( 0.000000000000000000, 0.000000000000000000, -1.000000000000000000 ) ) ;
#5598=EDGE_LOOP ( 'NONE', ( #10439, #14759 ) ) ;
#5612=DIRECTION ( 'NONE',  ( -0.6718749999999997780, -0.7406645559057084549, 0.000000000000000000 ) ) ;
#5617=DIRECTION ( 'NONE',  ( 0.000000000000000000, 0.000000000000000000, 1.000000000000000000 ) ) ;
#5623=VERTEX_POINT ( 'NONE', #7123 ) ;
#5634=VERTEX_POINT ( 'NONE', #5689 ) ;
#5636=CARTESIAN_POINT ( 'NONE',  ( 100.0290433904799698, -111.7820284656621368, 0.3810183304975476859 ) ) ;
#5641=CARTESIAN_POINT ( 'NONE',  ( -134.7188131032333445, -72.93593548660989256, 1.387778780781445676E-14 ) ) ;
#5649=DIRECTION ( 'NONE',  ( 0.000000000000000000, 0.000000000000000000, 1.000000000000000000 ) ) ;
#5650=AXIS2_PLACEMENT_3D ( 'NONE', #18746, #15355, #13610 ) ;
#5654=EDGE_CURVE ( 'NONE', #13855, #18133, #15565, .T. ) ;
#5658=CARTESIAN_POINT ( 'NONE',  ( 0.000000000000000000, 0.000000000000000000, -105.0000000000000142 ) ) ;
#5660=VERTEX_POINT ( 'NONE', #1284 ) ;
#5666=EDGE_CURVE ( 'NONE', #15773, #11866, #12518, .T. ) ;
#5669=CARTESIAN_POINT ( 'NONE',  ( -133.2435246741110006, -68.89240257401093004, 40.00000000000000000 ) ) ;
#5670=DIRECTION ( 'NONE',  ( -0.9009688679024212554, 0.4338837391175534575, 0.000000000000000000 ) ) ;
#5671=CARTESIAN_POINT ( 'NONE',  ( 134.7188131032333445, -72.93593548660993520, 10.00000000000000533 ) ) ;
#5672=VECTOR ( 'NONE', #13827, 1000.000000000000000 ) ;
#5679=VERTEX_POINT ( 'NONE', #18369 ) ;
#5680=ORIENTED_EDGE ( 'NONE', *, *, #4603, .F. ) ;
#5683=VECTOR ( 'NONE', #8609, 1000.000000000000000 ) ;
#5685=DIRECTION ( 'NONE',  ( -0.000000000000000000, -1.000000000000000000, -0.000000000000000000 ) ) ;
#5689=CARTESIAN_POINT ( 'NONE',  ( -78.68887634719366986, -147.8252249328922687, 49.99999999999999289 ) ) ;
#5694=CARTESIAN_POINT ( 'NONE',  ( -131.2500704209022615, -90.93860529234680712, 6.324512672832136480E-16 ) ) ;
#5696=CARTESIAN_POINT ( 'NONE',  ( 132.6415777375408425, -85.19230204981589338, 39.23511747715267717 ) ) ;
#5697=CIRCLE ( 'NONE', #18795, 7.500000000000007994 ) ;
#5701=AXIS2_PLACEMENT_3D ( 'NONE', #16237, #9884, #8348 ) ;
#5704=CARTESIAN_POINT ( 'NONE',  ( 0.000000000000000000, 0.000000000000000000, 0.000000000000000000 ) ) ;
#5706=VERTEX_POINT ( 'NONE', #13649 ) ;
#5709=CARTESIAN_POINT ( 'NONE',  ( -82.39904996721718078, -125.3411509769706242, 33.95830863599796601 ) ) ;
#5713=DIRECTION ( 'NONE',  ( -0.000000000000000000, -0.000000000000000000, 1.000000000000000000 ) ) ;
#5718=CARTESIAN_POINT ( 'NONE',  ( 110.0000000000000142, 0.000000000000000000, -9.999999999999994671 ) ) ;
#5722=CARTESIAN_POINT ( 'NONE',  ( -133.8357118474723961, -78.97256401901071854, 37.04716089610885632 ) ) ;
#5725=EDGE_LOOP ( 'NONE', ( #2767, #10803 ) ) ;
#5729=ADVANCED_FACE ( 'NONE', ( #16728 ), #15290, .F. ) ;
#5734=VERTEX_POINT ( 'NONE', #19897 ) ;
#5738=ORIENTED_EDGE ( 'NONE', *, *, #960, .T. ) ;
#5740=CARTESIAN_POINT ( 'NONE',  ( 99.33980890135488551, -112.3956798702031676, 0.8361447343429230239 ) ) ;
#5741=CARTESIAN_POINT ( 'NONE',  ( -100.0291087224201334, -111.7819692016497015, 0.3809852373215633636 ) ) ;
#5743=DIRECTION ( 'NONE',  ( 0.000000000000000000, 0.000000000000000000, 1.000000000000000000 ) ) ;
#5750=VERTEX_POINT ( 'NONE', #4664 ) ;
#5751=DIRECTION ( 'NONE',  ( 0.000000000000000000, 0.000000000000000000, 1.000000000000000000 ) ) ;
#5753=EDGE_LOOP ( 'NONE', ( #11316, #13208, #4839 ) ) ;
#5755=VERTEX_POINT ( 'NONE', #6206 ) ;
#5756=EDGE_CURVE ( 'NONE', #18071, #5912, #14895, .T. ) ;
#5758=ORIENTED_EDGE ( 'NONE', *, *, #10034, .T. ) ;
#5761=ORIENTED_EDGE ( 'NONE', *, *, #11490, .T. ) ;
#5764=CIRCLE ( 'NONE', #8053, 32.50000000000000000 ) ;
#5766=CARTESIAN_POINT ( 'NONE',  ( -95.54273718347639033, -115.6434791701697833, 49.24035574262877901 ) ) ;
#5767=DIRECTION ( 'NONE',  ( -1.000000000000000000, 0.000000000000000000, 0.000000000000000000 ) ) ;
#5769=DIRECTION ( 'NONE',  ( 1.000000000000000000, 0.000000000000000000, 0.000000000000000000 ) ) ;
#5770=CARTESIAN_POINT ( 'NONE',  ( -132.3052566686612579, -70.67971788940300826, -3.041505667804067947 ) ) ;
#5772=EDGE_CURVE ( 'NONE', #16770, #20118, #4972, .T. ) ;
#5773=CARTESIAN_POINT ( 'NONE',  ( 122.8001410695374602, -86.14014948502068592, -9.999999999999998224 ) ) ;
#5775=CARTESIAN_POINT ( 'NONE',  ( -135.1060089022256818, -65.16414933467422088, 30.00000000000000711 ) ) ;
#5783=EDGE_CURVE ( 'NONE', #18061, #1300, #2490, .T. ) ;
#5785=TOROIDAL_SURFACE ( 'NONE', #17230, 110.0000000000000142, 40.00000000000000000 ) ;
#5786=VERTEX_POINT ( 'NONE', #1589 ) ;
#5787=EDGE_CURVE ( 'NONE', #15721, #13855, #14172, .T. ) ;
#5791=CARTESIAN_POINT ( 'NONE',  ( -137.3668080473636053, -22.65449782367379328, -16.82459036858919177 ) ) ;
#5798=VECTOR ( 'NONE', #2431, 1000.000000000000000 ) ;
#5802=CARTESIAN_POINT ( 'NONE',  ( -156.4179374840092862, -52.02840013024096066, 39.99999999999999289 ) ) ;
#5807=ORIENTED_EDGE ( 'NONE', *, *, #4277, .T. ) ;
#5810=DIRECTION ( 'NONE',  ( 0.6234898018587433643, -0.7818314824680220321, 0.000000000000000000 ) ) ;
#5817=CARTESIAN_POINT ( 'NONE',  ( -126.0117988550010182, -81.37275256441674287, 49.38489965504906110 ) ) ;
#5819=LINE ( 'NONE', #9186, #817 ) ;
#5820=ORIENTED_EDGE ( 'NONE', *, *, #15534, .T. ) ;
#5822=CARTESIAN_POINT ( 'NONE',  ( -131.9731329243527682, -88.11278280481133152, 39.76642901553087484 ) ) ;
#5831=CARTESIAN_POINT ( 'NONE',  ( -82.23581699221313102, -125.4482974261014192, 32.97002058077946174 ) ) ;
#5833=EDGE_CURVE ( 'NONE', #5755, #16770, #6417, .T. ) ;
#5838=DIRECTION ( 'NONE',  ( 1.000000000000000000, 0.000000000000000000, 0.000000000000000000 ) ) ;
#5839=CARTESIAN_POINT ( 'NONE',  ( -98.08728810294334721, -113.5042871117647962, 1.876579804940954110 ) ) ;
#5840=AXIS2_PLACEMENT_3D ( 'NONE', #18724, #18935, #12875 ) ;
#5841=VECTOR ( 'NONE', #6028, 1000.000000000000227 ) ;
#5870=AXIS2_PLACEMENT_3D ( 'NONE', #18891, #4771, #12222 ) ;
#5874=CARTESIAN_POINT ( 'NONE',  ( -134.7264294273345797, -65.94569739564882127, 4.828444922764884240 ) ) ;
#5876=CARTESIAN_POINT ( 'NONE',  ( 132.0132531075724387, -71.33615934021467808, 3.697065622178481004 ) ) ;
#5879=CARTESIAN_POINT ( 'NONE',  ( -133.2712073793125569, -68.96827650305597501, 30.00000000000000000 ) ) ;
#5888=DIRECTION ( 'NONE',  ( 0.7406645559057084549, 0.6718749999999998890, -1.123343240388176004E-15 ) ) ;
#5896=AXIS2_PLACEMENT_3D ( 'NONE', #6340, #4700, #9398 ) ;
#5898=DIRECTION ( 'NONE',  ( 0.4338837391175526248, 0.9009688679024218105, -0.000000000000000000 ) ) ;
#5901=CIRCLE ( 'NONE', #16027, 7.500000000000006217 ) ;
#5902=CARTESIAN_POINT ( 'NONE',  ( 144.1130761623740568, -69.50842595698583182, 30.00000000000000000 ) ) ;
#5905=ADVANCED_FACE ( 'NONE', ( #9234 ), #11983, .F. ) ;
#5906=CARTESIAN_POINT ( 'NONE',  ( 122.8001410695374886, -86.14014948502062907, 40.00000000000000711 ) ) ;
#5912=VERTEX_POINT ( 'NONE', #13937 ) ;
#5923=DIRECTION ( 'NONE',  ( -0.000000000000000000, -0.000000000000000000, -1.000000000000000000 ) ) ;
#5925=ORIENTED_EDGE ( 'NONE', *, *, #7063, .F. ) ;
#5933=DIRECTION ( 'NONE',  ( -1.000000000000000000, 0.000000000000000000, 0.000000000000000000 ) ) ;
#5935=CARTESIAN_POINT ( 'NONE',  ( -110.0000000000000142, 86.60254037844390496, 39.99999999999997868 ) ) ;
#5936=EDGE_CURVE ( 'NONE', #9122, #9886, #7068, .T. ) ;
#5941=ORIENTED_EDGE ( 'NONE', *, *, #10899, .T. ) ;
#5942=CARTESIAN_POINT ( 'NONE',  ( -97.58310720701108210, -133.8455726501527181, 31.29999797859053956 ) ) ;
#5945=CARTESIAN_POINT ( 'NONE',  ( 0.000000000000000000, 0.000000000000000000, -49.99999999999999289 ) ) ;
#5946=ORIENTED_EDGE ( 'NONE', *, *, #13127, .F. ) ;
#5949=CARTESIAN_POINT ( 'NONE',  ( -136.4619910415503625, -31.11745988142876129, -11.67418830189604328 ) ) ;
#5954=CARTESIAN_POINT ( 'NONE',  ( 84.12422660803940744, -124.1903156958371000, 39.21023289894657893 ) ) ;
#5955=VERTEX_POINT ( 'NONE', #10020 ) ;
#5961=VECTOR ( 'NONE', #16019, 1000.000000000000000 ) ;
#5969=DIRECTION ( 'NONE',  ( -0.5742676632334714482, -0.8186676071302495528, 0.000000000000000000 ) ) ;
#5974=CARTESIAN_POINT ( 'NONE',  ( -134.3415992761221105, -66.72651222969516027, 2.774043998594589056 ) ) ;
#5975=CARTESIAN_POINT ( 'NONE',  ( 134.2478682171850437, -76.37034190854629401, 4.533283974515958548 ) ) ;
#5977=CIRCLE ( 'NONE', #10522, 7.500000000000012434 ) ;
#5979=CYLINDRICAL_SURFACE ( 'NONE', #19639, 7.500000000000020428 ) ;
#5980=CARTESIAN_POINT ( 'NONE',  ( -135.0085555318103729, -65.36720921928038308, 33.00376037643530935 ) ) ;
#5982=ORIENTED_EDGE ( 'NONE', *, *, #11603, .F. ) ;
#5991=EDGE_CURVE ( 'NONE', #9376, #6851, #10864, .T. ) ;
#5992=CARTESIAN_POINT ( 'NONE',  ( -138.8349868765292854, -24.00226663467886468, 24.84023710039527799 ) ) ;
#5993=EDGE_CURVE ( 'NONE', #11053, #5734, #11071, .T. ) ;
#5995=CYLINDRICAL_SURFACE ( 'NONE', #3847, 34.99999999999997868 ) ;
#6002=CARTESIAN_POINT ( 'NONE',  ( -134.4445132543467309, -75.00751837915889553, 5.690310535856665908 ) ) ;
#6004=EDGE_CURVE ( 'NONE', #13843, #5526, #11453, .T. ) ;
#6005=CIRCLE ( 'NONE', #17836, 7.500000000000000000 ) ;
#6006=CARTESIAN_POINT ( 'NONE',  ( 130.9868171408399746, -91.88282611735534999, 40.00000000000000000 ) ) ;
#6010=CARTESIAN_POINT ( 'NONE',  ( 32.50000000000000000, 3.980102097228897837E-15, -105.0000000000000142 ) ) ;
#6011=ORIENTED_EDGE ( 'NONE', *, *, #7642, .T. ) ;
#6014=CARTESIAN_POINT ( 'NONE',  ( -181.0783081749256667, -200.0000000000000853, 10.00000000000000178 ) ) ;
#6015=AXIS2_PLACEMENT_3D ( 'NONE', #20225, #4579, #4471 ) ;
#6017=ORIENTED_EDGE ( 'NONE', *, *, #2616, .T. ) ;
#6018=EDGE_CURVE ( 'NONE', #16017, #2735, #17843, .T. ) ;
#6027=FACE_BOUND ( 'NONE', #5598, .T. ) ;
#6028=DIRECTION ( 'NONE',  ( -0.9749279121818226201, -0.2225209339563185285, 0.000000000000000000 ) ) ;
#6031=EDGE_CURVE ( 'NONE', #5360, #3019, #4745, .T. ) ;
#6049=CARTESIAN_POINT ( 'NONE',  ( 82.18707601317576916, -125.4802243595265736, 7.400004042823632666 ) ) ;
#6054=LINE ( 'NONE', #15046, #5253 ) ;
#6060=CARTESIAN_POINT ( 'NONE',  ( 101.4383890160197126, -128.4709723833431383, 37.98072183278354430 ) ) ;
#6074=CARTESIAN_POINT ( 'NONE',  ( -107.4999999999999716, -118.5063289449133777, 40.00000000000000711 ) ) ;
#6076=FACE_OUTER_BOUND ( 'NONE', #13508, .T. ) ;
#6079=CARTESIAN_POINT ( 'NONE',  ( -134.7130977013099198, -72.98159303034539391, 9.251533979818299613 ) ) ;
#6080=CARTESIAN_POINT ( 'NONE',  ( 133.6156149914907303, -80.24737158797387337, 2.358024411017839661 ) ) ;
#6081=DIRECTION ( 'NONE',  ( 0.000000000000000000, 0.000000000000000000, 1.000000000000000000 ) ) ;
#6084=CARTESIAN_POINT ( 'NONE',  ( -129.7375433114042096, -75.28992114163499139, 46.76778812272521435 ) ) ;
#6085=VERTEX_POINT ( 'NONE', #5318 ) ;
#6086=DIRECTION ( 'NONE',  ( -1.000000000000000000, 0.000000000000000000, 0.000000000000000000 ) ) ;
#6094=PLANE ( 'NONE',  #7006 ) ;
#6095=CARTESIAN_POINT ( 'NONE',  ( -15.91767397667354800, 149.1530343478547422, 49.99999999999999289 ) ) ;
#6096=ORIENTED_EDGE ( 'NONE', *, *, #242, .T. ) ;
#6097=CARTESIAN_POINT ( 'NONE',  ( -135.6462056290698968, -28.96440493867737587, -18.85007980121054771 ) ) ;
#6098=DIRECTION ( 'NONE',  ( 1.000000000000000000, 0.000000000000000000, 0.000000000000000000 ) ) ;
#6099=ORIENTED_EDGE ( 'NONE', *, *, #4033, .T. ) ;
#6108=CARTESIAN_POINT ( 'NONE',  ( 133.2472142827512869, -69.01451035582651627, 31.05647528840589544 ) ) ;
#6109=CARTESIAN_POINT ( 'NONE',  ( -176.7850001792984926, -190.0000000000000284, 33.42750952962406075 ) ) ;
#6113=ORIENTED_EDGE ( 'NONE', *, *, #5534, .F. ) ;
#6117=EDGE_LOOP ( 'NONE', ( #3522, #13539, #15252, #4438, #4343, #1577 ) ) ;
#6121=DIRECTION ( 'NONE',  ( 0.000000000000000000, 0.000000000000000000, 1.000000000000000000 ) ) ;
#6124=CARTESIAN_POINT ( 'NONE',  ( -150.0000000000000284, 0.000000000000000000, 49.99999999999999289 ) ) ;
#6132=EDGE_CURVE ( 'NONE', #7965, #17276, #3171, .T. ) ;
#6135=CARTESIAN_POINT ( 'NONE',  ( -134.5348546532066223, -74.34984901039666738, 33.58727947796721480 ) ) ;
#6136=CARTESIAN_POINT ( 'NONE',  ( -92.45893247793782166, 105.1283412284861214, 35.29463395659252711 ) ) ;
#6137=VERTEX_POINT ( 'NONE', #13268 ) ;
#6138=DIRECTION ( 'NONE',  ( -0.000000000000000000, -0.000000000000000000, 1.000000000000000000 ) ) ;
#6141=AXIS2_PLACEMENT_3D ( 'NONE', #13675, #15526, #1511 ) ;
#6154=CARTESIAN_POINT ( 'NONE',  ( -110.0000000000000142, 275.0000000000000000, -75.00000000000000000 ) ) ;
#6156=AXIS2_PLACEMENT_3D ( 'NONE', #16380, #2167, #3981 ) ;
#6161=EDGE_CURVE ( 'NONE', #18071, #11232, #17856, .T. ) ;
#6163=CARTESIAN_POINT ( 'NONE',  ( 91.90390622750021521, -118.5498891763774481, 47.62726813621947741 ) ) ;
#6166=PLANE ( 'NONE',  #19848 ) ;
#6167=LINE ( 'NONE', #16794, #19685 ) ;
#6175=FACE_OUTER_BOUND ( 'NONE', #11130, .T. ) ;
#6176=AXIS2_PLACEMENT_3D ( 'NONE', #5669, #3926, #755 ) ;
#6179=CARTESIAN_POINT ( 'NONE',  ( -159.9599531637108782, -36.50981547337168109, 39.99999999999999289 ) ) ;
#6181=CARTESIAN_POINT ( 'NONE',  ( 135.0831964404852954, -65.21150773178307247, 31.46019346751870316 ) ) ;
#6182=CARTESIAN_POINT ( 'NONE',  ( -103.5848300920826688, -125.1657093462234229, 39.20674415995744511 ) ) ;
#6187=CARTESIAN_POINT ( 'NONE',  ( 124.7133609680326032, -83.36099555804651118, -0.8783870393142805266 ) ) ;
#6190=DIRECTION ( 'NONE',  ( 0.3427509529624101492, -0.9394263059140720573, -0.000000000000000000 ) ) ;
#6192=CARTESIAN_POINT ( 'NONE',  ( -134.3546152455176355, -75.63949198389248352, 34.87809301592528755 ) ) ;
#6199=EDGE_LOOP ( 'NONE', ( #15926, #2250, #9115, #15038, #12898, #10732, #18439, #9436, #15076, #17218 ) ) ;
#6204=DIRECTION ( 'NONE',  ( 0.000000000000000000, 0.000000000000000000, 1.000000000000000000 ) ) ;
#6206=CARTESIAN_POINT ( 'NONE',  ( -85.53020504959707182, -140.9188050298390067, 39.99999999999999289 ) ) ;
#6209=CARTESIAN_POINT ( 'NONE',  ( -103.2107452891376198, 83.78616291780149083, -29.34215614146094353 ) ) ;
#6214=CARTESIAN_POINT ( 'NONE',  ( 135.1060089021447368, -65.16414933484200844, 30.74984108339598876 ) ) ;
#6222=DIRECTION ( 'NONE',  ( -0.000000000000000000, -0.000000000000000000, -1.000000000000000000 ) ) ;
#6236=CARTESIAN_POINT ( 'NONE',  ( -72.91900756452172061, 131.0832496385607158, -10.00000000000000178 ) ) ;
#6237=LINE ( 'NONE', #3262, #3879 ) ;
#6240=CARTESIAN_POINT ( 'NONE',  ( 134.1130761623740568, -69.50842595698583182, 30.00000000000000000 ) ) ;
#6241=CYLINDRICAL_SURFACE ( 'NONE', #13143, 15.91767397667354089 ) ;
#6253=DIRECTION ( 'NONE',  ( -1.000000000000000000, 0.000000000000000000, 0.000000000000000000 ) ) ;
#6256=CARTESIAN_POINT ( 'NONE',  ( 82.35314629726865121, -125.3713054028912950, 6.290984962544095005 ) ) ;
#6259=VECTOR ( 'NONE', #18274, 1000.000000000000000 ) ;
#6262=EDGE_LOOP ( 'NONE', ( #8217, #15103, #2688, #17395 ) ) ;
#6265=DIRECTION ( 'NONE',  ( 0.000000000000000000, 0.000000000000000000, 1.000000000000000000 ) ) ;
#6266=CARTESIAN_POINT ( 'NONE',  ( 99.06221739375077107, -131.8607669219688887, 35.36983001673655025 ) ) ;
#6268=ADVANCED_FACE ( 'NONE', ( #2852, #9077, #2956, #6027, #15214, #12346 ), #13887, .F. ) ;
#6278=CARTESIAN_POINT ( 'NONE',  ( -98.69444885161524894, -132.3639744934813791, 5.244265984552241910 ) ) ;
#6280=ORIENTED_EDGE ( 'NONE', *, *, #16624, .T. ) ;
#6286=EDGE_CURVE ( 'NONE', #10224, #65, #4668, .T. ) ;
#6287=CARTESIAN_POINT ( 'NONE',  ( -103.8658874392065599, -124.7161237612890687, 39.32103072359011264 ) ) ;
#6289=CARTESIAN_POINT ( 'NONE',  ( -118.0540516568924545, 75.28054536010147046, 39.07880203530302765 ) ) ;
#6293=CARTESIAN_POINT ( 'NONE',  ( -128.4532923017889345, -77.52586173742388098, 40.42418673595172862 ) ) ;
#6299=ORIENTED_EDGE ( 'NONE', *, *, #7107, .F. ) ;
#6302=ADVANCED_FACE ( 'NONE', ( #17587 ), #1716, .T. ) ;
#6304=VECTOR ( 'NONE', #2914, 1000.000000000000000 ) ;
#6313=CARTESIAN_POINT ( 'NONE',  ( 150.0000000000000284, 1.836970198721029747E-14, -10.00000000000000178 ) ) ;
#6315=CARTESIAN_POINT ( 'NONE',  ( 133.1515905083523705, -69.19806146150529003, 32.10257561466540466 ) ) ;
#6316=CARTESIAN_POINT ( 'NONE',  ( 134.6712220124679789, -73.31159846691426196, 31.91396761802506177 ) ) ;
#6327=CARTESIAN_POINT ( 'NONE',  ( -106.5749805965074728, -120.1845445602442624, 40.00000000000000000 ) ) ;
#6328=CARTESIAN_POINT ( 'NONE',  ( 85.53020504959901871, -140.9188050298377846, 49.99999999999999289 ) ) ;
#6330=VERTEX_POINT ( 'NONE', #6438 ) ;
#6335=DIRECTION ( 'NONE',  ( 0.9394263059140722794, -0.3427509529624098161, 0.000000000000000000 ) ) ;
#6338=CARTESIAN_POINT ( 'NONE',  ( 134.7188131032333445, -72.93593548660993520, 40.00000000000000711 ) ) ;
#6340=CARTESIAN_POINT ( 'NONE',  ( 0.000000000000000000, 0.000000000000000000, 49.99999999999999289 ) ) ;
#6344=CIRCLE ( 'NONE', #6015, 7.500000000000007994 ) ;
#6345=EDGE_LOOP ( 'NONE', ( #2704, #2654, #10491, #575 ) ) ;
#6349=CARTESIAN_POINT ( 'NONE',  ( -131.3857632021294535, 62.10379777574404869, -28.86798393970800092 ) ) ;
#6353=CARTESIAN_POINT ( 'NONE',  ( 83.25760956673217095, -124.7743995867201363, 2.742699998077471335 ) ) ;
#6359=EDGE_LOOP ( 'NONE', ( #19910, #10821, #5807, #17650 ) ) ;
#6362=EDGE_CURVE ( 'NONE', #5578, #65, #14404, .T. ) ;
#6364=CARTESIAN_POINT ( 'NONE',  ( 82.65886493344478936, -125.1699850288369191, 35.14462631893170652 ) ) ;
#6368=CARTESIAN_POINT ( 'NONE',  ( -71.24814492356442486, 131.9990795557087893, 14.95622185591408027 ) ) ;
#6381=DIRECTION ( 'NONE',  ( 0.000000000000000000, 0.000000000000000000, 1.000000000000000000 ) ) ;
#6384=CARTESIAN_POINT ( 'NONE',  ( -101.9549241234480803, -127.6987521375408363, 38.34482911501410030 ) ) ;
#6386=DIRECTION ( 'NONE',  ( 0.000000000000000000, 0.000000000000000000, 1.000000000000000000 ) ) ;
#6387=CARTESIAN_POINT ( 'NONE',  ( -96.48501399889541119, -114.8592206156971542, -9.502595028825394863 ) ) ;
#6388=( BOUNDED_SURFACE ( )  B_SPLINE_SURFACE ( 3, 2, ( 
 ( #15267, #19769, #6074 ),
 ( #16514, #1253, #11881 ),
 ( #4120, #10350, #16608 ),
 ( #2595, #8824, #15064 ),
 ( #5766, #11982, #17335 ),
 ( #4531, #228, #6287 ),
 ( #12399, #15477, #6182 ),
 ( #6487, #20181, #15692 ),
 ( #3207, #1673, #4956 ),
 ( #18662, #4638, #6384 ),
 ( #7899, #11070, #9445 ),
 ( #14044, #9233, #1462 ),
 ( #3004, #4850, #10863 ),
 ( #12600, #17118, #17017 ),
 ( #3311, #11173, #12498 ),
 ( #12706, #14145, #10764 ),
 ( #7691, #132, #18864 ),
 ( #13936, #3105, #10966 ),
 ( #9336, #15582, #1568 ),
 ( #9546, #7803, #4743 ),
 ( #33, #15786, #1771 ),
 ( #18763, #8003, #17227 ),
 ( #14249, #18969, #15229 ),
 ( #16775, #20146, #2765 ),
 ( #10825, #19734, #8988 ),
 ( #16679, #16875, #15442 ),
 ( #13799, #4393, #19833 ),
 ( #5831, #9092, #8890 ),
 ( #1214, #13484, #5942 ),
 ( #12156, #15035, #4495 ),
 ( #7456, #7262, #9197 ),
 ( #20044, #10619, #12050 ) ),
 .UNSPECIFIED., .F., .F., .F. ) 
 B_SPLINE_SURFACE_WITH_KNOTS ( ( 4, 2, 2, 2, 2, 2, 2, 2, 2, 2, 2, 2, 2, 2, 2, 4 ),
 ( 3, 3 ),
 ( 0.02531008572351745728, 0.02976618726483494168, 0.03422228880615242608, 0.03645033957681116654, 0.03867839034746990701, 0.04313449188878738794, 0.04424851727411675817, 0.04536254265944612840, 0.04759059343010486887, 0.04981864420076360933, 0.05093266958609297956, 0.05204669497142234980, 0.05650279651273983073, 0.05761682189806920096, 0.05873084728339857119, 0.06095889805405731859 ),
 ( 0.000000000000000000, 1.000000000000000000 ),
 .UNSPECIFIED. ) 
 GEOMETRIC_REPRESENTATION_ITEM ( )  RATIONAL_B_SPLINE_SURFACE ( (
 ( 1.000000000000000000, 0.7071067811865477948, 1.000000000000000000),
 ( 1.000000000000000000, 0.6938858163893895092, 1.000000000000000000),
 ( 1.000000000000000000, 0.6806631601997592540, 1.000000000000000000),
 ( 1.000000000000000000, 0.6542661407889984737, 1.000000000000000000),
 ( 1.000000000000000000, 0.6410910482671290378, 1.000000000000000000),
 ( 1.000000000000000000, 0.6214215355381913497, 1.000000000000000000),
 ( 1.000000000000000000, 0.6148567640636197762, 1.000000000000000000),
 ( 1.000000000000000000, 0.6019746658715365850, 1.000000000000000000),
 ( 1.000000000000000000, 0.5956402134854033026, 1.000000000000000000),
 ( 1.000000000000000000, 0.5769855966605448305, 1.000000000000000000),
 ( 1.000000000000000000, 0.5650096313357982902, 1.000000000000000000),
 ( 1.000000000000000000, 0.5507648555195425732, 1.000000000000000000),
 ( 1.000000000000000000, 0.5479490128870788679, 1.000000000000000000),
 ( 1.000000000000000000, 0.5424554856653597268, 1.000000000000000000),
 ( 1.000000000000000000, 0.5397704441657605878, 1.000000000000000000),
 ( 1.000000000000000000, 0.5319045985430522760, 1.000000000000000000),
 ( 1.000000000000000000, 0.5269125948469715048, 1.000000000000000000),
 ( 1.000000000000000000, 0.5174644824776444274, 1.000000000000000000),
 ( 1.000000000000000000, 0.5130081457584507731, 1.000000000000000000),
 ( 1.000000000000000000, 0.5067628861632463844, 1.000000000000000000),
 ( 1.000000000000000000, 0.5047490957320780458, 1.000000000000000000),
 ( 1.000000000000000000, 0.5009263418717803118, 1.000000000000000000),
 ( 1.000000000000000000, 0.4991119735066952279, 1.000000000000000000),
 ( 1.000000000000000000, 0.4905251103113591471, 1.000000000000000000),
 ( 1.000000000000000000, 0.4851887169573420033, 1.000000000000000000),
 ( 1.000000000000000000, 0.4806071066593465835, 1.000000000000000000),
 ( 1.000000000000000000, 0.4797938356042399377, 1.000000000000000000),
 ( 1.000000000000000000, 0.4784048377100982297, 1.000000000000000000),
 ( 1.000000000000000000, 0.4778282137465386104, 1.000000000000000000),
 ( 1.000000000000000000, 0.4764456491723553233, 1.000000000000000000),
 ( 1.000000000000000000, 0.4759864261380953310, 1.000000000000000000),
 ( 1.000000000000000000, 0.4759858191164941243, 1.000000000000000000) ) ) 
 REPRESENTATION_ITEM ( '' )  SURFACE ( )  );
#6391=DIRECTION ( 'NONE',  ( 0.000000000000000000, 0.000000000000000000, 1.000000000000000000 ) ) ;
#6392=CARTESIAN_POINT ( 'NONE',  ( -133.6156149914909008, -80.24737158797381653, 37.64197558898200668 ) ) ;
#6394=EDGE_CURVE ( 'NONE', #17239, #18566, #17550, .T. ) ;
#6395=FACE_OUTER_BOUND ( 'NONE', #10081, .T. ) ;
#6396=ADVANCED_FACE ( 'NONE', ( #3561 ), #9895, .F. ) ;
#6399=ORIENTED_EDGE ( 'NONE', *, *, #17137, .T. ) ;
#6406=CARTESIAN_POINT ( 'NONE',  ( 181.0783081749256951, -199.9999999999999716, 0.000000000000000000 ) ) ;
#6410=CARTESIAN_POINT ( 'NONE',  ( 97.50000000000000000, -133.9542832461881119, 30.48586822279154873 ) ) ;
#6412=ORIENTED_EDGE ( 'NONE', *, *, #4503, .T. ) ;
#6417=CIRCLE ( 'NONE', #8372, 15.91767397667354267 ) ;
#6419=VERTEX_POINT ( 'NONE', #13548 ) ;
#6421=B_SPLINE_CURVE_WITH_KNOTS ( 'NONE', 3,
 ( #3565, #8261, #3953, #16252, #5303, #11532, #2233, #588, #3665, #494, #16346, #7133 ),
 .UNSPECIFIED., .F., .F.,
 ( 4, 2, 2, 2, 2, 4 ),
 ( 0.000000000000000000, 0.004378549521624888058, 0.008757099043249776116, 0.01094637380406223229, 0.01313564856487468846, 0.01751419808649958346 ),
 .UNSPECIFIED. ) ;
#6425=DIRECTION ( 'NONE',  ( 0.000000000000000000, 0.000000000000000000, 1.000000000000000000 ) ) ;
#6430=DIRECTION ( 'NONE',  ( 0.000000000000000000, 0.000000000000000000, 1.000000000000000000 ) ) ;
#6431=DIRECTION ( 'NONE',  ( 0.000000000000000000, 0.000000000000000000, 1.000000000000000000 ) ) ;
#6433=DIRECTION ( 'NONE',  ( -0.000000000000000000, 0.000000000000000000, 1.000000000000000000 ) ) ;
#6438=CARTESIAN_POINT ( 'NONE',  ( 7.500000000000001776, 60.00000000000000000, -100.0000000000000000 ) ) ;
#6441=AXIS2_PLACEMENT_3D ( 'NONE', #2235, #18079, #13155 ) ;
#6444=CARTESIAN_POINT ( 'NONE',  ( 88.72241907111769876, -120.9490000788567130, 45.32939563125253102 ) ) ;
#6447=VERTEX_POINT ( 'NONE', #19696 ) ;
#6448=AXIS2_PLACEMENT_3D ( 'NONE', #19999, #1173, #20206 ) ;
#6449=EDGE_CURVE ( 'NONE', #2619, #9376, #10029, .T. ) ;
#6450=EDGE_LOOP ( 'NONE', ( #16473, #789 ) ) ;
#6459=FACE_OUTER_BOUND ( 'NONE', #13648, .T. ) ;
#6463=DIRECTION ( 'NONE',  ( 0.000000000000000000, 0.000000000000000000, 1.000000000000000000 ) ) ;
#6468=AXIS2_PLACEMENT_3D ( 'NONE', #7753, #15846, #12865 ) ;
#6470=CARTESIAN_POINT ( 'NONE',  ( -72.24243551186484069, 131.4596132301078057, -8.327469122224886888 ) ) ;
#6471=VECTOR ( 'NONE', #16120, 1000.000000000000000 ) ;
#6472=ORIENTED_EDGE ( 'NONE', *, *, #5756, .F. ) ;
#6479=CARTESIAN_POINT ( 'NONE',  ( -145.8049199971885344, 35.51790619049093323, 22.99421396143800678 ) ) ;
#6481=CARTESIAN_POINT ( 'NONE',  ( 0.000000000000000000, 164.0736214083062805, 39.99999999999999289 ) ) ;
#6483=DIRECTION ( 'NONE',  ( 1.000000000000000000, 0.000000000000000000, 0.000000000000000000 ) ) ;
#6487=CARTESIAN_POINT ( 'NONE',  ( -92.40373333587341165, -118.1608478542227942, 47.90302656145166083 ) ) ;
#6489=DIRECTION ( 'NONE',  ( -0.000000000000000000, -0.000000000000000000, 1.000000000000000000 ) ) ;
#6491=DIRECTION ( 'NONE',  ( -0.9749279121818226201, -0.2225209339563185285, 0.000000000000000000 ) ) ;
#6493=CARTESIAN_POINT ( 'NONE',  ( -134.4267602304430795, -75.13220794377609479, 34.41794545084487567 ) ) ;
#6494=VERTEX_POINT ( 'NONE', #1070 ) ;
#6495=CYLINDRICAL_SURFACE ( 'NONE', #19989, 7.500000000000000000 ) ;
#6503=CARTESIAN_POINT ( 'NONE',  ( -142.3282607959048960, -17.64421488672613947, -8.419224594817324103 ) ) ;
#6506=CARTESIAN_POINT ( 'NONE',  ( 0.000000000000000000, 0.000000000000000000, 39.99999999999999289 ) ) ;
#6507=AXIS2_PLACEMENT_3D ( 'NONE', #2644, #3963, #7334 ) ;
#6508=DIRECTION ( 'NONE',  ( 0.4338837391175526248, 0.9009688679024218105, -0.000000000000000000 ) ) ;
#6519=CARTESIAN_POINT ( 'NONE',  ( 133.0788080491229550, -69.33756331726938527, 32.62557982921207866 ) ) ;
#6520=CARTESIAN_POINT ( 'NONE',  ( 134.6433994324794412, -73.52870175801844255, 32.36516242777680219 ) ) ;
#6525=AXIS2_PLACEMENT_3D ( 'NONE', #3433, #17756, #4977 ) ;
#6533=DIRECTION ( 'NONE',  ( -0.4338837391175523472, -0.9009688679024219216, 0.000000000000000000 ) ) ;
#6536=DIRECTION ( 'NONE',  ( 0.8186676071302493307, 0.5742676632334713371, 0.000000000000000000 ) ) ;
#6542=FACE_BOUND ( 'NONE', #11056, .T. ) ;
#6543=CIRCLE ( 'NONE', #6507, 10.00000000000000888 ) ;
#6548=ORIENTED_EDGE ( 'NONE', *, *, #12349, .F. ) ;
#6551=VERTEX_POINT ( 'NONE', #10578 ) ;
#6553=DIRECTION ( 'NONE',  ( -1.000000000000000000, 0.000000000000000000, 0.000000000000000000 ) ) ;
#6554=ORIENTED_EDGE ( 'NONE', *, *, #16422, .F. ) ;
#6556=CYLINDRICAL_SURFACE ( 'NONE', #16010, 15.91767397667355510 ) ;
#6563=DIRECTION ( 'NONE',  ( 0.000000000000000000, 0.000000000000000000, 1.000000000000000000 ) ) ;
#6575=CARTESIAN_POINT ( 'NONE',  ( 0.000000000000000000, 0.000000000000000000, 49.99999999999999289 ) ) ;
#6583=CARTESIAN_POINT ( 'NONE',  ( -149.9377538849844882, 4.462546922558185081, 7.303857415559938282 ) ) ;
#6584=EDGE_LOOP ( 'NONE', ( #15552, #8121, #10567, #455 ) ) ;
#6585=AXIS2_PLACEMENT_3D ( 'NONE', #5376, #14681, #6912 ) ;
#6588=CARTESIAN_POINT ( 'NONE',  ( 131.6317334595287036, -71.92650142027842719, 44.25146303588275742 ) ) ;
#6593=CARTESIAN_POINT ( 'NONE',  ( 106.6880305650188205, 105.4403344747995988, 49.99999999999999289 ) ) ;
#6594=CARTESIAN_POINT ( 'NONE',  ( -29.99999999999887379, 275.0000000000000000, 12.49999999999916511 ) ) ;
#6595=ORIENTED_EDGE ( 'NONE', *, *, #17619, .T. ) ;
#6596=AXIS2_PLACEMENT_3D ( 'NONE', #11352, #14220, #15863 ) ;
#6597=CARTESIAN_POINT ( 'NONE',  ( -138.4582331060196623, 17.23264747863311896, -15.37944944523201585 ) ) ;
#6598=B_SPLINE_CURVE_WITH_KNOTS ( 'NONE', 3,
 ( #1675, #15892, #14047, #7903, #14357, #6387, #17438, #12603, #1871, #15791, #8102, #8006, #230, #333, #19553, #8608, #928, #17830, #10050, #5542, #16394, #16299, #14750, #11672, #3902, #18120, #7078, #2186, #8410, #14842 ),
 .UNSPECIFIED., .F., .F.,
 ( 4, 2, 2, 2, 2, 2, 2, 2, 2, 2, 2, 2, 2, 2, 4 ),
 ( 0.000000000000000000, 0.002170930610089446579, 0.004341861220178893158, 0.008683722440357753355, 0.01085465305044718519, 0.01302558366053661876, 0.01519651427062605059, 0.01736744488071548242, 0.02170930610089434956, 0.02388023671098378140, 0.02605116732107320629, 0.02822209793116263465, 0.02930756323620734363, 0.03039302854125205608, 0.03473488976143088158 ),
 .UNSPECIFIED. ) ;
#6599=ORIENTED_EDGE ( 'NONE', *, *, #5993, .T. ) ;
#6602=CARTESIAN_POINT ( 'NONE',  ( 135.1060089022256818, -65.16414933467422088, 30.00000000000000000 ) ) ;
#6608=LINE ( 'NONE', #156, #3882 ) ;
#6616=DIRECTION ( 'NONE',  ( 0.000000000000000000, 0.000000000000000000, -1.000000000000000000 ) ) ;
#6629=LINE ( 'NONE', #12444, #1440 ) ;
#6630=DIRECTION ( 'NONE',  ( -1.000000000000000000, 0.000000000000000000, 0.000000000000000000 ) ) ;
#6633=CARTESIAN_POINT ( 'NONE',  ( 134.6444961603440902, -66.11310837778572136, 4.324214274277042414 ) ) ;
#6637=CARTESIAN_POINT ( 'NONE',  ( -110.0000000000000142, 165.0000000000000000, -34.99999999999997868 ) ) ;
#6638=CARTESIAN_POINT ( 'NONE',  ( -109.9999999999983515, 265.0000000000000000, 77.50000000000000000 ) ) ;
#6639=CARTESIAN_POINT ( 'NONE',  ( 141.8714406926367815, -48.70825716237079916, 49.99999999999999289 ) ) ;
#6647=EDGE_CURVE ( 'NONE', #4447, #4182, #16885, .T. ) ;
#6649=VERTEX_POINT ( 'NONE', #10792 ) ;
#6651=PLANE ( 'NONE',  #5840 ) ;
#6653=B_SPLINE_CURVE_WITH_KNOTS ( 'NONE', 3,
 ( #12593, #15685, #11165, #1457, #7893, #1761, #2997, #11064, #8094, #9330, #6278, #7686, #12700, #1666, #4524, #9636, #10958, #13928, #18652, #20173, #12393, #18855, #7996, #12491, #17219, #3200 ),
 .UNSPECIFIED., .F., .F.,
 ( 4, 2, 2, 2, 2, 2, 2, 2, 2, 2, 2, 2, 4 ),
 ( 0.000000000000000000, 0.001429785831555309026, 0.002144678747332965599, 0.002859571663110624992, 0.004289357494665932066, 0.005719143326221240442, 0.007148929157776548818, 0.008578714989331853724, 0.01143828665244240976, 0.01429785831555296580, 0.01572764414710824468, 0.01715742997866355479, 0.02287657330488494789 ),
 .UNSPECIFIED. ) ;
#6671=CARTESIAN_POINT ( 'NONE',  ( 106.9434821670232623, -119.5159909196223111, 40.00000000000000000 ) ) ;
#6678=ORIENTED_EDGE ( 'NONE', *, *, #10648, .F. ) ;
#6682=ORIENTED_EDGE ( 'NONE', *, *, #12825, .T. ) ;
#6688=CARTESIAN_POINT ( 'NONE',  ( -82.57283217324577151, -125.2267376009800444, 5.213532245358446282 ) ) ;
#6689=FACE_OUTER_BOUND ( 'NONE', #17347, .T. ) ;
#6694=CARTESIAN_POINT ( 'NONE',  ( 0.000000000000000000, 0.000000000000000000, -100.0000000000000000 ) ) ;
#6697=CARTESIAN_POINT ( 'NONE',  ( -128.5162560489251860, 45.03435910158038524, -24.76419096631276417 ) ) ;
#6703=FACE_OUTER_BOUND ( 'NONE', #17301, .T. ) ;
#6706=DIRECTION ( 'NONE',  ( -0.9009688679024160374, -0.4338837391175646707, 0.000000000000000000 ) ) ;
#6709=DIRECTION ( 'NONE',  ( -1.000000000000000000, 0.000000000000000000, 0.000000000000000000 ) ) ;
#6714=ORIENTED_EDGE ( 'NONE', *, *, #15135, .T. ) ;
#6715=AXIS2_PLACEMENT_3D ( 'NONE', #3619, #15898, #8110 ) ;
#6716=CARTESIAN_POINT ( 'NONE',  ( 134.1103769904815408, -77.28650662340041322, 36.11580906139592173 ) ) ;
#6720=VERTEX_POINT ( 'NONE', #17250 ) ;
#6727=APPLICATION_CONTEXT ( 'automotive_design' ) ;
#6735=AXIS2_PLACEMENT_3D ( 'NONE', #11523, #11710, #16338 ) ;
#6740=CARTESIAN_POINT ( 'NONE',  ( 87.33261371895460456, -121.9603527571197361, 43.99921538561949319 ) ) ;
#6753=DIRECTION ( 'NONE',  ( -1.000000000000000000, 0.000000000000000000, 0.000000000000000000 ) ) ;
#6758=EDGE_CURVE ( 'NONE', #4372, #17725, #4650, .T. ) ;
#6761=DIRECTION ( 'NONE',  ( -8.294538580027652572E-17, 2.273402209432136919E-16, -1.000000000000000000 ) ) ;
#6765=CARTESIAN_POINT ( 'NONE',  ( 89.19226148815698707, -120.6070458769191163, -5.778503507065541278 ) ) ;
#6766=CARTESIAN_POINT ( 'NONE',  ( 100.7812500000000284, -111.0996833858562809, 39.99999999999999289 ) ) ;
#6771=CARTESIAN_POINT ( 'NONE',  ( -99.66897253883981023, 112.1566004585619964, 43.73620438184401138 ) ) ;
#6778=EDGE_CURVE ( 'NONE', #2503, #573, #19091, .T. ) ;
#6779=DIRECTION ( 'NONE',  ( -1.000000000000000000, 0.000000000000000000, 0.000000000000000000 ) ) ;
#6782=CYLINDRICAL_SURFACE ( 'NONE', #8666, 7.500000000000003553 ) ;
#6784=CARTESIAN_POINT ( 'NONE',  ( -87.54876440220090217, -121.8053786065146511, -4.230840218062975389 ) ) ;
#6789=LINE ( 'NONE', #827, #2952 ) ;
#6793=PLANE ( 'NONE',  #3917 ) ;
#6798=EDGE_LOOP ( 'NONE', ( #969, #9593, #17261, #1817, #16224, #2508 ) ) ;
#6804=CARTESIAN_POINT ( 'NONE',  ( -135.0831964404853238, -65.21150773178311510, 8.539806532481302170 ) ) ;
#6805=DIRECTION ( 'NONE',  ( -1.000000000000000000, 0.000000000000000000, 0.000000000000000000 ) ) ;
#6809=CARTESIAN_POINT ( 'NONE',  ( 133.9275976130212200, -67.55320356804583071, 1.164109098278201193 ) ) ;
#6811=CARTESIAN_POINT ( 'NONE',  ( 99.09522870387660021, -131.8160711339301372, 35.43273011591471544 ) ) ;
#6816=AXIS2_PLACEMENT_3D ( 'NONE', #3692, #8593, #9931 ) ;
#6818=ORIENTED_EDGE ( 'NONE', *, *, #9505, .T. ) ;
#6825=AXIS2_PLACEMENT_3D ( 'NONE', #18617, #18309, #4595 ) ;
#6829=DIRECTION ( 'NONE',  ( 0.9009688679024218105, -0.4338837391175526248, 0.000000000000000000 ) ) ;
#6832=CARTESIAN_POINT ( 'NONE',  ( -95.84941630392641798, 106.2995539097782824, -32.42387014996108263 ) ) ;
#6834=CARTESIAN_POINT ( 'NONE',  ( 134.7188131032333445, -72.93593548660993520, 10.00000000000000178 ) ) ;
#6837=CARTESIAN_POINT ( 'NONE',  ( 84.97262318626000877, -123.6115503146182277, 40.77684021904739353 ) ) ;
#6841=DIRECTION ( 'NONE',  ( 0.000000000000000000, 1.000000000000000000, 0.000000000000000000 ) ) ;
#6842=ORIENTED_EDGE ( 'NONE', *, *, #7746, .T. ) ;
#6847=CARTESIAN_POINT ( 'NONE',  ( -84.32000978867637286, -124.0571233621915610, 39.58209758642278331 ) ) ;
#6851=VERTEX_POINT ( 'NONE', #8227 ) ;
#6852=CARTESIAN_POINT ( 'NONE',  ( 0.000000000000000000, 0.000000000000000000, -40.00000000000000000 ) ) ;
#6853=CARTESIAN_POINT ( 'NONE',  ( 107.5000000000000142, -118.5063289449133492, 0.000000000000000000 ) ) ;
#6855=CARTESIAN_POINT ( 'NONE',  ( 141.8714406926368099, -48.70825716237079916, 49.99999999999999289 ) ) ;
#6860=DIRECTION ( 'NONE',  ( -1.000000000000000000, 0.000000000000000000, 0.000000000000000000 ) ) ;
#6863=ORIENTED_EDGE ( 'NONE', *, *, #11265, .F. ) ;
#6865=LINE ( 'NONE', #16286, #19063 ) ;
#6872=VECTOR ( 'NONE', #16076, 1000.000000000000000 ) ;
#6877=ORIENTED_EDGE ( 'NONE', *, *, #740, .F. ) ;
#6878=DIRECTION ( 'NONE',  ( 0.000000000000000000, 0.000000000000000000, -1.000000000000000000 ) ) ;
#6880=CARTESIAN_POINT ( 'NONE',  ( -97.11506731898813882, -115.6376992562254742, 10.35708075459104371 ) ) ;
#6882=ORIENTED_EDGE ( 'NONE', *, *, #9505, .F. ) ;
#6891=DIRECTION ( 'NONE',  ( -1.000000000000000000, 0.000000000000000000, 0.000000000000000000 ) ) ;
#6899=B_SPLINE_CURVE_WITH_KNOTS ( 'NONE', 3,
 ( #5935, #9084, #4384, #12148, #12354, #2961, #15645, #20037, #10820, #15327, #12456, #6136, #9191, #15221, #18718, #4701, #15434, #16765, #1206, #12560, #1425, #20135, #18409, #4284, #18613, #1525, #17076, #3066, #9299, #3167, #10509, #15543, #13996, #10926, #17592, #16052, #5110, #4913, #3365, #5012, #9903, #1722, #15743, #3667, #18926, #7960, #11339, #8363 ),
 .UNSPECIFIED., .F., .F.,
 ( 4, 2, 2, 2, 2, 2, 2, 2, 2, 2, 2, 2, 2, 2, 2, 2, 2, 2, 2, 2, 2, 2, 2, 4 ),
 ( 0.09493486412272097996, 0.09745231401683318584, 0.09996976391094537784, 0.1050046636991697896, 0.1150744632756185853, 0.1201093630638430110, 0.1226268129579552169, 0.1251442628520674227, 0.1301791626402918900, 0.1326966125344041236, 0.1352140624285163295, 0.1402489622167407690, 0.1452838620049651808, 0.1478013118990773589, 0.1503187617931895925, 0.1553536615814139765, 0.1566123865284700933, 0.1578711114755261824, 0.1603885613696383605, 0.1654234611578627445, 0.1666821861049188613, 0.1679409110519749504, 0.1704583609460871285, 0.1754932607343114848 ),
 .UNSPECIFIED. ) ;
#6900=VERTEX_POINT ( 'NONE', #757 ) ;
#6901=DIRECTION ( 'NONE',  ( 0.000000000000000000, 0.000000000000000000, 1.000000000000000000 ) ) ;
#6902=CARTESIAN_POINT ( 'NONE',  ( -124.4460166144179141, -83.75677717049846649, -9.878997880596227077 ) ) ;
#6906=DIRECTION ( 'NONE',  ( 1.000000000000000000, 0.000000000000000000, 0.000000000000000000 ) ) ;
#6907=CARTESIAN_POINT ( 'NONE',  ( -131.5441688916725980, -89.82688951535520516, 0.05736369426573884045 ) ) ;
#6909=EDGE_CURVE ( 'NONE', #5912, #380, #9970, .T. ) ;
#6910=CARTESIAN_POINT ( 'NONE',  ( 134.7221128596253550, -65.95429948960817512, 4.840168302597956718 ) ) ;
#6912=DIRECTION ( 'NONE',  ( 1.000000000000000000, 0.000000000000000000, 0.000000000000000000 ) ) ;
#6913=AXIS2_PLACEMENT_3D ( 'NONE', #11600, #3829, #4029 ) ;
#6920=ORIENTED_EDGE ( 'NONE', *, *, #19168, .T. ) ;
#6922=ADVANCED_FACE ( 'NONE', ( #8729 ), #8338, .F. ) ;
#6924=CARTESIAN_POINT ( 'NONE',  ( 138.2024300533213932, 89.85329105948596862, 39.99999999999999289 ) ) ;
#6929=ORIENTED_EDGE ( 'NONE', *, *, #4244, .F. ) ;
#6935=LINE ( 'NONE', #13154, #6304 ) ;
#6938=DIRECTION ( 'NONE',  ( 0.000000000000000000, 0.000000000000000000, 1.000000000000000000 ) ) ;
#6944=CARTESIAN_POINT ( 'NONE',  ( 7.500000000000420997, -60.00000000000000000, -105.0000000000000142 ) ) ;
#6945=CARTESIAN_POINT ( 'NONE',  ( -90.16928584620096387, -119.8796671366212365, 46.53660721316358462 ) ) ;
#6950=CARTESIAN_POINT ( 'NONE',  ( 102.1674435767773730, -127.3754966267598405, 1.518799369789654463 ) ) ;
#6958=FACE_OUTER_BOUND ( 'NONE', #10044, .T. ) ;
#6966=AXIS2_PLACEMENT_3D ( 'NONE', #19731, #8689, #3892 ) ;
#6971=CIRCLE ( 'NONE', #2717, 7.500000000000020428 ) ;
#6973=CARTESIAN_POINT ( 'NONE',  ( 56.84754764479240663, -154.7316448359447634, 49.99999999999999289 ) ) ;
#6974=CARTESIAN_POINT ( 'NONE',  ( -95.93567628221582311, -116.0760901523938315, 9.548040410739892181 ) ) ;
#6987=ADVANCED_FACE ( 'NONE', ( #11176 ), #15695, .F. ) ;
#6989=DIRECTION ( 'NONE',  ( -0.2225209339563047894, -0.9749279121818258398, 0.000000000000000000 ) ) ;
#6990=VECTOR ( 'NONE', #5174, 1000.000000000000000 ) ;
#6992=EDGE_LOOP ( 'NONE', ( #8096, #5554, #16507, #17840 ) ) ;
#6993=EDGE_CURVE ( 'NONE', #2271, #3721, #10833, .T. ) ;
#6996=CARTESIAN_POINT ( 'NONE',  ( -122.8001410695374602, -86.14014948502067170, -10.00000000000000178 ) ) ;
#6997=CARTESIAN_POINT ( 'NONE',  ( 0.000000000000000000, 0.000000000000000000, -10.00000000000000178 ) ) ;
#7003=CARTESIAN_POINT ( 'NONE',  ( -122.8001410695374744, -86.14014948502068592, -1.214306433183764966E-14 ) ) ;
#7005=CARTESIAN_POINT ( 'NONE',  ( 134.6956030146747025, -73.12307453597284734, 8.498119811773092280 ) ) ;
#7006=AXIS2_PLACEMENT_3D ( 'NONE', #12310, #10369, #16827 ) ;
#7013=EDGE_LOOP ( 'NONE', ( #11778, #20068, #4726, #14705 ) ) ;
#7014=EDGE_LOOP ( 'NONE', ( #6554, #20195, #15100, #10720 ) ) ;
#7015=CIRCLE ( 'NONE', #17486, 9.999999999999994671 ) ;
#7020=CARTESIAN_POINT ( 'NONE',  ( 0.000000000000000000, 164.0736214083062805, 49.99999999999999289 ) ) ;
#7021=FACE_BOUND ( 'NONE', #2659, .T. ) ;
#7031=EDGE_CURVE ( 'NONE', #9870, #11160, #2818, .T. ) ;
#7036=DIRECTION ( 'NONE',  ( 0.000000000000000000, 0.000000000000000000, 1.000000000000000000 ) ) ;
#7044=ORIENTED_EDGE ( 'NONE', *, *, #10414, .F. ) ;
#7050=LINE ( 'NONE', #11643, #12905 ) ;
#7051=CIRCLE ( 'NONE', #18478, 7.500000000000007994 ) ;
#7054=CARTESIAN_POINT ( 'NONE',  ( 98.70372244599823830, -132.3513910121201604, 5.227003128891625217 ) ) ;
#7058=ORIENTED_EDGE ( 'NONE', *, *, #14021, .T. ) ;
#7061=CARTESIAN_POINT ( 'NONE',  ( 87.79934266039369106, -121.6207432329495504, -4.446207472610150369 ) ) ;
#7063=EDGE_CURVE ( 'NONE', #4062, #11036, #1573, .T. ) ;
#7065=DIRECTION ( 'NONE',  ( 0.9749279121818257288, -0.2225209339563047062, 0.000000000000000000 ) ) ;
#7068=CIRCLE ( 'NONE', #18496, 32.50000000000000000 ) ;
#7073=DIRECTION ( 'NONE',  ( 0.000000000000000000, 0.000000000000000000, 1.000000000000000000 ) ) ;
#7074=ORIENTED_EDGE ( 'NONE', *, *, #19168, .F. ) ;
#7075=CARTESIAN_POINT ( 'NONE',  ( 96.21889527877688408, -115.1753595937449433, 4.451389559091587955 ) ) ;
#7076=CARTESIAN_POINT ( 'NONE',  ( -103.5930306438084472, -125.1526588151300956, 0.7897485457623537597 ) ) ;
#7077=VECTOR ( 'NONE', #183, 1000.000000000000000 ) ;
#7078=CARTESIAN_POINT ( 'NONE',  ( -82.53664710575304753, -125.2505858294166927, 5.373891644490333519 ) ) ;
#7080=CLOSED_SHELL ( 'NONE', ( #19911, #18276, #7955, #15126, #5905, #10987, #5413, #8958, #6396, #10381, #18616, #8105, #14374, #12330, #14108, #4137, #2643, #17443, #3179, #9246, #9891, #18946, #11121, #13316, #10336, #12752, #18272, #8324, #3767, #8241, #13274, #11108, #19742, #4801, #5588, #2898, #16755, #3303, #14780, #15621, #8258, #4104, #15636, #1339, #6268, #17265, #19729, #15476, #7612, #4236, #8159, #19163, #1220, #5499, #13495, #1914, #2760, #2919, #18797, #415, #17924, #8112, #11137, #15991, #19004, #11878, #18733, #16665, #7576, #11281, #12592, #16100, #4655, #7229, #13344, #20140, #11749, #10262, #6987, #5531, #620, #3714, #2139, #871, #16161, #20128, #18288, #7172, #3740, #18660, #654, #13110, #5729, #4107, #13411, #17861, #14515, #4015, #18286, #1038, #12229, #13009, #6922, #1991, #15749, #8163, #16361, #17255, #10228, #3552, #17537, #15844, #19245, #6302, #4390, #13733, #8726, #11481, #12452, #5422, #18655, #15158, #10614, #7616, #13206, #15536, #15516 ) ) ;
#7082=CARTESIAN_POINT ( 'NONE',  ( -82.03124999999998579, -125.5821405433014064, 49.99999999999999289 ) ) ;
#7086=ORIENTED_EDGE ( 'NONE', *, *, #19059, .F. ) ;
#7089=CARTESIAN_POINT ( 'NONE',  ( -123.8492616149702741, -72.31991210363503342, 10.00000000000000178 ) ) ;
#7097=CIRCLE ( 'NONE', #18535, 140.0000000000000000 ) ;
#7107=EDGE_CURVE ( 'NONE', #6494, #12362, #10506, .T. ) ;
#7108=VERTEX_POINT ( 'NONE', #16495 ) ;
#7112=ORIENTED_EDGE ( 'NONE', *, *, #5237, .T. ) ;
#7115=ORIENTED_EDGE ( 'NONE', *, *, #7031, .F. ) ;
#7118=EDGE_CURVE ( 'NONE', #18229, #16974, #5321, .T. ) ;
#7121=CARTESIAN_POINT ( 'NONE',  ( 0.000000000000000000, 0.000000000000000000, -100.0000000000000000 ) ) ;
#7123=CARTESIAN_POINT ( 'NONE',  ( -42.50000000000000000, 5.204748896376250896E-15, -49.99999999999999289 ) ) ;
#7125=CIRCLE ( 'NONE', #8100, 77.50000000000000000 ) ;
#7130=CARTESIAN_POINT ( 'NONE',  ( -7.499999999999583444, -60.00000000000000000, -105.0000000000000142 ) ) ;
#7133=CARTESIAN_POINT ( 'NONE',  ( -134.7652707650784407, -31.41120252075685215, -19.73219286542039441 ) ) ;
#7135=ORIENTED_EDGE ( 'NONE', *, *, #12837, .T. ) ;
#7136=DIRECTION ( 'NONE',  ( -1.000000000000000000, 1.224646799147352961E-16, 0.000000000000000000 ) ) ;
#7138=ORIENTED_EDGE ( 'NONE', *, *, #19139, .F. ) ;
#7141=ORIENTED_EDGE ( 'NONE', *, *, #13616, .F. ) ;
#7145=ORIENTED_EDGE ( 'NONE', *, *, #19893, .F. ) ;
#7150=CARTESIAN_POINT ( 'NONE',  ( -99.70874217756772850, -112.0725815587889969, 50.00000000000000000 ) ) ;
#7151=DIRECTION ( 'NONE',  ( 0.000000000000000000, 0.000000000000000000, 1.000000000000000000 ) ) ;
#7154=CARTESIAN_POINT ( 'NONE',  ( -134.7540465048386977, -65.88919983460813512, 34.98379477817776007 ) ) ;
#7171=AXIS2_PLACEMENT_3D ( 'NONE', #11583, #14753, #14847 ) ;
#7172=ADVANCED_FACE ( 'NONE', ( #7183, #11580 ), #9844, .T. ) ;
#7176=CARTESIAN_POINT ( 'NONE',  ( 106.6880305650188205, 105.4403344747995988, 39.99999999999999289 ) ) ;
#7179=CARTESIAN_POINT ( 'NONE',  ( 98.08520584363758132, -113.5061255252653751, 1.878459693818897991 ) ) ;
#7183=FACE_OUTER_BOUND ( 'NONE', #9301, .T. ) ;
#7184=DIRECTION ( 'NONE',  ( 1.000000000000000000, 0.000000000000000000, 0.000000000000000000 ) ) ;
#7192=ORIENTED_EDGE ( 'NONE', *, *, #9355, .F. ) ;
#7197=VECTOR ( 'NONE', #19845, 1000.000000000000000 ) ;
#7199=DIRECTION ( 'NONE',  ( 1.613511099790691498E-16, -1.000000000000000000, 0.000000000000000000 ) ) ;
#7204=CARTESIAN_POINT ( 'NONE',  ( 134.4924637689107669, -74.66092226661579900, 6.056214776001138667 ) ) ;
#7207=CARTESIAN_POINT ( 'NONE',  ( -107.5000000000000000, -1.734524432274993541E-14, 40.00000000000000000 ) ) ;
#7216=FACE_BOUND ( 'NONE', #4361, .T. ) ;
#7220=CARTESIAN_POINT ( 'NONE',  ( -47.22802745636877120, -134.7565053399285091, 39.99999999999999289 ) ) ;
#7227=AXIS2_PLACEMENT_3D ( 'NONE', #12915, #6391, #16098 ) ;
#7229=ADVANCED_FACE ( 'NONE', ( #2188 ), #14559, .F. ) ;
#7233=EDGE_CURVE ( 'NONE', #7267, #19595, #8582, .T. ) ;
#7234=DIRECTION ( 'NONE',  ( -1.000000000000000000, -5.551115123125777969E-15, 0.000000000000000000 ) ) ;
#7236=EDGE_LOOP ( 'NONE', ( #13409, #15781, #6472, #12023 ) ) ;
#7242=CARTESIAN_POINT ( 'NONE',  ( -82.22461745850685588, -125.4556360547412197, 32.88769404282036390 ) ) ;
#7246=CARTESIAN_POINT ( 'NONE',  ( -133.3341203894445357, -68.71829099011286246, 40.67712301011120246 ) ) ;
#7249=CARTESIAN_POINT ( 'NONE',  ( 75.91068486117727332, -120.9436655338208340, 39.99999999999999289 ) ) ;
#7253=EDGE_CURVE ( 'NONE', #13254, #18093, #13788, .T. ) ;
#7254=CARTESIAN_POINT ( 'NONE',  ( -134.6687524777004796, -73.33058021821595673, 31.91433120627149123 ) ) ;
#7262=CARTESIAN_POINT ( 'NONE',  ( -97.49999999993794120, -115.4778303847070902, 29.92289092923461524 ) ) ;
#7267=VERTEX_POINT ( 'NONE', #12062 ) ;
#7270=CARTESIAN_POINT ( 'NONE',  ( -136.4994460260996902, -31.11111111111111072, -9.999999999999985789 ) ) ;
#7287=AXIS2_PLACEMENT_3D ( 'NONE', #5704, #10592, #13560 ) ;
#7289=CARTESIAN_POINT ( 'NONE',  ( -110.0000000000000142, 265.0000000000000000, 5.000000000000000888 ) ) ;
#7295=CYLINDRICAL_SURFACE ( 'NONE', #19263, 9.999999999999994671 ) ;
#7296=CARTESIAN_POINT ( 'NONE',  ( -130.0656023054207822, -74.72982709287477121, -6.442063508531142624 ) ) ;
#7297=CARTESIAN_POINT ( 'NONE',  ( 122.8001410695374460, -86.14014948502070013, 8.673617379884035472E-15 ) ) ;
#7301=DIRECTION ( 'NONE',  ( -0.000000000000000000, -0.000000000000000000, 1.000000000000000000 ) ) ;
#7306=ORIENTED_EDGE ( 'NONE', *, *, #16109, .F. ) ;
#7314=CARTESIAN_POINT ( 'NONE',  ( 0.000000000000000000, 0.000000000000000000, 49.99999999999999289 ) ) ;
#7317=CARTESIAN_POINT ( 'NONE',  ( 130.9868171408399746, -91.88282611735537841, 40.00000000000000000 ) ) ;
#7319=CARTESIAN_POINT ( 'NONE',  ( -131.4992782843381462, -89.99675518205303604, 0.04849131325310787610 ) ) ;
#7321=CARTESIAN_POINT ( 'NONE',  ( 127.6186898578139761, -78.88112642940112096, 40.77662057728262113 ) ) ;
#7326=CARTESIAN_POINT ( 'NONE',  ( -176.7850001792985211, -188.8278678429259685, 32.32637774726087798 ) ) ;
#7328=ORIENTED_EDGE ( 'NONE', *, *, #10236, .T. ) ;
#7332=VERTEX_POINT ( 'NONE', #8900 ) ;
#7334=DIRECTION ( 'NONE',  ( -1.000000000000000000, 0.000000000000000000, 0.000000000000000000 ) ) ;
#7342=VERTEX_POINT ( 'NONE', #16788 ) ;
#7345=CYLINDRICAL_SURFACE ( 'NONE', #18459, 7.500000000000007105 ) ;
#7347=CARTESIAN_POINT ( 'NONE',  ( 71.18887634719571622, -147.8252249328912740, 49.99999999999999289 ) ) ;
#7348=CARTESIAN_POINT ( 'NONE',  ( -71.18887634719365565, -147.8252249328922687, 39.99999999999999289 ) ) ;
#7352=EDGE_CURVE ( 'NONE', #12362, #6494, #5977, .T. ) ;
#7353=CYLINDRICAL_SURFACE ( 'NONE', #12013, 140.0000000000000284 ) ;
#7355=ORIENTED_EDGE ( 'NONE', *, *, #1328, .F. ) ;
#7357=CARTESIAN_POINT ( 'NONE',  ( -107.4999999999999858, -118.5063289449133777, 40.00000000000000000 ) ) ;
#7363=VERTEX_POINT ( 'NONE', #18526 ) ;
#7364=CARTESIAN_POINT ( 'NONE',  ( 96.81625497255032542, -114.6298681929799557, 3.428784747764392460 ) ) ;
#7368=CARTESIAN_POINT ( 'NONE',  ( -109.9999999999983515, 275.0000000000000000, 77.50000000000000000 ) ) ;
#7372=FACE_OUTER_BOUND ( 'NONE', #3399, .T. ) ;
#7380=ORIENTED_EDGE ( 'NONE', *, *, #13442, .F. ) ;
#7383=EDGE_CURVE ( 'NONE', #6649, #14876, #15561, .T. ) ;
#7384=DIRECTION ( 'NONE',  ( 1.000000000000000000, 0.000000000000000000, 0.000000000000000000 ) ) ;
#7393=DIRECTION ( 'NONE',  ( 0.000000000000000000, 0.000000000000000000, -1.000000000000000000 ) ) ;
#7394=CARTESIAN_POINT ( 'NONE',  ( -131.4393841463108288, -72.38802639018405216, 2.524901613696201697 ) ) ;
#7395=CARTESIAN_POINT ( 'NONE',  ( 131.2164711380734730, -72.78471332658568826, 2.208503663874919365 ) ) ;
#7396=CYLINDRICAL_SURFACE ( 'NONE', #358, 10.00000000000000888 ) ;
#7398=CARTESIAN_POINT ( 'NONE',  ( -60.00000000000000000, -2.094888803305880013E-13, -105.0000000000000142 ) ) ;
#7410=CARTESIAN_POINT ( 'NONE',  ( -110.0000000000000142, 1.347111479062088839E-14, -9.999999999999994671 ) ) ;
#7411=CARTESIAN_POINT ( 'NONE',  ( 15.91767397667354800, 164.0736214083062805, 49.99999999999999289 ) ) ;
#7418=CARTESIAN_POINT ( 'NONE',  ( -82.11169388575343930, 112.6076301679229772, -16.15456432045361979 ) ) ;
#7423=CIRCLE ( 'NONE', #18206, 7.500000000000007105 ) ;
#7428=DIRECTION ( 'NONE',  ( 0.000000000000000000, 0.000000000000000000, 1.000000000000000000 ) ) ;
#7433=EDGE_LOOP ( 'NONE', ( #13634, #19564, #128, #14785 ) ) ;
#7437=DIRECTION ( 'NONE',  ( -0.000000000000000000, -1.000000000000000000, -0.000000000000000000 ) ) ;
#7438=EDGE_LOOP ( 'NONE', ( #310, #7787, #5093, #15364 ) ) ;
#7442=CARTESIAN_POINT ( 'NONE',  ( -88.53631457789035153, 115.2621388628904526, -28.80465452976635632 ) ) ;
#7443=CARTESIAN_POINT ( 'NONE',  ( -163.5019688434124419, -20.99123081650240863, 49.99999999999999289 ) ) ;
#7446=CYLINDRICAL_SURFACE ( 'NONE', #13381, 15.91767397667354800 ) ;
#7449=ORIENTED_EDGE ( 'NONE', *, *, #18275, .T. ) ;
#7450=AXIS2_PLACEMENT_3D ( 'NONE', #8081, #12581, #6265 ) ;
#7456=CARTESIAN_POINT ( 'NONE',  ( -82.03125000005908873, -125.5821405432628382, 30.74521087840624034 ) ) ;
#7462=CARTESIAN_POINT ( 'NONE',  ( 99.98863955314980956, -130.5690324404832268, 3.390001990510095986 ) ) ;
#7464=VECTOR ( 'NONE', #14960, 1000.000000000000114 ) ;
#7465=VECTOR ( 'NONE', #12192, 1000.000000000000000 ) ;
#7467=CARTESIAN_POINT ( 'NONE',  ( -137.2265357449624616, -24.54992354075934458, -16.95325888733908215 ) ) ;
#7472=CARTESIAN_POINT ( 'NONE',  ( 95.77047472624727220, -116.1200526047208967, 30.77282038149522236 ) ) ;
#7483=ORIENTED_EDGE ( 'NONE', *, *, #84, .F. ) ;
#7485=ORIENTED_EDGE ( 'NONE', *, *, #5783, .T. ) ;
#7487=CARTESIAN_POINT ( 'NONE',  ( 134.7188131032333445, -72.93593548660993520, 10.00000000000000178 ) ) ;
#7491=DIRECTION ( 'NONE',  ( 0.8186676071302493307, -0.5742676632334713371, 0.000000000000000000 ) ) ;
#7492=CARTESIAN_POINT ( 'NONE',  ( 107.5000000000000000, 1.734524432274993541E-14, 30.00000000000000000 ) ) ;
#7495=VERTEX_POINT ( 'NONE', #7880 ) ;
#7498=CARTESIAN_POINT ( 'NONE',  ( 134.0015816819113184, -77.97298368086231335, 3.467253640805495252 ) ) ;
#7501=FACE_OUTER_BOUND ( 'NONE', #7236, .T. ) ;
#7503=DIRECTION ( 'NONE',  ( -0.000000000000000000, -0.000000000000000000, 1.000000000000000000 ) ) ;
#7505=EDGE_CURVE ( 'NONE', #9853, #5389, #206, .T. ) ;
#7514=VERTEX_POINT ( 'NONE', #2061 ) ;
#7516=LINE ( 'NONE', #6406, #8481 ) ;
#7518=CARTESIAN_POINT ( 'NONE',  ( -78.37722339831623231, 116.0043570404596522, -9.999999999999984013 ) ) ;
#7527=ORIENTED_EDGE ( 'NONE', *, *, #3413, .F. ) ;
#7543=CARTESIAN_POINT ( 'NONE',  ( -29.99999999999887379, 275.0000000000000000, 4.999999999999158007 ) ) ;
#7547=DIRECTION ( 'NONE',  ( 1.000000000000000000, 0.000000000000000000, 0.000000000000000000 ) ) ;
#7548=VECTOR ( 'NONE', #14622, 1000.000000000000000 ) ;
#7553=B_SPLINE_CURVE_WITH_KNOTS ( 'NONE', 3,
 ( #134, #18866, #38, #4852, #4746, #18765, #3209, #19167, #17337, #11383, #17539, #10970, #14453, #15993, #11280, #17229, #9447, #3414, #440, #1981, #9644, #3313, #6289, #19073, #8207, #14252 ),
 .UNSPECIFIED., .F., .F.,
 ( 4, 2, 2, 2, 2, 2, 2, 2, 2, 2, 2, 2, 4 ),
 ( 6.938893903907228378E-18, 0.005933429007670090738, 0.01186685801534017454, 0.02373371603068033520, 0.02966714503835042246, 0.03560057404602051667, 0.04746743206136066345, 0.05933429007670083105, 0.07120114809204097783, 0.07416786259587601626, 0.07713457709971105469, 0.08306800610738104829, 0.09493486412272097996 ),
 .UNSPECIFIED. ) ;
#7554=CARTESIAN_POINT ( 'NONE',  ( 82.03125000000004263, -125.5821405433013780, 30.00000000000000000 ) ) ;
#7556=VERTEX_POINT ( 'NONE', #19441 ) ;
#7561=CARTESIAN_POINT ( 'NONE',  ( -144.0985391606959354, 40.21647770819863865, -15.98578004590384438 ) ) ;
#7562=DIRECTION ( 'NONE',  ( 1.000000000000000000, 0.000000000000000000, 0.000000000000000000 ) ) ;
#7564=CARTESIAN_POINT ( 'NONE',  ( 96.95682486763449504, -115.7027609143983398, 10.38738059575018724 ) ) ;
#7567=LINE ( 'NONE', #18324, #7197 ) ;
#7570=DIRECTION ( 'NONE',  ( 1.000000000000000000, 0.000000000000000000, -0.000000000000000000 ) ) ;
#7571=CARTESIAN_POINT ( 'NONE',  ( 100.4426743476961974, -129.9257371803372791, 37.11542010922146062 ) ) ;
#7572=ORIENTED_EDGE ( 'NONE', *, *, #17307, .T. ) ;
#7573=CARTESIAN_POINT ( 'NONE',  ( -110.0000000000000142, 275.0000000000000000, -82.50000000000001421 ) ) ;
#7575=ORIENTED_EDGE ( 'NONE', *, *, #5367, .F. ) ;
#7576=ADVANCED_FACE ( 'NONE', ( #5134 ), #14726, .F. ) ;
#7580=AXIS2_PLACEMENT_3D ( 'NONE', #13198, #2085, #8310 ) ;
#7588=CARTESIAN_POINT ( 'NONE',  ( -85.53020504959707182, -140.9188050298390067, 49.99999999999999289 ) ) ;
#7589=CARTESIAN_POINT ( 'NONE',  ( 0.000000000000000000, 0.000000000000000000, -9.999999999999994671 ) ) ;
#7590=ORIENTED_EDGE ( 'NONE', *, *, #9760, .T. ) ;
#7592=DIRECTION ( 'NONE',  ( -0.2225209339563195554, 0.9749279121818223981, 0.000000000000000000 ) ) ;
#7594=CARTESIAN_POINT ( 'NONE',  ( 134.3546152455197955, -75.63949198389357775, 5.121906984077789993 ) ) ;
#7595=AXIS2_PLACEMENT_3D ( 'NONE', #6575, #14537, #19056 ) ;
#7598=DIRECTION ( 'NONE',  ( 0.000000000000000000, 0.000000000000000000, -1.000000000000000000 ) ) ;
#7599=CARTESIAN_POINT ( 'NONE',  ( -133.0181789769753777, -69.32831038615765351, 41.48694412335748183 ) ) ;
#7600=VERTEX_POINT ( 'NONE', #19247 ) ;
#7601=CYLINDRICAL_SURFACE ( 'NONE', #409, 99.99999999999997158 ) ;
#7602=CIRCLE ( 'NONE', #7287, 160.0000000000000284 ) ;
#7607=ORIENTED_EDGE ( 'NONE', *, *, #19651, .T. ) ;
#7612=ADVANCED_FACE ( 'NONE', ( #19340 ), #11358, .F. ) ;
#7616=ADVANCED_FACE ( 'NONE', ( #16373 ), #10127, .F. ) ;
#7620=DIRECTION ( 'NONE',  ( -0.000000000000000000, -0.000000000000000000, -1.000000000000000000 ) ) ;
#7623=AXIS2_PLACEMENT_3D ( 'NONE', #16153, #14902, #7136 ) ;
#7624=CARTESIAN_POINT ( 'NONE',  ( 124.9958490023956301, -82.94424249022426920, 40.96431696885655782 ) ) ;
#7633=CARTESIAN_POINT ( 'NONE',  ( -97.49999999999997158, -200.0000000000000000, 30.00000000000000000 ) ) ;
#7635=ORIENTED_EDGE ( 'NONE', *, *, #6132, .F. ) ;
#7636=CARTESIAN_POINT ( 'NONE',  ( 135.1060089022256818, -65.16414933467422088, 10.00000000000000355 ) ) ;
#7638=( LENGTH_UNIT ( ) NAMED_UNIT ( * ) SI_UNIT ( .MILLI., .METRE. ) );
#7642=EDGE_CURVE ( 'NONE', #13254, #2847, #18176, .T. ) ;
#7649=CARTESIAN_POINT ( 'NONE',  ( -107.5000000000000000, -1.734524432274993541E-14, 30.00000000000000000 ) ) ;
#7653=CARTESIAN_POINT ( 'NONE',  ( -131.4993367897275789, -89.99660315853896009, 39.95156676386486083 ) ) ;
#7654=FACE_OUTER_BOUND ( 'NONE', #11396, .T. ) ;
#7661=EDGE_CURVE ( 'NONE', #19189, #1562, #2022, .T. ) ;
#7663=VECTOR ( 'NONE', #18821, 1000.000000000000000 ) ;
#7666=FACE_OUTER_BOUND ( 'NONE', #10804, .T. ) ;
#7669=CARTESIAN_POINT ( 'NONE',  ( 82.03125000000001421, -125.5821405433014064, 9.999999999999991118 ) ) ;
#7675=AXIS2_PLACEMENT_3D ( 'NONE', #14363, #13015, #17544 ) ;
#7676=CARTESIAN_POINT ( 'NONE',  ( 118.3534152657848608, 114.7431683447366595, 49.99999999999999289 ) ) ;
#7677=FACE_BOUND ( 'NONE', #5725, .T. ) ;
#7678=CARTESIAN_POINT ( 'NONE',  ( 99.45845524092791834, -131.3126558323551478, 35.94668960775785393 ) ) ;
#7686=CARTESIAN_POINT ( 'NONE',  ( -99.09522870387660021, -131.8160711339301656, 4.567269884085281006 ) ) ;
#7689=DIRECTION ( 'NONE',  ( -0.000000000000000000, -0.000000000000000000, -1.000000000000000000 ) ) ;
#7690=DIRECTION ( 'NONE',  ( 0.000000000000000000, 0.000000000000000000, -1.000000000000000000 ) ) ;
#7691=CARTESIAN_POINT ( 'NONE',  ( -86.28560748592356333, -122.6989046848843969, 42.70417760891430703 ) ) ;
#7693=CARTESIAN_POINT ( 'NONE',  ( -72.91900756452172061, 131.0832496385607158, -10.00000000000000178 ) ) ;
#7697=CARTESIAN_POINT ( 'NONE',  ( -133.2712073793125001, -68.96827650305596080, 10.00000000000000888 ) ) ;
#7698=CARTESIAN_POINT ( 'NONE',  ( 126.6625757374826549, -80.35588318643314665, -9.093145544296387328 ) ) ;
#7702=CARTESIAN_POINT ( 'NONE',  ( -133.5474595738625680, -68.30173510457200337, 40.05649235983763390 ) ) ;
#7703=EDGE_LOOP ( 'NONE', ( #9682, #497 ) ) ;
#7706=ORIENTED_EDGE ( 'NONE', *, *, #13108, .F. ) ;
#7708=VERTEX_POINT ( 'NONE', #19107 ) ;
#7720=EDGE_CURVE ( 'NONE', #7514, #7708, #20032, .T. ) ;
#7726=AXIS2_PLACEMENT_3D ( 'NONE', #8503, #16486, #16582 ) ;
#7727=CARTESIAN_POINT ( 'NONE',  ( 133.9967726966432338, -77.99266392030685324, 36.52075283398300343 ) ) ;
#7745=DIRECTION ( 'NONE',  ( 1.000000000000000000, 0.000000000000000000, 0.000000000000000000 ) ) ;
#7746=EDGE_CURVE ( 'NONE', #5045, #5530, #753, .T. ) ;
#7753=CARTESIAN_POINT ( 'NONE',  ( 0.000000000000000000, 0.000000000000000000, -10.00000000000000178 ) ) ;
#7755=CARTESIAN_POINT ( 'NONE',  ( 159.9599531637113330, -36.50981547336952104, 39.99999999999999289 ) ) ;
#7765=DIRECTION ( 'NONE',  ( 1.000000000000000000, 0.000000000000000000, 0.000000000000000000 ) ) ;
#7766=VERTEX_POINT ( 'NONE', #8647 ) ;
#7767=CARTESIAN_POINT ( 'NONE',  ( -111.9753657172487635, 86.11583021959165762, -34.99999999999998579 ) ) ;
#7768=DIRECTION ( 'NONE',  ( -0.000000000000000000, -0.000000000000000000, -1.000000000000000000 ) ) ;
#7780=DIRECTION ( 'NONE',  ( 0.9749279121818227312, 0.2225209339563182231, -0.000000000000000000 ) ) ;
#7781=CARTESIAN_POINT ( 'NONE',  ( 96.67218534449422407, -115.8154871359606375, 29.72277444615395936 ) ) ;
#7782=ORIENTED_EDGE ( 'NONE', *, *, #3853, .T. ) ;
#7784=CARTESIAN_POINT ( 'NONE',  ( 130.9868171408399462, -91.88282611735539263, 0.000000000000000000 ) ) ;
#7787=ORIENTED_EDGE ( 'NONE', *, *, #14261, .T. ) ;
#7792=AXIS2_PLACEMENT_3D ( 'NONE', #2492, #10256, #7199 ) ;
#7794=AXIS2_PLACEMENT_3D ( 'NONE', #2957, #19623, #3163 ) ;
#7803=CARTESIAN_POINT ( 'NONE',  ( -96.05830942202625522, -116.0381168402466159, 30.26647072828682639 ) ) ;
#7805=CARTESIAN_POINT ( 'NONE',  ( 87.10655032386927132, -147.8252249328912740, 39.99999999999999289 ) ) ;
#7806=FACE_OUTER_BOUND ( 'NONE', #5385, .T. ) ;
#7807=FACE_OUTER_BOUND ( 'NONE', #9677, .T. ) ;
#7810=CARTESIAN_POINT ( 'NONE',  ( -109.9999999999983515, 275.0000000000000000, 85.00000000000001421 ) ) ;
#7811=CARTESIAN_POINT ( 'NONE',  ( -132.9666886943602719, -83.66363014847074453, 38.85988273695094364 ) ) ;
#7814=CARTESIAN_POINT ( 'NONE',  ( 42.50000000000000000, 0.000000000000000000, -100.0000000000000000 ) ) ;
#7815=ORIENTED_EDGE ( 'NONE', *, *, #14835, .T. ) ;
#7824=CARTESIAN_POINT ( 'NONE',  ( -109.9999999999874376, 73.61623156955475622, -29.99999999999998579 ) ) ;
#7826=DIRECTION ( 'NONE',  ( 0.000000000000000000, 0.000000000000000000, 1.000000000000000000 ) ) ;
#7830=CARTESIAN_POINT ( 'NONE',  ( 132.3052566686612863, -70.67971788940297984, 43.04150566780438680 ) ) ;
#7833=ORIENTED_EDGE ( 'NONE', *, *, #15079, .F. ) ;
#7840=CARTESIAN_POINT ( 'NONE',  ( -100.4560359297607874, -129.9019447003570349, 37.10626013476207419 ) ) ;
#7842=CIRCLE ( 'NONE', #2312, 7.500000000000006217 ) ;
#7843=LINE ( 'NONE', #4900, #13176 ) ;
#7844=FACE_OUTER_BOUND ( 'NONE', #14129, .T. ) ;
#7854=EDGE_CURVE ( 'NONE', #6551, #12474, #16333, .T. ) ;
#7859=DIRECTION ( 'NONE',  ( 0.000000000000000000, 0.000000000000000000, 1.000000000000000000 ) ) ;
#7867=ORIENTED_EDGE ( 'NONE', *, *, #19137, .F. ) ;
#7868=CARTESIAN_POINT ( 'NONE',  ( -120.9637972807140045, 75.12262024236758862, -33.48191611480011431 ) ) ;
#7871=CARTESIAN_POINT ( 'NONE',  ( 82.07017599500315441, -125.5567397147592743, 8.511632757311264896 ) ) ;
#7876=EDGE_CURVE ( 'NONE', #17725, #4372, #16434, .T. ) ;
#7878=CARTESIAN_POINT ( 'NONE',  ( 0.000000000000000000, 0.000000000000000000, 49.99999999999999289 ) ) ;
#7880=CARTESIAN_POINT ( 'NONE',  ( -110.0000000000000142, 275.0000000000000000, -29.99999999999998224 ) ) ;
#7883=CARTESIAN_POINT ( 'NONE',  ( 98.30983243222797796, -132.8827373471760893, 33.95839073212757597 ) ) ;
#7884=ORIENTED_EDGE ( 'NONE', *, *, #9396, .T. ) ;
#7885=CARTESIAN_POINT ( 'NONE',  ( -110.0000000000000142, 265.0000000000000000, -75.00000000000000000 ) ) ;
#7886=CARTESIAN_POINT ( 'NONE',  ( -70.08028827194087285, 132.6226048388235199, 2.306676233856181479 ) ) ;
#7888=ORIENTED_EDGE ( 'NONE', *, *, #2753, .T. ) ;
#7893=CARTESIAN_POINT ( 'NONE',  ( -97.67667160654316660, -133.7228621772585484, 8.114239421803903340 ) ) ;
#7895=ORIENTED_EDGE ( 'NONE', *, *, #13573, .F. ) ;
#7896=CARTESIAN_POINT ( 'NONE',  ( 128.2779226595531270, 102.2982297021113141, 49.99999999999999289 ) ) ;
#7897=CARTESIAN_POINT ( 'NONE',  ( -110.0000000000000142, 265.0000000000000000, 5.000000000000000888 ) ) ;
#7899=CARTESIAN_POINT ( 'NONE',  ( -89.41054993673267859, -120.4453604907586310, 45.95706278337525674 ) ) ;
#7903=CARTESIAN_POINT ( 'NONE',  ( -98.63291732527035549, -113.0135401039851786, -9.876607713649601550 ) ) ;
#7904=DIRECTION ( 'NONE',  ( 1.613511099790691498E-16, -1.000000000000000000, 0.000000000000000000 ) ) ;
#7907=CARTESIAN_POINT ( 'NONE',  ( -131.9259051260646629, -88.29481989230392003, 39.77911086439604560 ) ) ;
#7919=CARTESIAN_POINT ( 'NONE',  ( -47.22802745636877120, -134.7565053399285091, 39.99999999999999289 ) ) ;
#7928=EDGE_CURVE ( 'NONE', #16974, #4062, #13826, .T. ) ;
#7930=CARTESIAN_POINT ( 'NONE',  ( 134.6114153021046320, -66.18050771012664768, 35.86948590222475985 ) ) ;
#7931=CARTESIAN_POINT ( 'NONE',  ( 133.3649390995069268, -81.63041515106810664, 38.20349535801842933 ) ) ;
#7936=ORIENTED_EDGE ( 'NONE', *, *, #17235, .F. ) ;
#7937=ORIENTED_EDGE ( 'NONE', *, *, #18680, .T. ) ;
#7942=CARTESIAN_POINT ( 'NONE',  ( -97.67856431661350314, -133.7203759155860894, 31.89566238906889240 ) ) ;
#7948=LINE ( 'NONE', #12551, #19746 ) ;
#7953=AXIS2_PLACEMENT_3D ( 'NONE', #10417, #15128, #8984 ) ;
#7955=ADVANCED_FACE ( 'NONE', ( #12290 ), #18759, .F. ) ;
#7960=CARTESIAN_POINT ( 'NONE',  ( -77.07195518394449607, 116.8771345694330108, -6.980692854872754260 ) ) ;
#7961=EDGE_LOOP ( 'NONE', ( #19130, #19931, #15839, #9361 ) ) ;
#7963=VECTOR ( 'NONE', #17502, 1000.000000000000000 ) ;
#7965=VERTEX_POINT ( 'NONE', #4528 ) ;
#7969=CARTESIAN_POINT ( 'NONE',  ( -125.8454112683333506, 69.15288340776045573, -31.78671230953092319 ) ) ;
#7970=DIRECTION ( 'NONE',  ( 0.000000000000000000, 0.000000000000000000, 1.000000000000000000 ) ) ;
#7978=CARTESIAN_POINT ( 'NONE',  ( -170.2125097089225960, -199.3942630591407692, 0.000000000000000000 ) ) ;
#7982=CARTESIAN_POINT ( 'NONE',  ( -166.7850001792984926, -200.0000000000000284, 0.000000000000000000 ) ) ;
#7985=ORIENTED_EDGE ( 'NONE', *, *, #9851, .T. ) ;
#7987=CARTESIAN_POINT ( 'NONE',  ( -103.6230814261940623, 108.4577647952326487, 44.49395664845071252 ) ) ;
#7996=CARTESIAN_POINT ( 'NONE',  ( -104.3997176008718810, -123.8500140569469181, 0.4893052421375900241 ) ) ;
#7997=CARTESIAN_POINT ( 'NONE',  ( -136.7839808106123485, 61.60861089918629574, 34.73673964685640669 ) ) ;
#7998=ORIENTED_EDGE ( 'NONE', *, *, #9541, .T. ) ;
#8003=CARTESIAN_POINT ( 'NONE',  ( -96.25732604711518547, -115.9704170962522198, 30.03172575643280595 ) ) ;
#8006=CARTESIAN_POINT ( 'NONE',  ( -90.67862352884070276, -119.4897427140443682, -6.860445880948178754 ) ) ;
#8010=CARTESIAN_POINT ( 'NONE',  ( 176.1792632384392334, -186.5724904703758682, 30.00000000000000000 ) ) ;
#8011=CARTESIAN_POINT ( 'NONE',  ( -134.0015816819225165, -77.97298368087619735, 36.53274635918683799 ) ) ;
#8012=ORIENTED_EDGE ( 'NONE', *, *, #19258, .F. ) ;
#8013=CARTESIAN_POINT ( 'NONE',  ( -123.2780666175815298, 53.67120218771228934, -27.39856999340311106 ) ) ;
#8018=ORIENTED_EDGE ( 'NONE', *, *, #12852, .F. ) ;
#8021=CARTESIAN_POINT ( 'NONE',  ( -142.7819598182928189, -16.97992044938526490, 17.29344121494534647 ) ) ;
#8035=DIRECTION ( 'NONE',  ( -1.000000000000000000, 0.000000000000000000, 0.000000000000000000 ) ) ;
#8037=ORIENTED_EDGE ( 'NONE', *, *, #14056, .T. ) ;
#8038=ORIENTED_EDGE ( 'NONE', *, *, #11603, .T. ) ;
#8039=ORIENTED_EDGE ( 'NONE', *, *, #5666, .F. ) ;
#8042=CARTESIAN_POINT ( 'NONE',  ( 126.5370453525553387, 80.55045718954887946, 49.99999999999999289 ) ) ;
#8046=CARTESIAN_POINT ( 'NONE',  ( -107.4999999999999858, -118.5063289449133777, 40.00000000000000000 ) ) ;
#8049=DIRECTION ( 'NONE',  ( 0.5742676632334713371, -0.8186676071302493307, 0.000000000000000000 ) ) ;
#8053=AXIS2_PLACEMENT_3D ( 'NONE', #5658, #8915, #16035 ) ;
#8059=CARTESIAN_POINT ( 'NONE',  ( 0.000000000000000000, 0.000000000000000000, -105.0000000000000142 ) ) ;
#8060=CARTESIAN_POINT ( 'NONE',  ( -29.99999999999887379, 275.0000000000000000, -2.500000000000847766 ) ) ;
#8061=DIRECTION ( 'NONE',  ( 0.2225209339563182509, -0.9749279121818227312, 0.000000000000000000 ) ) ;
#8073=DIRECTION ( 'NONE',  ( 0.000000000000000000, 0.000000000000000000, 1.000000000000000000 ) ) ;
#8081=CARTESIAN_POINT ( 'NONE',  ( -110.0000000000000142, 275.0000000000000000, 5.000000000000000888 ) ) ;
#8083=AXIS2_PLACEMENT_3D ( 'NONE', #13983, #18293, #20226 ) ;
#8094=CARTESIAN_POINT ( 'NONE',  ( -98.17232476720997170, -133.0668712321317741, 6.370955715338651792 ) ) ;
#8095=CARTESIAN_POINT ( 'NONE',  ( -149.9004280568922809, 5.577261304408828835, 7.878901868833741773 ) ) ;
#8096=ORIENTED_EDGE ( 'NONE', *, *, #7253, .T. ) ;
#8099=CARTESIAN_POINT ( 'NONE',  ( 128.8937720816053343, -76.72575536401154750, 47.58463383931721324 ) ) ;
#8100=AXIS2_PLACEMENT_3D ( 'NONE', #7121, #14987, #12950 ) ;
#8102=CARTESIAN_POINT ( 'NONE',  ( -91.69714670201400963, -118.7099181436120432, -7.507405155613667169 ) ) ;
#8103=FACE_BOUND ( 'NONE', #15734, .T. ) ;
#8105=ADVANCED_FACE ( 'NONE', ( #2181 ), #6782, .F. ) ;
#8110=DIRECTION ( 'NONE',  ( 1.000000000000000000, 0.000000000000000000, 0.000000000000000000 ) ) ;
#8112=ADVANCED_FACE ( 'NONE', ( #224 ), #12807, .T. ) ;
#8121=ORIENTED_EDGE ( 'NONE', *, *, #11704, .T. ) ;
#8122=CARTESIAN_POINT ( 'NONE',  ( -144.5247897876143384, -14.68938321827882376, 10.83348343318937523 ) ) ;
#8125=CARTESIAN_POINT ( 'NONE',  ( -159.9599531637108782, -36.50981547337168109, 49.99999999999999289 ) ) ;
#8138=CARTESIAN_POINT ( 'NONE',  ( 133.6648977371254148, -68.07564730484348559, 39.79982607272240358 ) ) ;
#8139=CARTESIAN_POINT ( 'NONE',  ( 134.3942145021295289, -75.36533733386920630, 34.64617282042209467 ) ) ;
#8140=ORIENTED_EDGE ( 'NONE', *, *, #15528, .T. ) ;
#8144=VECTOR ( 'NONE', #17777, 1000.000000000000000 ) ;
#8150=CARTESIAN_POINT ( 'NONE',  ( -123.8492616149702741, -72.31991210363501921, 0.000000000000000000 ) ) ;
#8152=CARTESIAN_POINT ( 'NONE',  ( 156.4179374840099683, -52.02840013023883614, 49.99999999999999289 ) ) ;
#8154=CARTESIAN_POINT ( 'NONE',  ( -189.9999999999988916, 265.0000000000000000, 5.000000000000268230 ) ) ;
#8159=ADVANCED_FACE ( 'NONE', ( #13191 ), #16584, .T. ) ;
#8162=AXIS2_PLACEMENT_3D ( 'NONE', #8125, #2101, #5076 ) ;
#8163=ADVANCED_FACE ( 'NONE', ( #19457 ), #3394, .F. ) ;
#8167=CARTESIAN_POINT ( 'NONE',  ( 82.03125000000004263, -125.5821405433013780, 30.00000000000000000 ) ) ;
#8179=ORIENTED_EDGE ( 'NONE', *, *, #5124, .T. ) ;
#8182=DIRECTION ( 'NONE',  ( 1.613511099790691498E-16, -1.000000000000000000, 0.000000000000000000 ) ) ;
#8183=DIRECTION ( 'NONE',  ( -1.000000000000000000, 0.000000000000000000, 0.000000000000000000 ) ) ;
#8193=CARTESIAN_POINT ( 'NONE',  ( -78.11514653572207578, 128.0610818020408601, 29.21201989692128365 ) ) ;
#8206=CARTESIAN_POINT ( 'NONE',  ( -96.82170812967324025, -114.6249810635578541, 3.420849988137867559 ) ) ;
#8207=CARTESIAN_POINT ( 'NONE',  ( -112.4702966502606643, 83.46484221923026325, 39.99999999999999289 ) ) ;
#8212=DIRECTION ( 'NONE',  ( -0.000000000000000000, -0.000000000000000000, -1.000000000000000000 ) ) ;
#8214=EDGE_CURVE ( 'NONE', #1847, #15721, #12163, .T. ) ;
#8216=DIRECTION ( 'NONE',  ( -0.000000000000000000, -0.000000000000000000, 1.000000000000000000 ) ) ;
#8217=ORIENTED_EDGE ( 'NONE', *, *, #12979, .F. ) ;
#8218=ORIENTED_EDGE ( 'NONE', *, *, #3733, .F. ) ;
#8221=LINE ( 'NONE', #11686, #6990 ) ;
#8223=CARTESIAN_POINT ( 'NONE',  ( -135.1060089022256818, -65.16414933467417825, 10.00000000000000178 ) ) ;
#8225=CARTESIAN_POINT ( 'NONE',  ( -7.499999999999583444, -60.00000000000000000, -105.0000000000000142 ) ) ;
#8227=CARTESIAN_POINT ( 'NONE',  ( -7.500000000000001776, 60.00000000000000000, -100.0000000000000000 ) ) ;
#8231=DIRECTION ( 'NONE',  ( 0.000000000000000000, 0.000000000000000000, 1.000000000000000000 ) ) ;
#8234=ORIENTED_EDGE ( 'NONE', *, *, #5529, .F. ) ;
#8239=ORIENTED_EDGE ( 'NONE', *, *, #6286, .T. ) ;
#8241=ADVANCED_FACE ( 'NONE', ( #3580 ), #19332, .T. ) ;
#8247=CARTESIAN_POINT ( 'NONE',  ( -102.1674435767773019, -127.3754966267598121, 38.48120063021033843 ) ) ;
#8248=LINE ( 'NONE', #14195, #17254 ) ;
#8251=CARTESIAN_POINT ( 'NONE',  ( 134.2425157119613459, -66.92593549375909845, 2.347053091275800973 ) ) ;
#8257=FACE_OUTER_BOUND ( 'NONE', #11445, .T. ) ;
#8258=ADVANCED_FACE ( 'NONE', ( #897 ), #5421, .F. ) ;
#8260=AXIS2_PLACEMENT_3D ( 'NONE', #7896, #11067, #12396 ) ;
#8261=CARTESIAN_POINT ( 'NONE',  ( -141.1002642289847131, -19.56295509475995686, -11.10155280223196961 ) ) ;
#8265=DIRECTION ( 'NONE',  ( -1.000000000000000000, 0.000000000000000000, 0.000000000000000000 ) ) ;
#8268=ORIENTED_EDGE ( 'NONE', *, *, #2547, .T. ) ;
#8275=EDGE_CURVE ( 'NONE', #8865, #10778, #4066, .T. ) ;
#8276=CARTESIAN_POINT ( 'NONE',  ( -107.4999999999999716, -200.0000000000000000, 40.00000000000000000 ) ) ;
#8279=DIRECTION ( 'NONE',  ( 0.8186676071302501079, -0.5742676632334704490, 0.000000000000000000 ) ) ;
#8289=CARTESIAN_POINT ( 'NONE',  ( 96.22303100968534295, -115.1714777947412074, 35.55703238301298796 ) ) ;
#8290=VERTEX_POINT ( 'NONE', #11642 ) ;
#8292=CARTESIAN_POINT ( 'NONE',  ( -71.68195843679204415, 131.7647605457766815, -6.617816534668000905 ) ) ;
#8299=ORIENTED_EDGE ( 'NONE', *, *, #19128, .F. ) ;
#8301=CARTESIAN_POINT ( 'NONE',  ( -122.5362376193369442, 86.52404603474892042, 42.99233187391926947 ) ) ;
#8306=CARTESIAN_POINT ( 'NONE',  ( -84.12422660803102303, -124.1903156958427559, 0.7897671010553509729 ) ) ;
#8310=DIRECTION ( 'NONE',  ( 0.2225209339563182231, -0.9749279121818227312, 0.000000000000000000 ) ) ;
#8312=PLANE ( 'NONE',  #9141 ) ;
#8316=CARTESIAN_POINT ( 'NONE',  ( -130.0921664654442509, 42.14112310077317858, -23.71395948546228283 ) ) ;
#8324=ADVANCED_FACE ( 'NONE', ( #16562 ), #2542, .T. ) ;
#8331=DIRECTION ( 'NONE',  ( 1.000000000000000000, 0.000000000000000000, 0.000000000000000000 ) ) ;
#8333=CARTESIAN_POINT ( 'NONE',  ( 60.00000000000000711, 6.284666409917639535E-13, -105.0000000000000142 ) ) ;
#8338=( BOUNDED_SURFACE ( )  B_SPLINE_SURFACE ( 3, 2, ( 
 ( #3828, #19675, #5671 ),
 ( #14965, #14679, #3928 ),
 ( #16420, #10071, #7005 ),
 ( #16323, #13035, #664 ),
 ( #6910, #2307, #14770 ),
 ( #855, #15069, #954 ),
 ( #11886, #5467, #11789 ),
 ( #10169, #2403, #4126 ),
 ( #5568, #18050, #7204 ),
 ( #6809, #11988, #4433 ),
 ( #9030, #5876, #1366 ),
 ( #1260, #3009, #7594 ),
 ( #12300, #16918, #18451 ),
 ( #10663, #15272, #5975 ),
 ( #16713, #7395, #2698 ),
 ( #2906, #20081, #7498 ),
 ( #2806, #13734, #4324 ),
 ( #19978, #1154, #6080 ),
 ( #13630, #19874, #8927 ),
 ( #15376, #17023, #18556 ),
 ( #13836, #10868, #4538 ),
 ( #9239, #12197, #17124 ),
 ( #9135, #1468, #10770 ),
 ( #15483, #13526, #9342 ),
 ( #7698, #19775, #15171 ),
 ( #13941, #20186, #12089 ),
 ( #18349, #6187, #10558 ),
 ( #16814, #12407, #18667 ),
 ( #4644, #3112, #1048 ),
 ( #5773, #7297, #18243 ) ),
 .UNSPECIFIED., .F., .F., .F. ) 
 B_SPLINE_SURFACE_WITH_KNOTS ( ( 4, 2, 2, 2, 2, 2, 2, 2, 2, 2, 2, 2, 2, 2, 4 ),
 ( 3, 3 ),
 ( 0.01087485647533276839, 0.01538493460406631201, 0.01651245413624969835, 0.01763997366843308295, 0.01989501273279985563, 0.02102253226498324024, 0.02215005179716662831, 0.02440509086153339752, 0.02891516899026694287, 0.03117020805463371555, 0.03342524711900048823, 0.03793532524773403358, 0.04019036431210080279, 0.04244540337646757200, 0.04695548150520111735 ),
 ( 0.000000000000000000, 1.000000000000000000 ),
 .UNSPECIFIED. ) 
 GEOMETRIC_REPRESENTATION_ITEM ( )  RATIONAL_B_SPLINE_SURFACE ( (
 ( 1.000000000000000000, 0.9212076576725561905, 1.000000000000000000),
 ( 1.000000000000000000, 0.9211983545445133759, 1.000000000000000000),
 ( 1.000000000000000000, 0.9192884530627715156, 1.000000000000000000),
 ( 1.000000000000000000, 0.9147257148663896498, 1.000000000000000000),
 ( 1.000000000000000000, 0.9137002753876459771, 1.000000000000000000),
 ( 1.000000000000000000, 0.9114460110779207813, 1.000000000000000000),
 ( 1.000000000000000000, 0.9102239901659180399, 1.000000000000000000),
 ( 1.000000000000000000, 0.9062907615862647592, 1.000000000000000000),
 ( 1.000000000000000000, 0.9033134084428577903, 1.000000000000000000),
 ( 1.000000000000000000, 0.8983619464026604273, 1.000000000000000000),
 ( 1.000000000000000000, 0.8966302762932976123, 1.000000000000000000),
 ( 1.000000000000000000, 0.8930095736512202453, 1.000000000000000000),
 ( 1.000000000000000000, 0.8911146393079001360, 1.000000000000000000),
 ( 1.000000000000000000, 0.8852539528818137438, 1.000000000000000000),
 ( 1.000000000000000000, 0.8811119717501193493, 1.000000000000000000),
 ( 1.000000000000000000, 0.8680569459630019802, 1.000000000000000000),
 ( 1.000000000000000000, 0.8585210289498550473, 1.000000000000000000),
 ( 1.000000000000000000, 0.8431029601255768391, 1.000000000000000000),
 ( 1.000000000000000000, 0.8377859708360378965, 1.000000000000000000),
 ( 1.000000000000000000, 0.8269824639698531987, 1.000000000000000000),
 ( 1.000000000000000000, 0.8214732595402479687, 1.000000000000000000),
 ( 1.000000000000000000, 0.8046428831056189335, 1.000000000000000000),
 ( 1.000000000000000000, 0.7930208592508356524, 1.000000000000000000),
 ( 1.000000000000000000, 0.7750195416464756848, 1.000000000000000000),
 ( 1.000000000000000000, 0.7688986879967366628, 1.000000000000000000),
 ( 1.000000000000000000, 0.7566232400043410022, 1.000000000000000000),
 ( 1.000000000000000000, 0.7504663834241424025, 1.000000000000000000),
 ( 1.000000000000000000, 0.7319497228655966747, 1.000000000000000000),
 ( 1.000000000000000000, 0.7195437534944766345, 1.000000000000000000),
 ( 1.000000000000000000, 0.7071067811865472397, 1.000000000000000000) ) ) 
 REPRESENTATION_ITEM ( '' )  SURFACE ( )  );
#8339=ORIENTED_EDGE ( 'NONE', *, *, #2361, .T. ) ;
#8344=LINE ( 'NONE', #10085, #2404 ) ;
#8348=DIRECTION ( 'NONE',  ( 0.000000000000000000, -0.000000000000000000, 1.000000000000000000 ) ) ;
#8351=CARTESIAN_POINT ( 'NONE',  ( 133.9144309718294608, -67.58001956112548214, 1.097951290815503356 ) ) ;
#8354=DIRECTION ( 'NONE',  ( 1.000000000000000000, 0.000000000000000000, 0.000000000000000000 ) ) ;
#8360=EDGE_CURVE ( 'NONE', #10908, #5623, #15110, .T. ) ;
#8363=CARTESIAN_POINT ( 'NONE',  ( -78.37722339831623231, 116.0043570404596522, -9.999999999999984013 ) ) ;
#8366=AXIS2_PLACEMENT_3D ( 'NONE', #8154, #14301, #9789 ) ;
#8369=ORIENTED_EDGE ( 'NONE', *, *, #10212, .F. ) ;
#8370=DIRECTION ( 'NONE',  ( 0.000000000000000000, 0.000000000000000000, 1.000000000000000000 ) ) ;
#8371=VERTEX_POINT ( 'NONE', #9390 ) ;
#8372=AXIS2_PLACEMENT_3D ( 'NONE', #17954, #13314, #3923 ) ;
#8373=EDGE_CURVE ( 'NONE', #1151, #15881, #3464, .T. ) ;
#8377=DIRECTION ( 'NONE',  ( -0.000000000000000000, 0.000000000000000000, -1.000000000000000000 ) ) ;
#8378=LINE ( 'NONE', #308, #7548 ) ;
#8381=CARTESIAN_POINT ( 'NONE',  ( 97.83396368271631616, -133.5156904852159983, 7.427229934397163724 ) ) ;
#8383=CARTESIAN_POINT ( 'NONE',  ( 144.1130761623740568, -69.50842595698583182, 10.00000000000000178 ) ) ;
#8386=DIRECTION ( 'NONE',  ( 0.000000000000000000, 0.000000000000000000, 1.000000000000000000 ) ) ;
#8395=AXIS2_PLACEMENT_3D ( 'NONE', #13096, #7073, #4192 ) ;
#8397=DIRECTION ( 'NONE',  ( 0.000000000000000000, 0.000000000000000000, -1.000000000000000000 ) ) ;
#8400=CIRCLE ( 'NONE', #4140, 150.0000000000000284 ) ;
#8401=ORIENTED_EDGE ( 'NONE', *, *, #3412, .T. ) ;
#8406=ORIENTED_EDGE ( 'NONE', *, *, #4093, .T. ) ;
#8408=CARTESIAN_POINT ( 'NONE',  ( -98.61625419099686951, -132.4696700755308996, 5.394883550556022200 ) ) ;
#8410=CARTESIAN_POINT ( 'NONE',  ( -82.03125000000001421, -125.5821405433014348, 8.545780905957366613 ) ) ;
#8416=CARTESIAN_POINT ( 'NONE',  ( 0.000000000000000000, 0.000000000000000000, 0.000000000000000000 ) ) ;
#8417=CARTESIAN_POINT ( 'NONE',  ( 0.000000000000000000, 0.000000000000000000, 39.99999999999999289 ) ) ;
#8421=CARTESIAN_POINT ( 'NONE',  ( -139.6549061548003579, 6.995471948008744612, -13.59954962453111094 ) ) ;
#8428=CARTESIAN_POINT ( 'NONE',  ( 175.8776271403848739, -36.50981547336952104, 49.99999999999999289 ) ) ;
#8434=CARTESIAN_POINT ( 'NONE',  ( -124.4044063703166785, -83.81803169341358739, -9.885272611403726373 ) ) ;
#8453=ORIENTED_EDGE ( 'NONE', *, *, #14167, .T. ) ;
#8461=( BOUNDED_SURFACE ( )  B_SPLINE_SURFACE ( 3, 2, ( 
 ( #8999, #15241, #1228 ),
 ( #1441, #16887, #2571 ),
 ( #12376, #7467, #16991 ),
 ( #15343, #1336, #13704 ),
 ( #13809, #10429, #2674 ),
 ( #8898, #4403, #5949 ),
 ( #2876, #20054, #15141 ),
 ( #18523, #1124, #7270 ) ),
 .UNSPECIFIED., .F., .F., .F. ) 
 B_SPLINE_SURFACE_WITH_KNOTS ( ( 4, 2, 2, 4 ),
 ( 3, 3 ),
 ( -0.01955877148976023494, -0.007974286041951373499, -0.002182043318046942345, 0.003610199405857488809 ),
 ( 0.7413449081104728222, 1.000000000000000000 ),
 .UNSPECIFIED. ) 
 GEOMETRIC_REPRESENTATION_ITEM ( )  RATIONAL_B_SPLINE_SURFACE ( (
 ( 0.9153618001336600862, 0.9429157744658526186, 1.000000000000000000),
 ( 0.9156768966432011769, 0.9431282912755682979, 1.000000000000000000),
 ( 0.9159077319687689567, 0.9432839781380815136, 1.000000000000000000),
 ( 0.9161393926374885588, 0.9434402216532019603, 1.000000000000000000),
 ( 0.9161974188647875605, 0.9434793574364683799, 1.000000000000000000),
 ( 0.9162751259529473558, 0.9435317669743971125, 1.000000000000000000),
 ( 0.9162946951553196939, 0.9435449654210028569, 1.000000000000000000),
 ( 0.9162945902535410969, 0.9435448946700086825, 1.000000000000000000) ) ) 
 REPRESENTATION_ITEM ( '' )  SURFACE ( )  );
#8468=EDGE_CURVE ( 'NONE', #9870, #10982, #4474, .T. ) ;
#8474=FACE_OUTER_BOUND ( 'NONE', #12617, .T. ) ;
#8476=CARTESIAN_POINT ( 'NONE',  ( -83.18633423686334538, -124.8217490215423879, 37.05209266191527462 ) ) ;
#8480=VECTOR ( 'NONE', #4735, 1000.000000000000000 ) ;
#8481=VECTOR ( 'NONE', #1590, 1000.000000000000000 ) ;
#8484=DIRECTION ( 'NONE',  ( 0.000000000000000000, 0.000000000000000000, 1.000000000000000000 ) ) ;
#8491=CARTESIAN_POINT ( 'NONE',  ( 100.7812500000000000, -111.0996833858562525, -10.00000000000000178 ) ) ;
#8492=CARTESIAN_POINT ( 'NONE',  ( 0.000000000000000000, 164.0736214083062805, 39.99999999999999289 ) ) ;
#8503=CARTESIAN_POINT ( 'NONE',  ( -85.53020504959707182, -140.9188050298390067, 39.99999999999999289 ) ) ;
#8506=CARTESIAN_POINT ( 'NONE',  ( 100.8144812491504325, -129.3825068912776999, 2.561523122930402074 ) ) ;
#8508=CARTESIAN_POINT ( 'NONE',  ( -91.90390622750267369, -118.5498891763755864, -7.627268136224651940 ) ) ;
#8512=PRODUCT_DEFINITION_FORMATION_WITH_SPECIFIED_SOURCE ( 'ANY', '', #513, .NOT_KNOWN. ) ;
#8520=EDGE_CURVE ( 'NONE', #8371, #12416, #3100, .T. ) ;
#8521=CARTESIAN_POINT ( 'NONE',  ( 100.7812500000000000, -111.0996833858562525, -10.00000000000000178 ) ) ;
#8527=EDGE_CURVE ( 'NONE', #16530, #1562, #2126, .T. ) ;
#8528=EDGE_CURVE ( 'NONE', #7267, #22, #17177, .T. ) ;
#8530=EDGE_CURVE ( 'NONE', #380, #12588, #15852, .T. ) ;
#8534=ORIENTED_EDGE ( 'NONE', *, *, #10693, .F. ) ;
#8536=DIRECTION ( 'NONE',  ( 0.000000000000000000, 0.000000000000000000, 1.000000000000000000 ) ) ;
#8539=CARTESIAN_POINT ( 'NONE',  ( -135.1060089022256818, -65.16414933467417825, 10.00000000000000178 ) ) ;
#8545=ORIENTED_EDGE ( 'NONE', *, *, #17671, .T. ) ;
#8554=EDGE_CURVE ( 'NONE', #3346, #5032, #14197, .T. ) ;
#8555=ORIENTED_EDGE ( 'NONE', *, *, #287, .T. ) ;
#8556=DIRECTION ( 'NONE',  ( -1.000000000000000000, 0.000000000000000000, 0.000000000000000000 ) ) ;
#8559=DIRECTION ( 'NONE',  ( -0.000000000000000000, -0.000000000000000000, -1.000000000000000000 ) ) ;
#8567=ORIENTED_EDGE ( 'NONE', *, *, #3471, .F. ) ;
#8569=CARTESIAN_POINT ( 'NONE',  ( -110.0000000000000142, 275.0000000000000000, -75.00000000000000000 ) ) ;
#8573=CARTESIAN_POINT ( 'NONE',  ( -110.0000000000000142, 265.0000000000000000, -67.49999999999997158 ) ) ;
#8576=CARTESIAN_POINT ( 'NONE',  ( -110.0000000000000000, 275.0000000000000000, 104.9999999999999858 ) ) ;
#8580=LINE ( 'NONE', #804, #18577 ) ;
#8582=CIRCLE ( 'NONE', #87, 150.0000000000000284 ) ;
#8585=ORIENTED_EDGE ( 'NONE', *, *, #16366, .T. ) ;
#8589=CARTESIAN_POINT ( 'NONE',  ( 86.10242266703180292, -122.8274731153597799, -2.462352461605555654 ) ) ;
#8592=EDGE_CURVE ( 'NONE', #12327, #14347, #7948, .T. ) ;
#8593=DIRECTION ( 'NONE',  ( 0.000000000000000000, 0.000000000000000000, 1.000000000000000000 ) ) ;
#8603=AXIS2_PLACEMENT_3D ( 'NONE', #13212, #11593, #17842 ) ;
#8604=CARTESIAN_POINT ( 'NONE',  ( 100.6915138157988991, -129.5610470606159481, 2.673863972956103563 ) ) ;
#8605=CARTESIAN_POINT ( 'NONE',  ( -96.12039245752636418, -116.0188909747188575, 9.827413591029802831 ) ) ;
#8608=CARTESIAN_POINT ( 'NONE',  ( -87.33261371895457614, -121.9603527571197787, -3.999215385619499408 ) ) ;
#8609=DIRECTION ( 'NONE',  ( -0.000000000000000000, -1.000000000000000000, -0.000000000000000000 ) ) ;
#8611=AXIS2_PLACEMENT_3D ( 'NONE', #13253, #6841, #4057 ) ;
#8616=CARTESIAN_POINT ( 'NONE',  ( 120.7779226595531128, 102.2982297021113141, 49.99999999999999289 ) ) ;
#8619=EDGE_CURVE ( 'NONE', #15878, #573, #17813, .T. ) ;
#8622=EDGE_LOOP ( 'NONE', ( #7985, #14874, #11756, #13392 ) ) ;
#8623=CARTESIAN_POINT ( 'NONE',  ( -176.5810126522742110, -187.6736222527391647, 8.827867842925929409 ) ) ;
#8628=DIRECTION ( 'NONE',  ( -0.000000000000000000, -0.000000000000000000, -1.000000000000000000 ) ) ;
#8630=LINE ( 'NONE', #3924, #1967 ) ;
#8632=CARTESIAN_POINT ( 'NONE',  ( -129.1041139275565683, -76.37100075998222337, -7.395096211630200145 ) ) ;
#8646=DIRECTION ( 'NONE',  ( -3.129754055707530415E-16, 1.000000000000000000, -0.000000000000000000 ) ) ;
#8647=CARTESIAN_POINT ( 'NONE',  ( -32.50000000000000000, 0.000000000000000000, -105.0000000000000142 ) ) ;
#8649=FACE_OUTER_BOUND ( 'NONE', #15412, .T. ) ;
#8651=CIRCLE ( 'NONE', #20087, 9.999999999999992895 ) ;
#8653=DIRECTION ( 'NONE',  ( 0.000000000000000000, 1.000000000000000000, 0.000000000000000000 ) ) ;
#8661=FACE_OUTER_BOUND ( 'NONE', #2955, .T. ) ;
#8664=DIRECTION ( 'NONE',  ( 0.000000000000000000, 0.000000000000000000, -1.000000000000000000 ) ) ;
#8666=AXIS2_PLACEMENT_3D ( 'NONE', #1867, #13004, #6878 ) ;
#8667=EDGE_CURVE ( 'NONE', #14077, #1203, #375, .T. ) ;
#8671=ORIENTED_EDGE ( 'NONE', *, *, #5936, .T. ) ;
#8674=DIRECTION ( 'NONE',  ( 0.000000000000000000, 0.000000000000000000, -1.000000000000000000 ) ) ;
#8679=DIRECTION ( 'NONE',  ( 0.000000000000000000, 0.000000000000000000, 1.000000000000000000 ) ) ;
#8681=CARTESIAN_POINT ( 'NONE',  ( 0.000000000000000000, 60.00000000000000000, -100.0000000000000000 ) ) ;
#8685=CARTESIAN_POINT ( 'NONE',  ( 87.35350281426670449, -121.9411179691607003, -3.975120933794691336 ) ) ;
#8689=DIRECTION ( 'NONE',  ( 0.000000000000000000, 0.000000000000000000, -1.000000000000000000 ) ) ;
#8690=ORIENTED_EDGE ( 'NONE', *, *, #17948, .T. ) ;
#8691=VECTOR ( 'NONE', #8484, 1000.000000000000000 ) ;
#8700=CARTESIAN_POINT ( 'NONE',  ( -175.4992877478424873, -40.00000000000000000, -115.0000000000000142 ) ) ;
#8703=CARTESIAN_POINT ( 'NONE',  ( -140.0000000000000568, -2.688074818803143362, 23.02775637731987501 ) ) ;
#8706=CIRCLE ( 'NONE', #8395, 150.0000000000000284 ) ;
#8718=ORIENTED_EDGE ( 'NONE', *, *, #16159, .T. ) ;
#8726=ADVANCED_FACE ( 'NONE', ( #15990 ), #15263, .F. ) ;
#8728=CARTESIAN_POINT ( 'NONE',  ( -127.7402033587038375, -78.63140257242432085, -8.470234954248022419 ) ) ;
#8729=FACE_OUTER_BOUND ( 'NONE', #13452, .T. ) ;
#8737=ORIENTED_EDGE ( 'NONE', *, *, #11104, .F. ) ;
#8740=ORIENTED_EDGE ( 'NONE', *, *, #14167, .F. ) ;
#8747=VECTOR ( 'NONE', #776, 1000.000000000000000 ) ;
#8749=ORIENTED_EDGE ( 'NONE', *, *, #17619, .F. ) ;
#8750=DIRECTION ( 'NONE',  ( 1.000000000000000000, -0.000000000000000000, -0.000000000000000000 ) ) ;
#8753=FACE_OUTER_BOUND ( 'NONE', #14535, .T. ) ;
#8755=CARTESIAN_POINT ( 'NONE',  ( 124.4044063703119321, -83.81803169342077808, 49.88527261140372815 ) ) ;
#8759=CARTESIAN_POINT ( 'NONE',  ( -110.0000000000000142, 265.0000000000000000, -75.00000000000000000 ) ) ;
#8767=ORIENTED_EDGE ( 'NONE', *, *, #12607, .F. ) ;
#8770=CARTESIAN_POINT ( 'NONE',  ( -100.7812499999999716, -111.0996833858562809, 49.99999999999999289 ) ) ;
#8784=AXIS2_PLACEMENT_3D ( 'NONE', #17849, #3826, #6906 ) ;
#8787=CARTESIAN_POINT ( 'NONE',  ( 83.18633423686338801, -124.8217490215423737, 2.947907338084742701 ) ) ;
#8789=ORIENTED_EDGE ( 'NONE', *, *, #6647, .T. ) ;
#8800=CARTESIAN_POINT ( 'NONE',  ( 92.40373333587093896, -118.1608478542247553, -7.903026561454264076 ) ) ;
#8807=CARTESIAN_POINT ( 'NONE',  ( -134.8030718230775449, -47.09494809331346232, 49.99999999999999289 ) ) ;
#8819=VERTEX_POINT ( 'NONE', #15140 ) ;
#8820=AXIS2_PLACEMENT_3D ( 'NONE', #5157, #6489, #9548 ) ;
#8821=CARTESIAN_POINT ( 'NONE',  ( 133.8357118474723677, -78.97256401901070433, 2.952839103891145900 ) ) ;
#8824=CARTESIAN_POINT ( 'NONE',  ( -98.08520584366951311, -113.5061255252650483, 38.12154030620245493 ) ) ;
#8829=FACE_OUTER_BOUND ( 'NONE', #7013, .T. ) ;
#8830=DIRECTION ( 'NONE',  ( 0.000000000000000000, 0.000000000000000000, 1.000000000000000000 ) ) ;
#8832=LINE ( 'NONE', #19777, #4479 ) ;
#8836=EDGE_CURVE ( 'NONE', #11005, #16596, #8996, .T. ) ;
#8837=ORIENTED_EDGE ( 'NONE', *, *, #5262, .T. ) ;
#8838=VERTEX_POINT ( 'NONE', #10428 ) ;
#8840=ORIENTED_EDGE ( 'NONE', *, *, #1979, .F. ) ;
#8841=DIRECTION ( 'NONE',  ( -1.000000000000000000, 1.224646799147352961E-16, 0.000000000000000000 ) ) ;
#8850=EDGE_LOOP ( 'NONE', ( #7867, #3239, #777, #18676 ) ) ;
#8853=CARTESIAN_POINT ( 'NONE',  ( -134.7188131032333445, -72.93593548660989256, 10.00000000000000178 ) ) ;
#8854=CARTESIAN_POINT ( 'NONE',  ( 107.5000000000000284, -118.5063289449133492, 50.00000000000000000 ) ) ;
#8855=CARTESIAN_POINT ( 'NONE',  ( 127.3324793557656136, -79.33838548636531129, 40.86166200754897204 ) ) ;
#8864=CARTESIAN_POINT ( 'NONE',  ( -110.0000000000000000, 265.0000000000000000, 104.9999999999999858 ) ) ;
#8865=VERTEX_POINT ( 'NONE', #15450 ) ;
#8873=CARTESIAN_POINT ( 'NONE',  ( -132.4400928985788823, -70.43137869103949811, 42.82464599639617120 ) ) ;
#8890=CARTESIAN_POINT ( 'NONE',  ( -97.60910239587758497, -133.8115172545150529, 31.48501029038536814 ) ) ;
#8895=ORIENTED_EDGE ( 'NONE', *, *, #19258, .T. ) ;
#8898=CARTESIAN_POINT ( 'NONE',  ( -141.6220008579448972, -18.66460740341266700, -11.97000856754251785 ) ) ;
#8900=CARTESIAN_POINT ( 'NONE',  ( -163.5019688434124419, -20.99123081650240863, 39.99999999999999289 ) ) ;
#8903=CARTESIAN_POINT ( 'NONE',  ( 163.5019688434126977, -20.99123081650019529, 49.99999999999999289 ) ) ;
#8915=DIRECTION ( 'NONE',  ( 0.000000000000000000, 0.000000000000000000, -1.000000000000000000 ) ) ;
#8918=CARTESIAN_POINT ( 'NONE',  ( 133.1920331248151115, -82.53376026279583755, 1.486861419600814305 ) ) ;
#8926=CARTESIAN_POINT ( 'NONE',  ( -133.8517991834421821, -78.87665408946898538, 3.000515938330789112 ) ) ;
#8927=CARTESIAN_POINT ( 'NONE',  ( 133.5298479455745735, -80.72596075551817307, 2.158131001320439335 ) ) ;
#8928=VECTOR ( 'NONE', #2097, 1000.000000000000000 ) ;
#8929=DIRECTION ( 'NONE',  ( 0.000000000000000000, 0.000000000000000000, -1.000000000000000000 ) ) ;
#8930=CARTESIAN_POINT ( 'NONE',  ( 133.2435246741110006, -68.89240257401093004, 30.00000000000000000 ) ) ;
#8932=EDGE_LOOP ( 'NONE', ( #5380, #44 ) ) ;
#8946=EDGE_LOOP ( 'NONE', ( #18062, #1640 ) ) ;
#8953=DIRECTION ( 'NONE',  ( -0.000000000000000000, -0.000000000000000000, -1.000000000000000000 ) ) ;
#8958=ADVANCED_FACE ( 'NONE', ( #15555 ), #17304, .T. ) ;
#8962=VECTOR ( 'NONE', #16883, 1000.000000000000000 ) ;
#8965=CYLINDRICAL_SURFACE ( 'NONE', #11362, 7.500000000000006217 ) ;
#8966=ORIENTED_EDGE ( 'NONE', *, *, #17374, .F. ) ;
#8979=CARTESIAN_POINT ( 'NONE',  ( -134.7188131032333160, -72.93593548660990677, 30.49674468329109445 ) ) ;
#8980=AXIS2_PLACEMENT_3D ( 'NONE', #11450, #12978, #2152 ) ;
#8983=CARTESIAN_POINT ( 'NONE',  ( -71.18887634719365565, -147.8252249328922687, 49.99999999999999289 ) ) ;
#8984=DIRECTION ( 'NONE',  ( 0.000000000000000000, 0.000000000000000000, -1.000000000000000000 ) ) ;
#8988=CARTESIAN_POINT ( 'NONE',  ( -97.91442649640831064, -133.4097810206876034, 32.94424152684068474 ) ) ;
#8991=DIRECTION ( 'NONE',  ( 0.9009688679024154823, 0.4338837391175657809, 0.000000000000000000 ) ) ;
#8996=LINE ( 'NONE', #4196, #8962 ) ;
#8999=CARTESIAN_POINT ( 'NONE',  ( -139.5603828663319916, -18.86179323242330952, -21.49533993996032066 ) ) ;
#9015=EDGE_LOOP ( 'NONE', ( #18853, #17525, #8895, #9828 ) ) ;
#9024=EDGE_CURVE ( 'NONE', #19819, #11232, #7050, .T. ) ;
#9027=DIRECTION ( 'NONE',  ( 0.000000000000000000, 0.000000000000000000, 1.000000000000000000 ) ) ;
#9028=CARTESIAN_POINT ( 'NONE',  ( -133.2472142827617461, -69.01451035579515292, 8.943524711593516585 ) ) ;
#9030=CARTESIAN_POINT ( 'NONE',  ( 133.8370531740367824, -67.73246766859801937, 0.8536925741625657205 ) ) ;
#9036=LINE ( 'NONE', #12413, #17737 ) ;
#9053=VECTOR ( 'NONE', #6533, 1000.000000000000000 ) ;
#9057=CARTESIAN_POINT ( 'NONE',  ( -63.68887634719365565, -147.8252249328922687, 39.99999999999999289 ) ) ;
#9062=EDGE_LOOP ( 'NONE', ( #14196, #1809, #1256, #20061 ) ) ;
#9064=LINE ( 'NONE', #6014, #13808 ) ;
#9065=ORIENTED_EDGE ( 'NONE', *, *, #7854, .F. ) ;
#9077=FACE_OUTER_BOUND ( 'NONE', #10588, .T. ) ;
#9082=CARTESIAN_POINT ( 'NONE',  ( -29.99999999999887379, 275.0000000000000000, 4.999999999999158007 ) ) ;
#9083=FACE_OUTER_BOUND ( 'NONE', #3516, .T. ) ;
#9084=CARTESIAN_POINT ( 'NONE',  ( -109.4759482221338516, 87.26817553548865192, 40.00000000000000000 ) ) ;
#9085=AXIS2_PLACEMENT_3D ( 'NONE', #18237, #10448, #2692 ) ;
#9087=AXIS2_PLACEMENT_3D ( 'NONE', #3395, #11463, #114 ) ;
#9090=ORIENTED_EDGE ( 'NONE', *, *, #6647, .F. ) ;
#9092=CARTESIAN_POINT ( 'NONE',  ( -97.34896704141375778, -115.5410409671962384, 29.72470138523284788 ) ) ;
#9094=ORIENTED_EDGE ( 'NONE', *, *, #18159, .F. ) ;
#9096=CARTESIAN_POINT ( 'NONE',  ( 0.000000000000000000, 0.000000000000000000, -49.99999999999999289 ) ) ;
#9098=CARTESIAN_POINT ( 'NONE',  ( 95.52811048055005472, -116.1520858409644745, 8.469523593983353749 ) ) ;
#9101=VECTOR ( 'NONE', #6563, 1000.000000000000000 ) ;
#9102=EDGE_CURVE ( 'NONE', #4859, #6447, #12575, .T. ) ;
#9106=DIRECTION ( 'NONE',  ( 1.000000000000000000, 0.000000000000000000, 0.000000000000000000 ) ) ;
#9108=CARTESIAN_POINT ( 'NONE',  ( 95.42019791136713991, -116.1393900958193655, 32.10275980689200992 ) ) ;
#9110=AXIS2_PLACEMENT_3D ( 'NONE', #5546, #1028, #7184 ) ;
#9114=AXIS2_PLACEMENT_3D ( 'NONE', #15838, #4585, #7745 ) ;
#9115=ORIENTED_EDGE ( 'NONE', *, *, #12344, .T. ) ;
#9117=EDGE_CURVE ( 'NONE', #3818, #14077, #9654, .T. ) ;
#9119=ORIENTED_EDGE ( 'NONE', *, *, #20172, .T. ) ;
#9122=VERTEX_POINT ( 'NONE', #11244 ) ;
#9124=CARTESIAN_POINT ( 'NONE',  ( 132.8201933467846061, -84.36756360499407492, 0.9536901868107962033 ) ) ;
#9128=DIRECTION ( 'NONE',  ( 0.000000000000000000, 0.000000000000000000, 1.000000000000000000 ) ) ;
#9130=CIRCLE ( 'NONE', #14372, 15.91767397667355155 ) ;
#9135=CARTESIAN_POINT ( 'NONE',  ( 128.0993248974582741, -78.05374007934287306, -8.252068616993026851 ) ) ;
#9136=CARTESIAN_POINT ( 'NONE',  ( -170.2125097089225960, -199.3942630591407692, 0.000000000000000000 ) ) ;
#9138=CARTESIAN_POINT ( 'NONE',  ( -134.3287459046936760, -75.81846210759933058, 35.02824617995954526 ) ) ;
#9141=AXIS2_PLACEMENT_3D ( 'NONE', #2087, #14560, #6491 ) ;
#9143=EDGE_CURVE ( 'NONE', #18380, #1203, #8651, .T. ) ;
#9145=EDGE_CURVE ( 'NONE', #11033, #13667, #2345, .T. ) ;
#9149=CARTESIAN_POINT ( 'NONE',  ( -137.5033450361952418, -27.36572496882791583, 26.67424988177857159 ) ) ;
#9151=DIRECTION ( 'NONE',  ( 0.000000000000000000, 0.000000000000000000, 1.000000000000000000 ) ) ;
#9152=EDGE_LOOP ( 'NONE', ( #7355, #16352, #16009, #10670, #7115, #16058 ) ) ;
#9154=CARTESIAN_POINT ( 'NONE',  ( -130.9868171408399462, -91.88282611735537841, 50.00000000000000000 ) ) ;
#9160=CARTESIAN_POINT ( 'NONE',  ( 170.2125097089226244, -199.3942630591406839, 0.000000000000000000 ) ) ;
#9164=CARTESIAN_POINT ( 'NONE',  ( 130.0656023054208106, -74.72982709287474279, 46.44206350853437471 ) ) ;
#9177=CARTESIAN_POINT ( 'NONE',  ( -163.5019688434124419, -20.99123081650240863, 39.99999999999999289 ) ) ;
#9181=DIRECTION ( 'NONE',  ( 1.000000000000000000, 0.000000000000000000, 0.000000000000000000 ) ) ;
#9182=ORIENTED_EDGE ( 'NONE', *, *, #16863, .T. ) ;
#9186=CARTESIAN_POINT ( 'NONE',  ( 75.91068486117727332, -120.9436655338208340, 49.99999999999999289 ) ) ;
#9189=CARTESIAN_POINT ( 'NONE',  ( -132.1979689506645741, -87.16940599486621011, 39.62925165859044796 ) ) ;
#9191=CARTESIAN_POINT ( 'NONE',  ( -91.86817182112051228, 105.6448302045327523, 34.94516124885768704 ) ) ;
#9196=ORIENTED_EDGE ( 'NONE', *, *, #16366, .F. ) ;
#9197=CARTESIAN_POINT ( 'NONE',  ( -97.49999999999997158, -133.9542832461778232, 30.37260543920541878 ) ) ;
#9200=DIRECTION ( 'NONE',  ( -1.000000000000000000, 0.000000000000000000, 0.000000000000000000 ) ) ;
#9203=CARTESIAN_POINT ( 'NONE',  ( 98.53720805795899196, -132.5762351826696204, 5.561479031436848075 ) ) ;
#9207=FACE_OUTER_BOUND ( 'NONE', #686, .T. ) ;
#9212=DIRECTION ( 'NONE',  ( 1.000000000000000000, 0.000000000000000000, 0.000000000000000000 ) ) ;
#9213=CARTESIAN_POINT ( 'NONE',  ( 85.51233150139638894, -123.2383548749651254, 41.61296411234719272 ) ) ;
#9216=CARTESIAN_POINT ( 'NONE',  ( -136.4994460260996902, -31.11111111111111427, 27.86436879316430648 ) ) ;
#9218=ORIENTED_EDGE ( 'NONE', *, *, #9967, .T. ) ;
#9222=VERTEX_POINT ( 'NONE', #2747 ) ;
#9226=DIRECTION ( 'NONE',  ( 1.000000000000000000, 3.320906611023727849E-16, 0.000000000000000000 ) ) ;
#9233=CARTESIAN_POINT ( 'NONE',  ( -95.44915936929146483, -116.0550301922269085, 32.61437126001344922 ) ) ;
#9234=FACE_OUTER_BOUND ( 'NONE', #18816, .T. ) ;
#9235=CARTESIAN_POINT ( 'NONE',  ( 71.18887634719571622, -147.8252249328912740, 39.99999999999999289 ) ) ;
#9237=CARTESIAN_POINT ( 'NONE',  ( -134.9140359355702685, -65.56103033672289371, 6.267746957543315567 ) ) ;
#9239=CARTESIAN_POINT ( 'NONE',  ( 128.7754324793921228, -76.93177152330439128, -7.719765474015907181 ) ) ;
#9240=CIRCLE ( 'NONE', #4678, 10.00000000000000888 ) ;
#9243=FACE_OUTER_BOUND ( 'NONE', #14368, .T. ) ;
#9244=CARTESIAN_POINT ( 'NONE',  ( -132.0512179319685515, -87.77725330520023306, 39.71072694138295844 ) ) ;
#9246=ADVANCED_FACE ( 'NONE', ( #14912 ), #4172, .F. ) ;
#9252=EDGE_CURVE ( 'NONE', #6551, #5955, #9313, .T. ) ;
#9260=DIRECTION ( 'NONE',  ( -1.000000000000000000, 0.000000000000000000, 0.000000000000000000 ) ) ;
#9270=EDGE_CURVE ( 'NONE', #15648, #7108, #9973, .T. ) ;
#9271=CARTESIAN_POINT ( 'NONE',  ( 134.9866372717144998, -65.41115948451921724, 32.98563192608333594 ) ) ;
#9279=EDGE_CURVE ( 'NONE', #19819, #6720, #11723, .T. ) ;
#9296=VECTOR ( 'NONE', #11519, 1000.000000000000000 ) ;
#9297=DIRECTION ( 'NONE',  ( 0.000000000000000000, 0.000000000000000000, 1.000000000000000000 ) ) ;
#9299=CARTESIAN_POINT ( 'NONE',  ( -76.58875299708743967, 117.1931663892607958, 15.45866710248154519 ) ) ;
#9301=EDGE_LOOP ( 'NONE', ( #18979, #15667, #3502, #19728 ) ) ;
#9303=ORIENTED_EDGE ( 'NONE', *, *, #19544, .T. ) ;
#9306=AXIS2_PLACEMENT_3D ( 'NONE', #1100, #12039, #12350 ) ;
#9308=CARTESIAN_POINT ( 'NONE',  ( -139.4006145564613917, 50.16213250608596042, -22.20134617928383491 ) ) ;
#9311=CARTESIAN_POINT ( 'NONE',  ( 99.76899065921492138, -130.8788316638307379, 3.647911195597622225 ) ) ;
#9313=CIRCLE ( 'NONE', #17168, 15.91767397667354444 ) ;
#9319=DIRECTION ( 'NONE',  ( -1.000000000000000000, 0.000000000000000000, 0.000000000000000000 ) ) ;
#9321=CARTESIAN_POINT ( 'NONE',  ( 98.17258311761688105, -133.0662226711789629, 33.62401363155364464 ) ) ;
#9322=VERTEX_POINT ( 'NONE', #13885 ) ;
#9328=AXIS2_PLACEMENT_3D ( 'NONE', #11449, #510, #6753 ) ;
#9330=CARTESIAN_POINT ( 'NONE',  ( -98.50852301078386120, -132.6154683359945636, 5.603543560907854548 ) ) ;
#9332=ORIENTED_EDGE ( 'NONE', *, *, #9355, .T. ) ;
#9336=CARTESIAN_POINT ( 'NONE',  ( -85.13411715130405355, -123.5004392096852683, 41.04246620030852455 ) ) ;
#9337=DIRECTION ( 'NONE',  ( 0.000000000000000000, 0.000000000000000000, 1.000000000000000000 ) ) ;
#9342=CARTESIAN_POINT ( 'NONE',  ( 132.4144148199947324, -86.21736781322083232, 0.5493819109983639759 ) ) ;
#9345=CARTESIAN_POINT ( 'NONE',  ( -133.2581445365307786, -82.18041427990793579, 38.38389406139176430 ) ) ;
#9354=ORIENTED_EDGE ( 'NONE', *, *, #9409, .F. ) ;
#9355=EDGE_CURVE ( 'NONE', #9886, #9122, #2274, .T. ) ;
#9356=CARTESIAN_POINT ( 'NONE',  ( -143.9003822582011765, -15.47344326723975882, 13.71750472807623211 ) ) ;
#9361=ORIENTED_EDGE ( 'NONE', *, *, #3614, .T. ) ;
#9362=CARTESIAN_POINT ( 'NONE',  ( -32.50000000000000000, 0.000000000000000000, -40.00000000000000000 ) ) ;
#9368=AXIS2_PLACEMENT_3D ( 'NONE', #19412, #5589, #10097 ) ;
#9375=AXIS2_PLACEMENT_3D ( 'NONE', #10839, #20058, #9319 ) ;
#9376=VERTEX_POINT ( 'NONE', #18495 ) ;
#9379=CARTESIAN_POINT ( 'NONE',  ( 0.000000000000000000, 0.000000000000000000, -105.0000000000000142 ) ) ;
#9381=ORIENTED_EDGE ( 'NONE', *, *, #6132, .T. ) ;
#9385=CARTESIAN_POINT ( 'NONE',  ( -99.30949456653213758, -131.5229532012209290, 35.79133943910348847 ) ) ;
#9390=CARTESIAN_POINT ( 'NONE',  ( -189.9999999999988916, 265.0000000000000000, 12.50000000000027178 ) ) ;
#9393=CARTESIAN_POINT ( 'NONE',  ( -78.17584345766714193, 126.7527627678825581, -19.23956518957315964 ) ) ;
#9396=EDGE_CURVE ( 'NONE', #17652, #7267, #16968, .T. ) ;
#9398=DIRECTION ( 'NONE',  ( 1.000000000000000000, 0.000000000000000000, 0.000000000000000000 ) ) ;
#9403=CIRCLE ( 'NONE', #8083, 77.50000000000000000 ) ;
#9404=ORIENTED_EDGE ( 'NONE', *, *, #8667, .T. ) ;
#9405=DIRECTION ( 'NONE',  ( 0.000000000000000000, 0.000000000000000000, 1.000000000000000000 ) ) ;
#9409=EDGE_CURVE ( 'NONE', #5147, #13667, #11079, .T. ) ;
#9413=CARTESIAN_POINT ( 'NONE',  ( 97.91442649640829643, -133.4097810207084081, 7.055758473159548849 ) ) ;
#9416=EDGE_CURVE ( 'NONE', #11180, #4182, #1622, .T. ) ;
#9417=AXIS2_PLACEMENT_3D ( 'NONE', #3745, #2421, #578 ) ;
#9418=DIRECTION ( 'NONE',  ( -0.000000000000000000, -0.000000000000000000, 1.000000000000000000 ) ) ;
#9419=CIRCLE ( 'NONE', #11046, 7.500000000000007105 ) ;
#9421=AXIS2_PLACEMENT_3D ( 'NONE', #13895, #1321, #13794 ) ;
#9425=LINE ( 'NONE', #12793, #2242 ) ;
#9426=CARTESIAN_POINT ( 'NONE',  ( 87.54876440221090661, -121.8053786065073467, 44.23084021805906474 ) ) ;
#9428=DIRECTION ( 'NONE',  ( 0.000000000000000000, 0.000000000000000000, 1.000000000000000000 ) ) ;
#9435=CIRCLE ( 'NONE', #10389, 40.00000000000000711 ) ;
#9436=ORIENTED_EDGE ( 'NONE', *, *, #19765, .T. ) ;
#9438=CARTESIAN_POINT ( 'NONE',  ( 126.5370453525553671, 80.55045718954890788, 39.99999999999999289 ) ) ;
#9442=DIRECTION ( 'NONE',  ( 1.000000000000000000, 0.000000000000000000, 0.000000000000000000 ) ) ;
#9443=CARTESIAN_POINT ( 'NONE',  ( -109.9999999999983515, 275.0000000000000000, 85.00000000000001421 ) ) ;
#9445=CARTESIAN_POINT ( 'NONE',  ( -101.4356266330729426, -128.4750511900866456, 37.97853139149559354 ) ) ;
#9447=CARTESIAN_POINT ( 'NONE',  ( -124.9072147131054180, 63.35168546091732367, 36.73018266758872130 ) ) ;
#9448=DIRECTION ( 'NONE',  ( 0.000000000000000000, -0.000000000000000000, 1.000000000000000000 ) ) ;
#9454=CARTESIAN_POINT ( 'NONE',  ( -126.6625757374809638, -80.35588318643578987, 49.09314554429377608 ) ) ;
#9460=ORIENTED_EDGE ( 'NONE', *, *, #7928, .F. ) ;
#9463=AXIS2_PLACEMENT_3D ( 'NONE', #10989, #15291, #6098 ) ;
#9476=CARTESIAN_POINT ( 'NONE',  ( 133.2712073793125569, -68.96827650305596080, 29.99999999999999645 ) ) ;
#9477=CARTESIAN_POINT ( 'NONE',  ( 131.2500704209023183, -90.93860529234677870, 39.99999999999998579 ) ) ;
#9493=AXIS2_PLACEMENT_3D ( 'NONE', #1955, #17309, #14330 ) ;
#9494=CARTESIAN_POINT ( 'NONE',  ( -141.8714406926360994, -48.70825716237271763, 49.99999999999999289 ) ) ;
#9495=CARTESIAN_POINT ( 'NONE',  ( -110.0000000000000142, 265.0000000000000000, 5.000000000000000888 ) ) ;
#9496=ORIENTED_EDGE ( 'NONE', *, *, #2535, .F. ) ;
#9497=CARTESIAN_POINT ( 'NONE',  ( -110.0000000000000000, 88.56916956954178488, -34.99999999999998579 ) ) ;
#9498=DIRECTION ( 'NONE',  ( -0.000000000000000000, -1.000000000000000000, -0.000000000000000000 ) ) ;
#9500=CARTESIAN_POINT ( 'NONE',  ( -52.50000000000000000, -2.094888803305880013E-13, -105.0000000000000142 ) ) ;
#9503=CARTESIAN_POINT ( 'NONE',  ( 98.63291732527038391, -113.0135401039851217, 49.87660771364959089 ) ) ;
#9504=EDGE_LOOP ( 'NONE', ( #2337, #12892, #9404, #19733, #14105 ) ) ;
#9505=EDGE_CURVE ( 'NONE', #12416, #8371, #10105, .T. ) ;
#9509=AXIS2_PLACEMENT_3D ( 'NONE', #9818, #16471, #5322 ) ;
#9510=ORIENTED_EDGE ( 'NONE', *, *, #9102, .F. ) ;
#9514=EDGE_CURVE ( 'NONE', #14876, #1151, #9991, .T. ) ;
#9527=CARTESIAN_POINT ( 'NONE',  ( 152.4599531637113330, -36.50981547336952104, 39.99999999999999289 ) ) ;
#9528=CARTESIAN_POINT ( 'NONE',  ( 85.14104117559514862, -123.4951580371803885, 41.03646238235858590 ) ) ;
#9529=ORIENTED_EDGE ( 'NONE', *, *, #18154, .F. ) ;
#9533=CARTESIAN_POINT ( 'NONE',  ( -92.96950599336983601, 117.7174478370289279, 41.20115630078900182 ) ) ;
#9539=LINE ( 'NONE', #26, #11722 ) ;
#9541=EDGE_CURVE ( 'NONE', #16770, #16122, #3846, .T. ) ;
#9545=CARTESIAN_POINT ( 'NONE',  ( 130.1925331961320182, -74.50863253846080170, 46.29641651522450729 ) ) ;
#9546=CARTESIAN_POINT ( 'NONE',  ( -84.61443574189109995, -123.8565353992701858, 40.13652017786752424 ) ) ;
#9548=DIRECTION ( 'NONE',  ( 1.000000000000000000, 0.000000000000000000, 0.000000000000000000 ) ) ;
#9554=CARTESIAN_POINT ( 'NONE',  ( -131.8028587768753823, -71.61967917966801167, 44.00945860701838086 ) ) ;
#9556=CARTESIAN_POINT ( 'NONE',  ( 67.50000000000000000, 6.284666409917639535E-13, -100.0000000000000000 ) ) ;
#9557=VECTOR ( 'NONE', #7503, 1000.000000000000000 ) ;
#9558=AXIS2_PLACEMENT_3D ( 'NONE', #15814, #9769, #18994 ) ;
#9564=CARTESIAN_POINT ( 'NONE',  ( -142.4959821499880945, -17.39774326699847151, -8.008195377800351622 ) ) ;
#9571=CARTESIAN_POINT ( 'NONE',  ( 0.000000000000000000, 0.000000000000000000, 49.99999999999999289 ) ) ;
#9573=CARTESIAN_POINT ( 'NONE',  ( 0.000000000000000000, 0.000000000000000000, 49.99999999999999289 ) ) ;
#9576=CARTESIAN_POINT ( 'NONE',  ( 134.6268015237237705, -73.65543454550100932, 32.58577753858380532 ) ) ;
#9577=CARTESIAN_POINT ( 'NONE',  ( 134.2328839869800845, -76.48032294689464550, 35.58107860435188741 ) ) ;
#9587=CARTESIAN_POINT ( 'NONE',  ( -97.49999999999998579, -133.9542832461881687, 30.00000000000000000 ) ) ;
#9588=DIRECTION ( 'NONE',  ( 0.000000000000000000, 1.000000000000000000, 0.000000000000000000 ) ) ;
#9593=ORIENTED_EDGE ( 'NONE', *, *, #18942, .T. ) ;
#9601=CARTESIAN_POINT ( 'NONE',  ( 82.53664710575304753, -125.2505858294166501, 34.62610835550965049 ) ) ;
#9609=CARTESIAN_POINT ( 'NONE',  ( -140.7359356944403430, 47.72516008681479605, -20.67287135512269813 ) ) ;
#9612=VERTEX_POINT ( 'NONE', #3749 ) ;
#9617=CYLINDRICAL_SURFACE ( 'NONE', #17370, 7.500000000000020428 ) ;
#9629=CARTESIAN_POINT ( 'NONE',  ( -70.58469675536078114, 132.3548539117337270, 11.82943511394700487 ) ) ;
#9636=CARTESIAN_POINT ( 'NONE',  ( -100.6828170698202172, -129.5784119885790915, 2.652022552455725268 ) ) ;
#9637=CARTESIAN_POINT ( 'NONE',  ( -149.9875400927184046, 2.232080205859953370, 6.152641185304041471 ) ) ;
#9638=ORIENTED_EDGE ( 'NONE', *, *, #1138, .T. ) ;
#9642=CARTESIAN_POINT ( 'NONE',  ( 131.9010376021428783, -71.43117396976204247, 43.79329771262451487 ) ) ;
#9644=CARTESIAN_POINT ( 'NONE',  ( -120.6301673961016547, 71.05871668019251786, 38.35088066313576149 ) ) ;
#9649=CYLINDRICAL_SURFACE ( 'NONE', #6715, 42.50000000000000000 ) ;
#9654=CIRCLE ( 'NONE', #11272, 10.00000000000000888 ) ;
#9662=CARTESIAN_POINT ( 'NONE',  ( -176.1792632384392050, -186.5724904703759535, 40.00000000000000000 ) ) ;
#9667=DIRECTION ( 'NONE',  ( -0.000000000000000000, -0.000000000000000000, 1.000000000000000000 ) ) ;
#9671=CARTESIAN_POINT ( 'NONE',  ( 100.6828170698202314, -129.5784119885790346, 37.34797744754428095 ) ) ;
#9674=CARTESIAN_POINT ( 'NONE',  ( 129.7881937802467860, -75.28665481069999998, 39.48948438905874525 ) ) ;
#9675=CARTESIAN_POINT ( 'NONE',  ( 133.8332678793154287, -78.98710468785299099, 37.05447038645785085 ) ) ;
#9677=EDGE_LOOP ( 'NONE', ( #9354, #3325 ) ) ;
#9679=ORIENTED_EDGE ( 'NONE', *, *, #12607, .T. ) ;
#9682=ORIENTED_EDGE ( 'NONE', *, *, #6449, .F. ) ;
#9687=ORIENTED_EDGE ( 'NONE', *, *, #11828, .F. ) ;
#9694=CARTESIAN_POINT ( 'NONE',  ( -71.18887634719365565, -147.8252249328922687, 39.99999999999999289 ) ) ;
#9696=AXIS2_PLACEMENT_3D ( 'NONE', #16374, #19341, #17713 ) ;
#9698=CYLINDRICAL_SURFACE ( 'NONE', #14709, 150.0000000000000284 ) ;
#9699=CARTESIAN_POINT ( 'NONE',  ( 82.79607015190580910, -125.0792639210692982, 35.66528578544987482 ) ) ;
#9713=CARTESIAN_POINT ( 'NONE',  ( 101.0196388379316659, 100.9199429146863167, 39.99999999999999289 ) ) ;
#9715=DIRECTION ( 'NONE',  ( 0.000000000000000000, 0.000000000000000000, -1.000000000000000000 ) ) ;
#9719=CARTESIAN_POINT ( 'NONE',  ( 159.9599531637113330, -36.50981547336952104, 49.99999999999999289 ) ) ;
#9728=EDGE_LOOP ( 'NONE', ( #4049, #18983 ) ) ;
#9733=CARTESIAN_POINT ( 'NONE',  ( -126.6376994899158177, 80.42828178209725820, 41.40291032811695970 ) ) ;
#9739=EDGE_CURVE ( 'NONE', #7332, #5360, #9130, .T. ) ;
#9744=DIRECTION ( 'NONE',  ( 0.000000000000000000, 0.000000000000000000, 1.000000000000000000 ) ) ;
#9748=ORIENTED_EDGE ( 'NONE', *, *, #1015, .T. ) ;
#9751=CIRCLE ( 'NONE', #1966, 10.00000000000000888 ) ;
#9753=AXIS2_PLACEMENT_3D ( 'NONE', #18830, #19035, #7765 ) ;
#9757=ORIENTED_EDGE ( 'NONE', *, *, #15009, .T. ) ;
#9759=CARTESIAN_POINT ( 'NONE',  ( 167.4599531637113330, -36.50981547336952104, 39.99999999999999289 ) ) ;
#9760=EDGE_CURVE ( 'NONE', #2667, #5578, #15001, .T. ) ;
#9764=AXIS2_PLACEMENT_3D ( 'NONE', #977, #15609, #1597 ) ;
#9767=DIRECTION ( 'NONE',  ( -0.000000000000000000, 0.000000000000000000, -1.000000000000000000 ) ) ;
#9769=DIRECTION ( 'NONE',  ( 0.000000000000000000, 0.000000000000000000, 1.000000000000000000 ) ) ;
#9771=CARTESIAN_POINT ( 'NONE',  ( 101.1753893487742175, -128.8598102521083604, 37.76972961429584075 ) ) ;
#9784=CARTESIAN_POINT ( 'NONE',  ( 159.9599531637113330, -36.50981547336952104, 39.99999999999999289 ) ) ;
#9785=CARTESIAN_POINT ( 'NONE',  ( -98.51475352695842957, -132.6070668284233136, 34.40940853324102733 ) ) ;
#9788=ORIENTED_EDGE ( 'NONE', *, *, #12837, .F. ) ;
#9789=DIRECTION ( 'NONE',  ( 0.000000000000000000, 0.000000000000000000, 1.000000000000000000 ) ) ;
#9792=CARTESIAN_POINT ( 'NONE',  ( -99.16663380741609046, 102.1467062937776120, -33.51457741426627734 ) ) ;
#9793=CARTESIAN_POINT ( 'NONE',  ( 15.91767397667355155, 149.1530343478547422, 49.99999999999999289 ) ) ;
#9795=CIRCLE ( 'NONE', #962, 7.500000000000002665 ) ;
#9798=LINE ( 'NONE', #17985, #5798 ) ;
#9799=PLANE ( 'NONE',  #3682 ) ;
#9801=CARTESIAN_POINT ( 'NONE',  ( 91.69714670201405227, -118.7099181436120290, 47.50740515561367516 ) ) ;
#9803=CARTESIAN_POINT ( 'NONE',  ( 60.00000000000000711, 6.284666409917639535E-13, -100.0000000000000000 ) ) ;
#9807=DIRECTION ( 'NONE',  ( 0.000000000000000000, 0.000000000000000000, 1.000000000000000000 ) ) ;
#9811=LINE ( 'NONE', #11241, #7963 ) ;
#9817=CARTESIAN_POINT ( 'NONE',  ( 102.6638558517306734, -126.6149147318370609, 1.229818221047174420 ) ) ;
#9818=CARTESIAN_POINT ( 'NONE',  ( 159.9599531637113330, -36.50981547336952104, 49.99999999999999289 ) ) ;
#9821=CARTESIAN_POINT ( 'NONE',  ( -56.84754764479025368, -154.7316448359455308, 39.99999999999999289 ) ) ;
#9823=AXIS2_PLACEMENT_3D ( 'NONE', #5718, #20105, #1598 ) ;
#9824=CARTESIAN_POINT ( 'NONE',  ( 96.60517994339912207, -114.8199649187202880, 36.24366236571611921 ) ) ;
#9827=CARTESIAN_POINT ( 'NONE',  ( -72.91900756452172061, 131.0832496385607158, -10.00000000000000178 ) ) ;
#9828=ORIENTED_EDGE ( 'NONE', *, *, #16624, .F. ) ;
#9830=ORIENTED_EDGE ( 'NONE', *, *, #5175, .T. ) ;
#9839=CARTESIAN_POINT ( 'NONE',  ( -97.58443926496194365, -133.8443912861145009, 8.507479503170321422 ) ) ;
#9844=PLANE ( 'NONE',  #7580 ) ;
#9849=CARTESIAN_POINT ( 'NONE',  ( -136.2592242320518210, 27.06617804205124500, -18.18972273333671907 ) ) ;
#9851=EDGE_CURVE ( 'NONE', #13843, #12327, #7516, .T. ) ;
#9853=VERTEX_POINT ( 'NONE', #17247 ) ;
#9854=APPLICATION_CONTEXT ( 'automotive_design' ) ;
#9866=FACE_BOUND ( 'NONE', #10441, .T. ) ;
#9867=AXIS2_PLACEMENT_3D ( 'NONE', #12502, #3210, #12911 ) ;
#9870=VERTEX_POINT ( 'NONE', #4874 ) ;
#9879=AXIS2_PLACEMENT_3D ( 'NONE', #4861, #17344, #11772 ) ;
#9882=CARTESIAN_POINT ( 'NONE',  ( -176.1792632384392050, -186.5724904703759535, 10.00000000000000178 ) ) ;
#9884=DIRECTION ( 'NONE',  ( 0.000000000000000000, 1.000000000000000000, 0.000000000000000000 ) ) ;
#9886=VERTEX_POINT ( 'NONE', #9362 ) ;
#9888=AXIS2_PLACEMENT_3D ( 'NONE', #8492, #10028, #19536 ) ;
#9889=DIRECTION ( 'NONE',  ( -0.000000000000000000, -0.000000000000000000, -1.000000000000000000 ) ) ;
#9891=ADVANCED_FACE ( 'NONE', ( #4768 ), #13857, .T. ) ;
#9893=ORIENTED_EDGE ( 'NONE', *, *, #4142, .F. ) ;
#9894=EDGE_CURVE ( 'NONE', #10980, #2833, #17146, .T. ) ;
#9895=CYLINDRICAL_SURFACE ( 'NONE', #13258, 7.500000000000007105 ) ;
#9896=CARTESIAN_POINT ( 'NONE',  ( -15.91767397667354800, 149.1530343478547422, 39.99999999999999289 ) ) ;
#9898=CARTESIAN_POINT ( 'NONE',  ( -134.5432410141372941, -66.31847138156592791, 36.21250959424132532 ) ) ;
#9900=VECTOR ( 'NONE', #4994, 1000.000000000000114 ) ;
#9903=CARTESIAN_POINT ( 'NONE',  ( -75.56543138647906233, 117.8553135366936147, -1.280227956710139781 ) ) ;
#9909=ORIENTED_EDGE ( 'NONE', *, *, #5050, .T. ) ;
#9910=CARTESIAN_POINT ( 'NONE',  ( -110.0000000000000142, 275.0000000000000000, 5.000000000000000888 ) ) ;
#9915=EDGE_CURVE ( 'NONE', #11866, #11373, #3021, .T. ) ;
#9922=EDGE_CURVE ( 'NONE', #12362, #4372, #14574, .T. ) ;
#9929=CARTESIAN_POINT ( 'NONE',  ( 103.5930306437996364, -125.1526588151300814, 39.21025145423357827 ) ) ;
#9931=DIRECTION ( 'NONE',  ( 0.9009688679024154823, 0.4338837391175657809, 0.000000000000000000 ) ) ;
#9937=AXIS2_PLACEMENT_3D ( 'NONE', #9443, #10761, #7690 ) ;
#9942=ORIENTED_EDGE ( 'NONE', *, *, #5050, .F. ) ;
#9945=CARTESIAN_POINT ( 'NONE',  ( -95.72167172977317762, -116.1306513017113957, 9.110179581664221260 ) ) ;
#9947=CARTESIAN_POINT ( 'NONE',  ( -139.3985923533142284, -13.22154594654577231, 24.00007470227639317 ) ) ;
#9953=DIRECTION ( 'NONE',  ( -0.000000000000000000, -1.000000000000000000, -0.000000000000000000 ) ) ;
#9957=VECTOR ( 'NONE', #13829, 1000.000000000000000 ) ;
#9960=ORIENTED_EDGE ( 'NONE', *, *, #16466, .F. ) ;
#9967=EDGE_CURVE ( 'NONE', #269, #13358, #5271, .T. ) ;
#9969=CARTESIAN_POINT ( 'NONE',  ( -15.91767397667354800, 164.0736214083062805, 49.99999999999999289 ) ) ;
#9970=LINE ( 'NONE', #5276, #394 ) ;
#9971=DIRECTION ( 'NONE',  ( 0.000000000000000000, 0.000000000000000000, 1.000000000000000000 ) ) ;
#9972=CARTESIAN_POINT ( 'NONE',  ( 104.1536737562094288, -124.2508859553631311, 39.42722059334807483 ) ) ;
#9973=CIRCLE ( 'NONE', #1140, 7.500000000000007105 ) ;
#9977=ORIENTED_EDGE ( 'NONE', *, *, #7383, .F. ) ;
#9987=FACE_BOUND ( 'NONE', #14707, .T. ) ;
#9988=CARTESIAN_POINT ( 'NONE',  ( 106.6880305650188063, 105.4403344747995845, 49.99999999999999289 ) ) ;
#9989=ORIENTED_EDGE ( 'NONE', *, *, #11769, .T. ) ;
#9991=LINE ( 'NONE', #11524, #5211 ) ;
#9996=FACE_OUTER_BOUND ( 'NONE', #5324, .T. ) ;
#10002=VECTOR ( 'NONE', #5923, 1000.000000000000000 ) ;
#10005=EDGE_LOOP ( 'NONE', ( #7833, #5266, #15276, #12876 ) ) ;
#10007=ORIENTED_EDGE ( 'NONE', *, *, #19711, .T. ) ;
#10020=CARTESIAN_POINT ( 'NONE',  ( 175.8776271403848739, -36.50981547336952104, 39.99999999999999289 ) ) ;
#10022=CARTESIAN_POINT ( 'NONE',  ( 0.000000000000000000, 0.000000000000000000, 39.99999999999999289 ) ) ;
#10027=CARTESIAN_POINT ( 'NONE',  ( 0.000000000000000000, 60.00000000000000000, -100.0000000000000000 ) ) ;
#10028=DIRECTION ( 'NONE',  ( 0.000000000000000000, 0.000000000000000000, 1.000000000000000000 ) ) ;
#10029=CIRCLE ( 'NONE', #9368, 7.500000000000001776 ) ;
#10034=EDGE_CURVE ( 'NONE', #13358, #5734, #3583, .T. ) ;
#10044=EDGE_LOOP ( 'NONE', ( #15687, #9460, #12967, #16777 ) ) ;
#10047=CARTESIAN_POINT ( 'NONE',  ( -97.83472796452241482, -133.5146506974499232, 7.427686840538095581 ) ) ;
#10049=B_SPLINE_CURVE_WITH_KNOTS ( 'NONE', 3,
 ( #3643, #9477, #12839, #19097, #266, #1700, #11311, #17259, #7931, #14183, #3238, #9675, #15823, #6716, #9577, #8139, #1805, #17568, #3441, #6520, #6316, #12742, #10999, #19001 ),
 .UNSPECIFIED., .F., .F.,
 ( 4, 2, 2, 2, 2, 2, 2, 2, 2, 2, 2, 4 ),
 ( 0.000000000000000000, 0.002919511036912160896, 0.005839022073824321792, 0.008758533110736483121, 0.01167804414764864358, 0.01313779966610474463, 0.01459755518456084568, 0.01751706622147301481, 0.01897682173992911239, 0.02043657725838521344, 0.02189633277684131102, 0.02335608829529741207 ),
 .UNSPECIFIED. ) ;
#10050=CARTESIAN_POINT ( 'NONE',  ( -84.97262318625999455, -123.6115503146182277, -0.7768402190473889801 ) ) ;
#10051=LINE ( 'NONE', #18217, #10257 ) ;
#10066=DIRECTION ( 'NONE',  ( 0.000000000000000000, 0.000000000000000000, 1.000000000000000000 ) ) ;
#10067=LINE ( 'NONE', #19571, #15646 ) ;
#10070=DIRECTION ( 'NONE',  ( 1.000000000000000000, 0.000000000000000000, 0.000000000000000000 ) ) ;
#10071=CARTESIAN_POINT ( 'NONE',  ( 133.1725405177770369, -69.15900471361744906, 7.877401435139040231 ) ) ;
#10076=PRODUCT_DEFINITION_CONTEXT ( 'detailed design', #6727, 'design' ) ;
#10077=ORIENTED_EDGE ( 'NONE', *, *, #9922, .F. ) ;
#10081=EDGE_LOOP ( 'NONE', ( #14813, #15880, #8555, #16151 ) ) ;
#10082=EDGE_CURVE ( 'NONE', #870, #12020, #8630, .T. ) ;
#10085=CARTESIAN_POINT ( 'NONE',  ( 15.91767397667354800, 164.0736214083062805, 49.99999999999999289 ) ) ;
#10088=AXIS2_PLACEMENT_3D ( 'NONE', #16639, #18269, #13441 ) ;
#10097=DIRECTION ( 'NONE',  ( -1.000000000000000000, 0.000000000000000000, 0.000000000000000000 ) ) ;
#10105=CIRCLE ( 'NONE', #14675, 7.500000000000003553 ) ;
#10106=ORIENTED_EDGE ( 'NONE', *, *, #9145, .F. ) ;
#10114=CARTESIAN_POINT ( 'NONE',  ( -82.17872144123516875, -125.4856950968008817, 32.52944088431316061 ) ) ;
#10122=CARTESIAN_POINT ( 'NONE',  ( 97.49999999999997158, -133.9542832461880835, 9.515056863104252471 ) ) ;
#10127=CYLINDRICAL_SURFACE ( 'NONE', #18730, 10.00000000000000888 ) ;
#10129=CARTESIAN_POINT ( 'NONE',  ( 99.70874217756774271, -112.0725815587889969, -9.999999999999996447 ) ) ;
#10131=ORIENTED_EDGE ( 'NONE', *, *, #8836, .F. ) ;
#10136=EDGE_CURVE ( 'NONE', #5586, #5786, #10423, .T. ) ;
#10139=CARTESIAN_POINT ( 'NONE',  ( 107.5000000000000284, -118.5063289449133492, -3.469446951953614189E-15 ) ) ;
#10140=CARTESIAN_POINT ( 'NONE',  ( -99.45845524092749201, -131.3126558323500319, 4.053310392242657656 ) ) ;
#10142=AXIS2_PLACEMENT_3D ( 'NONE', #1851, #12890, #19145 ) ;
#10154=CARTESIAN_POINT ( 'NONE',  ( 135.7779226595531270, 102.2982297021113141, 49.99999999999999289 ) ) ;
#10157=VECTOR ( 'NONE', #1367, 1000.000000000000000 ) ;
#10159=ORIENTED_EDGE ( 'NONE', *, *, #7505, .T. ) ;
#10169=CARTESIAN_POINT ( 'NONE',  ( 134.3401481871931651, -66.72943863802692022, 2.767325007884418930 ) ) ;
#10170=LINE ( 'NONE', #5468, #18997 ) ;
#10175=EDGE_LOOP ( 'NONE', ( #8140, #6113, #15851, #780 ) ) ;
#10178=DIRECTION ( 'NONE',  ( 0.000000000000000000, 0.000000000000000000, -1.000000000000000000 ) ) ;
#10183=ORIENTED_EDGE ( 'NONE', *, *, #3271, .F. ) ;
#10184=AXIS2_PLACEMENT_3D ( 'NONE', #4959, #11074, #9744 ) ;
#10190=CARTESIAN_POINT ( 'NONE',  ( -134.3942145021295005, -75.36533733386917788, 5.353827179577918649 ) ) ;
#10192=DIRECTION ( 'NONE',  ( -1.000000000000000000, 0.000000000000000000, 0.000000000000000000 ) ) ;
#10195=DIRECTION ( 'NONE',  ( 0.000000000000000000, 1.000000000000000000, 0.000000000000000000 ) ) ;
#10199=ORIENTED_EDGE ( 'NONE', *, *, #3016, .T. ) ;
#10201=ORIENTED_EDGE ( 'NONE', *, *, #5390, .F. ) ;
#10203=VECTOR ( 'NONE', #7780, 1000.000000000000000 ) ;
#10212=EDGE_CURVE ( 'NONE', #11724, #10980, #9795, .T. ) ;
#10217=CARTESIAN_POINT ( 'NONE',  ( 98.63424005417277840, -113.0189783045208287, -9.902513086295204658 ) ) ;
#10224=VERTEX_POINT ( 'NONE', #7693 ) ;
#10228=ADVANCED_FACE ( 'NONE', ( #1255 ), #18447, .T. ) ;
#10230=DIRECTION ( 'NONE',  ( 0.3427509529624095941, 0.9394263059140722794, -0.000000000000000000 ) ) ;
#10231=FACE_OUTER_BOUND ( 'NONE', #5165, .T. ) ;
#10234=CARTESIAN_POINT ( 'NONE',  ( -101.4383890160140425, -128.4709723833222768, 2.019278167221355780 ) ) ;
#10236=EDGE_CURVE ( 'NONE', #16933, #8290, #16810, .T. ) ;
#10237=CARTESIAN_POINT ( 'NONE',  ( -138.8107028532319873, -18.39471665163164715, 24.88022817150739385 ) ) ;
#10241=CYLINDRICAL_SURFACE ( 'NONE', #9110, 7.500000000000000000 ) ;
#10245=LINE ( 'NONE', #16503, #12503 ) ;
#10247=EDGE_LOOP ( 'NONE', ( #2357, #9496, #3250, #13021 ) ) ;
#10250=ORIENTED_EDGE ( 'NONE', *, *, #3523, .F. ) ;
#10251=EDGE_CURVE ( 'NONE', #11005, #11485, #4640, .T. ) ;
#10256=DIRECTION ( 'NONE',  ( -1.000000000000000000, -1.613511099790691498E-16, 0.000000000000000000 ) ) ;
#10257=VECTOR ( 'NONE', #3805, 1000.000000000000000 ) ;
#10262=ADVANCED_FACE ( 'NONE', ( #6076, #12786 ), #15584, .T. ) ;
#10268=ORIENTED_EDGE ( 'NONE', *, *, #14683, .F. ) ;
#10274=ORIENTED_EDGE ( 'NONE', *, *, #8214, .F. ) ;
#10282=CYLINDRICAL_SURFACE ( 'NONE', #6735, 140.0000000000000284 ) ;
#10284=ORIENTED_EDGE ( 'NONE', *, *, #18529, .F. ) ;
#10285=CYLINDRICAL_SURFACE ( 'NONE', #10088, 15.91767397667354089 ) ;
#10289=DIRECTION ( 'NONE',  ( -0.7406645559057076778, -0.6718750000000006661, -0.000000000000000000 ) ) ;
#10290=DIRECTION ( 'NONE',  ( -0.000000000000000000, -0.000000000000000000, 1.000000000000000000 ) ) ;
#10297=ORIENTED_EDGE ( 'NONE', *, *, #8528, .T. ) ;
#10299=DIRECTION ( 'NONE',  ( 0.000000000000000000, 0.000000000000000000, 1.000000000000000000 ) ) ;
#10302=DIRECTION ( 'NONE',  ( 0.000000000000000000, 0.000000000000000000, 1.000000000000000000 ) ) ;
#10311=CARTESIAN_POINT ( 'NONE',  ( 84.32000978867640129, -124.0571233621914899, 0.4179024135772307358 ) ) ;
#10319=AXIS2_PLACEMENT_3D ( 'NONE', #10700, #13671, #19915 ) ;
#10323=AXIS2_PLACEMENT_3D ( 'NONE', #1829, #8061, #14312 ) ;
#10327=CARTESIAN_POINT ( 'NONE',  ( -106.3852469178145412, -120.5001569748711461, 0.04619868349364349841 ) ) ;
#10328=CARTESIAN_POINT ( 'NONE',  ( -136.4994460260996902, -31.11111111111111427, 27.86436879316430648 ) ) ;
#10336=ADVANCED_FACE ( 'NONE', ( #16913 ), #4876, .T. ) ;
#10346=EDGE_LOOP ( 'NONE', ( #10106, #7527, #8401, #4187 ) ) ;
#10349=CARTESIAN_POINT ( 'NONE',  ( 107.5000000000000284, -199.9999999999999716, 0.000000000000000000 ) ) ;
#10350=CARTESIAN_POINT ( 'NONE',  ( -99.33980890132491481, -112.3956798702028692, 39.16385526563716724 ) ) ;
#10352=DIRECTION ( 'NONE',  ( -1.000000000000000000, 0.000000000000000000, 0.000000000000000000 ) ) ;
#10353=FACE_OUTER_BOUND ( 'NONE', #2505, .T. ) ;
#10354=CARTESIAN_POINT ( 'NONE',  ( -126.4587173007283809, -80.71184697946637243, -1.017284155395590250 ) ) ;
#10357=EDGE_CURVE ( 'NONE', #3818, #7363, #3971, .T. ) ;
#10360=CARTESIAN_POINT ( 'NONE',  ( -135.1060089016710037, -65.16414933582423430, 31.52442972994579051 ) ) ;
#10362=AXIS2_PLACEMENT_3D ( 'NONE', #14396, #15935, #19109 ) ;
#10369=DIRECTION ( 'NONE',  ( 0.000000000000000000, 0.000000000000000000, -1.000000000000000000 ) ) ;
#10371=EDGE_LOOP ( 'NONE', ( #4991, #12289 ) ) ;
#10372=DIRECTION ( 'NONE',  ( 0.4338837391175525693, 0.9009688679024216995, 0.000000000000000000 ) ) ;
#10376=FACE_OUTER_BOUND ( 'NONE', #15677, .T. ) ;
#10378=CARTESIAN_POINT ( 'NONE',  ( -133.6841479863219604, -79.85751371701380208, 2.530482114511096281 ) ) ;
#10381=ADVANCED_FACE ( 'NONE', ( #2054 ), #11353, .T. ) ;
#10389=AXIS2_PLACEMENT_3D ( 'NONE', #18445, #15165, #18344 ) ;
#10396=B_SPLINE_CURVE_WITH_KNOTS ( 'NONE', 3,
 ( #12675, #7767, #20047, #4604, #14109, #15658, #3176, #1536, #7868, #4498, #7969, #10827, #6349, #18833, #11037, #4925, #20149, #14007, #11140, #9308, #9609, #15858, #7561, #1651, #10729, #15550 ),
 .UNSPECIFIED., .F., .F.,
 ( 4, 2, 2, 2, 2, 2, 2, 2, 2, 2, 2, 2, 4 ),
 ( 0.06489813153835151394, 0.07443177014004152825, 0.07681517979046398326, 0.07919858944088645214, 0.08396540874173136215, 0.09349904734342115442, 0.1030326859451109606, 0.1077995052459558289, 0.1101829148963782701, 0.1125663245468007251, 0.1220999631484905035, 0.1316336017501802680, 0.1411672403518700325 ),
 .UNSPECIFIED. ) ;
#10405=EDGE_CURVE ( 'NONE', #5526, #4062, #2270, .T. ) ;
#10406=CIRCLE ( 'NONE', #12697, 34.99999999999997868 ) ;
#10410=ORIENTED_EDGE ( 'NONE', *, *, #17035, .T. ) ;
#10412=CARTESIAN_POINT ( 'NONE',  ( -134.1070788506806082, -77.29467090009929109, 36.09959090400466408 ) ) ;
#10414=EDGE_CURVE ( 'NONE', #7514, #18061, #8580, .T. ) ;
#10417=CARTESIAN_POINT ( 'NONE',  ( -110.0000000000000142, 165.0000000000000000, 5.000000000000000888 ) ) ;
#10418=ORIENTED_EDGE ( 'NONE', *, *, #11538, .F. ) ;
#10421=ORIENTED_EDGE ( 'NONE', *, *, #18154, .T. ) ;
#10423=CIRCLE ( 'NONE', #15017, 7.500000000000007105 ) ;
#10426=ORIENTED_EDGE ( 'NONE', *, *, #19634, .F. ) ;
#10428=CARTESIAN_POINT ( 'NONE',  ( 56.84754764479240663, -154.7316448359447634, 39.99999999999999289 ) ) ;
#10429=CARTESIAN_POINT ( 'NONE',  ( -137.8187983416405018, -24.47065216059271719, -13.51171419847062793 ) ) ;
#10434=CARTESIAN_POINT ( 'NONE',  ( -67.50000000000000000, -2.085703952312275003E-13, -105.0000000000000142 ) ) ;
#10435=DIRECTION ( 'NONE',  ( 0.000000000000000000, 0.000000000000000000, -1.000000000000000000 ) ) ;
#10437=DIRECTION ( 'NONE',  ( 0.000000000000000000, 1.000000000000000000, 0.000000000000000000 ) ) ;
#10439=ORIENTED_EDGE ( 'NONE', *, *, #10136, .T. ) ;
#10440=ORIENTED_EDGE ( 'NONE', *, *, #20008, .F. ) ;
#10441=EDGE_LOOP ( 'NONE', ( #6682, #12412 ) ) ;
#10442=VECTOR ( 'NONE', #3266, 1000.000000000000000 ) ;
#10446=CARTESIAN_POINT ( 'NONE',  ( 133.3655458879726723, -81.62736142943096240, 1.797406865988563807 ) ) ;
#10447=CARTESIAN_POINT ( 'NONE',  ( -15.91767397667354800, 149.1530343478547138, 49.99999999999999289 ) ) ;
#10448=DIRECTION ( 'NONE',  ( 0.000000000000000000, 1.000000000000000000, 0.000000000000000000 ) ) ;
#10452=CARTESIAN_POINT ( 'NONE',  ( -134.3599121685007276, -75.61163470460564895, 5.100086963784538518 ) ) ;
#10454=CARTESIAN_POINT ( 'NONE',  ( 7.500000000000420997, -60.00000000000000000, -100.0000000000000000 ) ) ;
#10462=ORIENTED_EDGE ( 'NONE', *, *, #18275, .F. ) ;
#10476=VERTEX_POINT ( 'NONE', #12141 ) ;
#10477=CARTESIAN_POINT ( 'NONE',  ( -86.99687941525527890, 106.8407010200819371, -21.44284787283443094 ) ) ;
#10483=CARTESIAN_POINT ( 'NONE',  ( 132.0570769712678043, -87.76803911441056982, 39.72258563631385897 ) ) ;
#10488=ORIENTED_EDGE ( 'NONE', *, *, #2616, .F. ) ;
#10491=ORIENTED_EDGE ( 'NONE', *, *, #3641, .F. ) ;
#10496=CARTESIAN_POINT ( 'NONE',  ( 166.7850001792985495, -199.9999999999999716, 0.000000000000000000 ) ) ;
#10497=ORIENTED_EDGE ( 'NONE', *, *, #5534, .T. ) ;
#10501=CARTESIAN_POINT ( 'NONE',  ( -131.9327818480801966, -71.37991627326493926, 43.78367249533801697 ) ) ;
#10506=CIRCLE ( 'NONE', #16741, 7.500000000000012434 ) ;
#10509=CARTESIAN_POINT ( 'NONE',  ( -75.55085777469670916, 117.8649308618484355, 11.41353043461176142 ) ) ;
#10517=EDGE_LOOP ( 'NONE', ( #2238, #17549, #9687, #12720 ) ) ;
#10522=AXIS2_PLACEMENT_3D ( 'NONE', #10631, #16890, #15346 ) ;
#10523=CARTESIAN_POINT ( 'NONE',  ( 88.24590234222766583, -121.2961002105575972, -4.876953754043664269 ) ) ;
#10535=( BOUNDED_CURVE ( )  B_SPLINE_CURVE ( 3, ( #18245, #666, #4231, #9136 ),
 .UNSPECIFIED., .F., .F. ) 
 B_SPLINE_CURVE_WITH_KNOTS ( ( 4, 4 ),
 ( 1.920639998745670818, 3.141592653589790896 ),
 .UNSPECIFIED. ) 
 CURVE ( )  GEOMETRIC_REPRESENTATION_ITEM ( )  RATIONAL_B_SPLINE_CURVE ( ( 1.000000000000000000, 0.8795833682608498183, 0.8795833682608498183, 1.000000000000000000 ) ) 
 REPRESENTATION_ITEM ( '' )  );
#10540=ORIENTED_EDGE ( 'NONE', *, *, #3128, .F. ) ;
#10553=FACE_OUTER_BOUND ( 'NONE', #15706, .T. ) ;
#10554=DIRECTION ( 'NONE',  ( 1.000000000000000000, 1.613511099790693471E-16, 0.000000000000000000 ) ) ;
#10557=CARTESIAN_POINT ( 'NONE',  ( -134.6900874600844134, -73.16343714252982977, 8.507184036954340556 ) ) ;
#10558=CARTESIAN_POINT ( 'NONE',  ( 131.9259051260548290, -88.29481989229334715, 0.2208891356029132336 ) ) ;
#10561=DIRECTION ( 'NONE',  ( 0.000000000000000000, 0.000000000000000000, 1.000000000000000000 ) ) ;
#10565=AXIS2_PLACEMENT_3D ( 'NONE', #18834, #7970, #3177 ) ;
#10567=ORIENTED_EDGE ( 'NONE', *, *, #17649, .T. ) ;
#10578=CARTESIAN_POINT ( 'NONE',  ( 156.4179374840099683, -52.02840013023883614, 39.99999999999999289 ) ) ;
#10581=EDGE_CURVE ( 'NONE', #2735, #1702, #20030, .T. ) ;
#10583=CARTESIAN_POINT ( 'NONE',  ( 127.7402033587085555, -78.63140257241676068, 48.47023495424932804 ) ) ;
#10587=EDGE_CURVE ( 'NONE', #14697, #12460, #17289, .T. ) ;
#10588=EDGE_LOOP ( 'NONE', ( #14225, #12642 ) ) ;
#10592=DIRECTION ( 'NONE',  ( 0.000000000000000000, 0.000000000000000000, 1.000000000000000000 ) ) ;
#10593=ORIENTED_EDGE ( 'NONE', *, *, #11769, .F. ) ;
#10594=ORIENTED_EDGE ( 'NONE', *, *, #4883, .T. ) ;
#10614=ADVANCED_FACE ( 'NONE', ( #12659 ), #18921, .T. ) ;
#10619=CARTESIAN_POINT ( 'NONE',  ( -97.49999999999997158, -115.4778303846450029, 29.99999999999999289 ) ) ;
#10621=AXIS2_PLACEMENT_3D ( 'NONE', #1774, #231, #18973 ) ;
#10626=CARTESIAN_POINT ( 'NONE',  ( 87.34436178610390300, -121.9468435064317617, -3.953023745371848197 ) ) ;
#10628=LINE ( 'NONE', #11957, #15033 ) ;
#10631=CARTESIAN_POINT ( 'NONE',  ( 128.2779226595531270, 102.2982297021113141, 39.99999999999999289 ) ) ;
#10633=FACE_BOUND ( 'NONE', #8946, .T. ) ;
#10637=CARTESIAN_POINT ( 'NONE',  ( 97.11506731898820988, -115.6376992562306469, 29.64291924541058521 ) ) ;
#10645=AXIS2_PLACEMENT_3D ( 'NONE', #19906, #8953, #1395 ) ;
#10648=EDGE_CURVE ( 'NONE', #7495, #13974, #10406, .T. ) ;
#10654=AXIS2_PLACEMENT_3D ( 'NONE', #7289, #17678, #4013 ) ;
#10659=ORIENTED_EDGE ( 'NONE', *, *, #3614, .F. ) ;
#10661=CARTESIAN_POINT ( 'NONE',  ( -133.6648977371338844, -68.07564730482667414, 0.2001739272734736064 ) ) ;
#10663=CARTESIAN_POINT ( 'NONE',  ( 133.2381282822229025, -68.90431829399533115, -0.9334320511221024796 ) ) ;
#10666=CARTESIAN_POINT ( 'NONE',  ( -132.1020537416607397, -71.17237643004155245, 36.09957904933038719 ) ) ;
#10667=EDGE_LOOP ( 'NONE', ( #1223, #7590 ) ) ;
#10670=ORIENTED_EDGE ( 'NONE', *, *, #11613, .T. ) ;
#10675=CARTESIAN_POINT ( 'NONE',  ( -141.5781605588074683, -18.79909027762237272, 20.09932341090167895 ) ) ;
#10677=DIRECTION ( 'NONE',  ( -0.000000000000000000, 1.000000000000000000, -0.000000000000000000 ) ) ;
#10679=CARTESIAN_POINT ( 'NONE',  ( -139.3225548399015850, -10.84875705434604498, -14.11339856648029212 ) ) ;
#10682=CARTESIAN_POINT ( 'NONE',  ( -85.01747478753389942, 109.2823643868091779, -19.52988736366387101 ) ) ;
#10684=FACE_OUTER_BOUND ( 'NONE', #14708, .T. ) ;
#10688=AXIS2_PLACEMENT_3D ( 'NONE', #7347, #19825, #15325 ) ;
#10690=CARTESIAN_POINT ( 'NONE',  ( 129.1041139275565968, -76.37100075998219495, 47.39509621162856945 ) ) ;
#10691=FACE_OUTER_BOUND ( 'NONE', #10247, .T. ) ;
#10693=EDGE_CURVE ( 'NONE', #6419, #11868, #6237, .T. ) ;
#10696=ORIENTED_EDGE ( 'NONE', *, *, #3411, .F. ) ;
#10700=CARTESIAN_POINT ( 'NONE',  ( -159.9599531637108782, -36.50981547337168109, 49.99999999999999289 ) ) ;
#10705=FACE_OUTER_BOUND ( 'NONE', #4560, .T. ) ;
#10711=DIRECTION ( 'NONE',  ( 0.000000000000000000, 0.000000000000000000, -1.000000000000000000 ) ) ;
#10715=DIRECTION ( 'NONE',  ( 0.000000000000000000, 1.000000000000000000, 0.000000000000000000 ) ) ;
#10720=ORIENTED_EDGE ( 'NONE', *, *, #9514, .F. ) ;
#10723=CARTESIAN_POINT ( 'NONE',  ( 0.000000000000000000, 0.000000000000000000, -115.0000000000000142 ) ) ;
#10725=ORIENTED_EDGE ( 'NONE', *, *, #19006, .F. ) ;
#10729=CARTESIAN_POINT ( 'NONE',  ( -146.5157903719973262, 32.27091178421088102, -11.39721689603033283 ) ) ;
#10732=ORIENTED_EDGE ( 'NONE', *, *, #16609, .F. ) ;
#10733=CARTESIAN_POINT ( 'NONE',  ( 84.44661573609288041, -123.9709896190459233, 0.1742278272254467741 ) ) ;
#10742=DIRECTION ( 'NONE',  ( 0.000000000000000000, 0.000000000000000000, -1.000000000000000000 ) ) ;
#10744=CARTESIAN_POINT ( 'NONE',  ( 97.93656923779383305, -133.3799209237882053, 32.92832214187814799 ) ) ;
#10745=ORIENTED_EDGE ( 'NONE', *, *, #8520, .F. ) ;
#10746=CIRCLE ( 'NONE', #7171, 150.0000000000000284 ) ;
#10751=VECTOR ( 'NONE', #10230, 1000.000000000000114 ) ;
#10758=EDGE_LOOP ( 'NONE', ( #9909, #8789 ) ) ;
#10761=DIRECTION ( 'NONE',  ( -0.000000000000000000, -1.000000000000000000, -0.000000000000000000 ) ) ;
#10764=CARTESIAN_POINT ( 'NONE',  ( -99.98863955314961061, -130.5690324404936291, 36.60999800948973615 ) ) ;
#10766=VECTOR ( 'NONE', #5020, 1000.000000000000000 ) ;
#10769=CARTESIAN_POINT ( 'NONE',  ( -134.5315346870343376, -74.37329574990532421, 6.387021999321605747 ) ) ;
#10770=CARTESIAN_POINT ( 'NONE',  ( 132.7564094051595589, -84.67399327755590832, 0.8739656915399692805 ) ) ;
#10773=CARTESIAN_POINT ( 'NONE',  ( -125.5405970674900971, -82.09774788367874976, 49.55822172878893639 ) ) ;
#10777=CYLINDRICAL_SURFACE ( 'NONE', #15758, 32.50000000000000000 ) ;
#10778=VERTEX_POINT ( 'NONE', #9793 ) ;
#10787=CARTESIAN_POINT ( 'NONE',  ( 0.000000000000000000, 0.000000000000000000, 40.00000000000000000 ) ) ;
#10790=ORIENTED_EDGE ( 'NONE', *, *, #17948, .F. ) ;
#10791=CARTESIAN_POINT ( 'NONE',  ( -82.42673853863954037, 112.2670201977909556, -16.56329132253156189 ) ) ;
#10792=CARTESIAN_POINT ( 'NONE',  ( -97.49999999999997158, -190.0000000000000000, 30.00000000000000000 ) ) ;
#10798=ORIENTED_EDGE ( 'NONE', *, *, #15405, .F. ) ;
#10802=CIRCLE ( 'NONE', #1334, 110.0000000000000142 ) ;
#10803=ORIENTED_EDGE ( 'NONE', *, *, #14231, .F. ) ;
#10804=EDGE_LOOP ( 'NONE', ( #7306, #17209, #4085, #9989 ) ) ;
#10808=CYLINDRICAL_SURFACE ( 'NONE', #6141, 9.999999999999994671 ) ;
#10811=CARTESIAN_POINT ( 'NONE',  ( 0.000000000000000000, 0.000000000000000000, -10.00000000000000178 ) ) ;
#10812=ORIENTED_EDGE ( 'NONE', *, *, #6161, .F. ) ;
#10815=DIRECTION ( 'NONE',  ( 0.000000000000000000, 1.000000000000000000, 0.000000000000000000 ) ) ;
#10818=DIRECTION ( 'NONE',  ( -0.000000000000000000, -1.000000000000000000, -0.000000000000000000 ) ) ;
#10820=CARTESIAN_POINT ( 'NONE',  ( -98.89944939536758284, 99.14269198534090322, 38.28897304660228684 ) ) ;
#10821=ORIENTED_EDGE ( 'NONE', *, *, #17432, .T. ) ;
#10824=VERTEX_POINT ( 'NONE', #9896 ) ;
#10825=CARTESIAN_POINT ( 'NONE',  ( -82.80829968035172328, -125.0716697069619840, 35.88848305379081438 ) ) ;
#10826=ORIENTED_EDGE ( 'NONE', *, *, #438, .T. ) ;
#10827=CARTESIAN_POINT ( 'NONE',  ( -129.5808341847080669, 64.44470624890260524, -29.94181153629256542 ) ) ;
#10830=CARTESIAN_POINT ( 'NONE',  ( 96.67521566530152199, -115.8170149452160018, 10.31811481433898692 ) ) ;
#10833=CIRCLE ( 'NONE', #10184, 7.500000000000003553 ) ;
#10836=FACE_BOUND ( 'NONE', #4488, .T. ) ;
#10839=CARTESIAN_POINT ( 'NONE',  ( 4.189777606611760026E-13, -60.00000000000000000, -100.0000000000000000 ) ) ;
#10842=CARTESIAN_POINT ( 'NONE',  ( 99.15855529360270282, -131.7281685730150400, 35.51823119121745265 ) ) ;
#10845=DIRECTION ( 'NONE',  ( 0.000000000000000000, 0.000000000000000000, 1.000000000000000000 ) ) ;
#10849=ORIENTED_EDGE ( 'NONE', *, *, #2547, .F. ) ;
#10855=PLANE ( 'NONE',  #12725 ) ;
#10858=AXIS2_PLACEMENT_3D ( 'NONE', #13606, #10435, #19852 ) ;
#10863=CARTESIAN_POINT ( 'NONE',  ( -100.6915138157995386, -129.5610470606159481, 37.32613602704453371 ) ) ;
#10864=LINE ( 'NONE', #17228, #16545 ) ;
#10868=CARTESIAN_POINT ( 'NONE',  ( 128.1750136849898354, -77.98139142652387079, -0.5590989923425794261 ) ) ;
#10871=DIRECTION ( 'NONE',  ( 0.9009688679024154823, 0.4338837391175657809, 0.000000000000000000 ) ) ;
#10872=DIRECTION ( 'NONE',  ( -0.000000000000000000, 1.000000000000000000, -0.000000000000000000 ) ) ;
#10873=CARTESIAN_POINT ( 'NONE',  ( -133.2381282822229025, -68.90431829399531694, 40.93343205112707750 ) ) ;
#10874=VERTEX_POINT ( 'NONE', #6638 ) ;
#10880=ORIENTED_EDGE ( 'NONE', *, *, #14749, .F. ) ;
#10883=EDGE_CURVE ( 'NONE', #1562, #6720, #4728, .T. ) ;
#10884=CARTESIAN_POINT ( 'NONE',  ( -130.9868171408399462, -91.88282611735539263, 0.000000000000000000 ) ) ;
#10886=ORIENTED_EDGE ( 'NONE', *, *, #19259, .F. ) ;
#10887=CIRCLE ( 'NONE', #771, 15.91767397667354444 ) ;
#10893=AXIS2_PLACEMENT_3D ( 'NONE', #15631, #9588, #6430 ) ;
#10897=CARTESIAN_POINT ( 'NONE',  ( 131.7825524766324463, -71.64958008132042266, 43.99896812349997077 ) ) ;
#10898=CARTESIAN_POINT ( 'NONE',  ( -107.4999999999999716, -200.0000000000000000, 0.000000000000000000 ) ) ;
#10899=EDGE_CURVE ( 'NONE', #16122, #3485, #19902, .T. ) ;
#10902=ORIENTED_EDGE ( 'NONE', *, *, #10899, .F. ) ;
#10908=VERTEX_POINT ( 'NONE', #1071 ) ;
#10926=CARTESIAN_POINT ( 'NONE',  ( -75.12965072324909954, 118.1335604146951113, 8.039948435259535842 ) ) ;
#10929=ORIENTED_EDGE ( 'NONE', *, *, #11626, .T. ) ;
#10935=DIRECTION ( 'NONE',  ( 0.000000000000000000, 0.000000000000000000, 1.000000000000000000 ) ) ;
#10938=CARTESIAN_POINT ( 'NONE',  ( 97.21757233051022240, -115.5955488200751518, 10.33714169725774212 ) ) ;
#10943=ORIENTED_EDGE ( 'NONE', *, *, #14231, .T. ) ;
#10948=CARTESIAN_POINT ( 'NONE',  ( 83.54968581051038257, -124.5775662629409766, 37.91678146420370155 ) ) ;
#10958=CARTESIAN_POINT ( 'NONE',  ( -101.1753893487742033, -128.8598102521084456, 2.230270385704167246 ) ) ;
#10959=B_SPLINE_CURVE_WITH_KNOTS ( 'NONE', 3,
 ( #9827, #6470, #8292, #2068, #115, #19149, #7886, #12797, #18956, #5041, #14233, #9629, #1661, #4942, #14127, #6368, #213, #17319, #12585, #12692, #1964, #12995, #12895, #18848, #8193, #19253, #11157, #17422, #4835, #17621, #317, #15674, #527, #1857, #11055, #9533, #15771, #1754, #6771, #5239, #7987, #3396, #15977, #3693, #3596, #11464 ),
 .UNSPECIFIED., .F., .F.,
 ( 4, 2, 2, 2, 2, 2, 2, 2, 2, 2, 2, 2, 2, 2, 2, 2, 2, 2, 2, 2, 2, 2, 4 ),
 ( 1.214306433183764966E-17, 0.005452065557044396583, 0.01090413111408878102, 0.01363016389261097021, 0.01635619667113315939, 0.02180826222817754123, 0.02317127861743863843, 0.02453429500669972868, 0.02726032778522194389, 0.03271239334226637430, 0.03543842612078860338, 0.03816445889931082552, 0.04361652445635528369, 0.04634255723487753359, 0.04906859001339978349, 0.05452065557044430411, 0.05997272112748881778, 0.06269875390601106768, 0.06542478668453331758, 0.07632891779862233106, 0.07905495057714460871, 0.08178098335566688637, 0.08723304891271140005 ),
 .UNSPECIFIED. ) ;
#10960=LINE ( 'NONE', #12288, #18172 ) ;
#10966=CARTESIAN_POINT ( 'NONE',  ( -99.35210738963753840, -131.4612102079657916, 35.80770037246424664 ) ) ;
#10968=VECTOR ( 'NONE', #953, 1000.000000000000000 ) ;
#10970=CARTESIAN_POINT ( 'NONE',  ( -134.6566615416656418, 38.49973993374615588, 29.87962448166155127 ) ) ;
#10971=PLANE ( 'NONE',  #14236 ) ;
#10973=CARTESIAN_POINT ( 'NONE',  ( -87.50000000000000000, -133.9542832461881687, 30.00000000000000000 ) ) ;
#10975=CARTESIAN_POINT ( 'NONE',  ( -130.5436973595314498, -73.98181611797480173, 38.74509961212098830 ) ) ;
#10980=VERTEX_POINT ( 'NONE', #7130 ) ;
#10981=AXIS2_PLACEMENT_3D ( 'NONE', #10787, #20098, #9260 ) ;
#10982=VERTEX_POINT ( 'NONE', #16543 ) ;
#10984=CARTESIAN_POINT ( 'NONE',  ( -142.9809548150034573, -16.70024071994362203, -6.750090680848771285 ) ) ;
#10987=ADVANCED_FACE ( 'NONE', ( #8753 ), #14994, .T. ) ;
#10989=CARTESIAN_POINT ( 'NONE',  ( 0.000000000000000000, 0.000000000000000000, -105.0000000000000142 ) ) ;
#10990=EDGE_CURVE ( 'NONE', #5660, #15236, #19569, .T. ) ;
#10993=DIRECTION ( 'NONE',  ( -0.000000000000000000, -0.000000000000000000, 1.000000000000000000 ) ) ;
#10998=CARTESIAN_POINT ( 'NONE',  ( 134.5985778548171652, -73.87143572891014287, 32.93474295113719563 ) ) ;
#10999=CARTESIAN_POINT ( 'NONE',  ( 134.7188131032333445, -72.93593548660992099, 30.49611318099233515 ) ) ;
#11004=ORIENTED_EDGE ( 'NONE', *, *, #13108, .T. ) ;
#11005=VERTEX_POINT ( 'NONE', #3332 ) ;
#11008=DIRECTION ( 'NONE',  ( 0.000000000000000000, 0.000000000000000000, 1.000000000000000000 ) ) ;
#11012=DIRECTION ( 'NONE',  ( -0.000000000000000000, -0.000000000000000000, -1.000000000000000000 ) ) ;
#11015=CARTESIAN_POINT ( 'NONE',  ( 131.0911649403506374, -72.90709374210200622, -5.085999411194714881 ) ) ;
#11018=ORIENTED_EDGE ( 'NONE', *, *, #5787, .F. ) ;
#11022=CARTESIAN_POINT ( 'NONE',  ( -86.93963912163985697, 117.1591715488320062, -27.74534354785872736 ) ) ;
#11025=DIRECTION ( 'NONE',  ( -0.000000000000000000, -0.000000000000000000, 1.000000000000000000 ) ) ;
#11027=PLANE ( 'NONE',  #10323 ) ;
#11029=CARTESIAN_POINT ( 'NONE',  ( 176.1792632384392334, -186.5724904703758682, 30.00000000000000000 ) ) ;
#11033=VERTEX_POINT ( 'NONE', #12428 ) ;
#11034=DIRECTION ( 'NONE',  ( -0.000000000000000000, -0.000000000000000000, -1.000000000000000000 ) ) ;
#11036=VERTEX_POINT ( 'NONE', #15508 ) ;
#11037=CARTESIAN_POINT ( 'NONE',  ( -134.7839606304467566, 57.38400188359436527, -26.41417060242037351 ) ) ;
#11041=CARTESIAN_POINT ( 'NONE',  ( 97.50000000000000000, -133.9542832461881687, 9.999999999999996447 ) ) ;
#11043=VECTOR ( 'NONE', #12421, 1000.000000000000000 ) ;
#11045=DIRECTION ( 'NONE',  ( -0.000000000000000000, -0.000000000000000000, -1.000000000000000000 ) ) ;
#11046=AXIS2_PLACEMENT_3D ( 'NONE', #9719, #17206, #14123 ) ;
#11050=DIRECTION ( 'NONE',  ( 0.2225209339563183342, -0.9749279121818226201, 0.000000000000000000 ) ) ;
#11052=FACE_OUTER_BOUND ( 'NONE', #14575, .T. ) ;
#11053=VERTEX_POINT ( 'NONE', #18788 ) ;
#11055=CARTESIAN_POINT ( 'NONE',  ( -91.62566160141871308, 118.7664292046248278, 40.53793933303452945 ) ) ;
#11056=EDGE_LOOP ( 'NONE', ( #13506, #16129 ) ) ;
#11061=VECTOR ( 'NONE', #13624, 1000.000000000000227 ) ;
#11064=CARTESIAN_POINT ( 'NONE',  ( -98.02151343901456926, -133.2674925500989218, 6.780480114272203984 ) ) ;
#11067=DIRECTION ( 'NONE',  ( 0.000000000000000000, 0.000000000000000000, 1.000000000000000000 ) ) ;
#11069=CARTESIAN_POINT ( 'NONE',  ( -97.49999999944088813, -115.4778303847294154, 10.15726746729510310 ) ) ;
#11070=CARTESIAN_POINT ( 'NONE',  ( -95.49511753037597828, -115.9200926448052940, 33.43441907682297654 ) ) ;
#11071=LINE ( 'NONE', #17119, #16857 ) ;
#11073=FACE_BOUND ( 'NONE', #17398, .T. ) ;
#11074=DIRECTION ( 'NONE',  ( 0.000000000000000000, 1.000000000000000000, 0.000000000000000000 ) ) ;
#11078=CARTESIAN_POINT ( 'NONE',  ( -126.7459963399414988, -80.26907437897514797, 41.00725567157765283 ) ) ;
#11079=CIRCLE ( 'NONE', #12372, 99.99999999999997158 ) ;
#11080=ORIENTED_EDGE ( 'NONE', *, *, #3017, .T. ) ;
#11086=CARTESIAN_POINT ( 'NONE',  ( -145.0141832565074935, -14.10286991559387459, 4.805853499333125889 ) ) ;
#11087=VECTOR ( 'NONE', #2000, 1000.000000000000000 ) ;
#11095=CARTESIAN_POINT ( 'NONE',  ( 128.2779226595531270, 102.2982297021113141, 49.99999999999999289 ) ) ;
#11096=CARTESIAN_POINT ( 'NONE',  ( 97.63534213009857865, -133.7771032679719667, 31.65634370844862389 ) ) ;
#11099=CARTESIAN_POINT ( 'NONE',  ( 134.7130977013151778, -72.98159303036058532, 30.74846602018423170 ) ) ;
#11100=TOROIDAL_SURFACE ( 'NONE', #9493, 160.0000000000000284, 10.00000000000000000 ) ;
#11102=ORIENTED_EDGE ( 'NONE', *, *, #10990, .T. ) ;
#11104=EDGE_CURVE ( 'NONE', #8290, #12020, #949, .T. ) ;
#11106=EDGE_CURVE ( 'NONE', #5457, #16596, #1294, .T. ) ;
#11108=ADVANCED_FACE ( 'NONE', ( #10684 ), #16942, .T. ) ;
#11112=CARTESIAN_POINT ( 'NONE',  ( -101.4288913641181438, -128.4806265586112204, 37.95194130168881230 ) ) ;
#11121=ADVANCED_FACE ( 'NONE', ( #18472 ), #1388, .F. ) ;
#11123=DIRECTION ( 'NONE',  ( 1.000000000000000000, 0.000000000000000000, 0.000000000000000000 ) ) ;
#11128=CYLINDRICAL_SURFACE ( 'NONE', #16025, 7.500000000000007105 ) ;
#11130=EDGE_LOOP ( 'NONE', ( #5024, #11018, #10274, #10421 ) ) ;
#11137=ADVANCED_FACE ( 'NONE', ( #356, #9866 ), #567, .T. ) ;
#11138=FACE_OUTER_BOUND ( 'NONE', #4950, .T. ) ;
#11140=CARTESIAN_POINT ( 'NONE',  ( -137.5420331966829224, 53.19132841792027477, -24.01216543166409068 ) ) ;
#11154=CARTESIAN_POINT ( 'NONE',  ( 97.52847697650780390, -113.9950050384823896, 37.53234943820369551 ) ) ;
#11157=CARTESIAN_POINT ( 'NONE',  ( -80.29253715427383042, 126.7026982456581123, 31.79868549975239134 ) ) ;
#11160=VERTEX_POINT ( 'NONE', #11197 ) ;
#11165=CARTESIAN_POINT ( 'NONE',  ( -97.53517841124883603, -133.9083944458743076, 9.039724941871954300 ) ) ;
#11173=CARTESIAN_POINT ( 'NONE',  ( -95.47048624632753899, -116.1260213179369600, 31.97844772384138068 ) ) ;
#11176=FACE_OUTER_BOUND ( 'NONE', #12816, .T. ) ;
#11178=CARTESIAN_POINT ( 'NONE',  ( -136.4994460260997187, -31.11111111111111782, -115.0000000000000142 ) ) ;
#11180=VERTEX_POINT ( 'NONE', #2105 ) ;
#11186=ORIENTED_EDGE ( 'NONE', *, *, #5772, .T. ) ;
#11189=CARTESIAN_POINT ( 'NONE',  ( -143.0918807612787020, -16.54827070355140961, 16.43686625575313087 ) ) ;
#11193=AXIS2_PLACEMENT_3D ( 'NONE', #17832, #15048, #2878 ) ;
#11197=CARTESIAN_POINT ( 'NONE',  ( -147.0809924354783220, 29.44794838685322702, -9.999999999999978684 ) ) ;
#11200=CARTESIAN_POINT ( 'NONE',  ( 4.189777606611760026E-13, -60.00000000000000000, -100.0000000000000000 ) ) ;
#11202=CARTESIAN_POINT ( 'NONE',  ( 134.7264294273387009, -65.94569739564036581, 35.17155507723151686 ) ) ;
#11206=AXIS2_PLACEMENT_3D ( 'NONE', #7020, #14591, #14787 ) ;
#11216=CARTESIAN_POINT ( 'NONE',  ( 50.37374754117451658, -141.2886604036503115, 39.99999999999999289 ) ) ;
#11218=CARTESIAN_POINT ( 'NONE',  ( 130.1901167961280237, -74.50443780700841501, -6.262183608668058454 ) ) ;
#11224=CIRCLE ( 'NONE', #5042, 42.50000000000000000 ) ;
#11231=CARTESIAN_POINT ( 'NONE',  ( 84.30790708731538530, -124.0658650269852501, 39.57734081243646074 ) ) ;
#11232=VERTEX_POINT ( 'NONE', #17563 ) ;
#11234=AXIS2_PLACEMENT_3D ( 'NONE', #19917, #12238, #15525 ) ;
#11238=FACE_OUTER_BOUND ( 'NONE', #16158, .T. ) ;
#11239=ORIENTED_EDGE ( 'NONE', *, *, #8592, .F. ) ;
#11241=CARTESIAN_POINT ( 'NONE',  ( -29.99999999999887379, 275.0000000000000000, 12.49999999999916511 ) ) ;
#11242=ORIENTED_EDGE ( 'NONE', *, *, #7383, .T. ) ;
#11244=CARTESIAN_POINT ( 'NONE',  ( 32.50000000000000000, 3.980102097228897837E-15, -40.00000000000000000 ) ) ;
#11246=EDGE_CURVE ( 'NONE', #19595, #10224, #3895, .T. ) ;
#11256=CARTESIAN_POINT ( 'NONE',  ( -109.9999999999874376, 73.61623156955475622, -29.99999999999998579 ) ) ;
#11257=CARTESIAN_POINT ( 'NONE',  ( 56.84754764479240663, -154.7316448359447634, 39.99999999999999289 ) ) ;
#11258=VERTEX_POINT ( 'NONE', #9438 ) ;
#11263=ORIENTED_EDGE ( 'NONE', *, *, #7031, .T. ) ;
#11265=EDGE_CURVE ( 'NONE', #7708, #1300, #9539, .T. ) ;
#11270=CARTESIAN_POINT ( 'NONE',  ( -118.0985281540987017, 92.51441522866370804, 44.20207086512186123 ) ) ;
#11271=ORIENTED_EDGE ( 'NONE', *, *, #17374, .T. ) ;
#11272=AXIS2_PLACEMENT_3D ( 'NONE', #14426, #8377, #406 ) ;
#11273=DIRECTION ( 'NONE',  ( 1.000000000000000000, 0.000000000000000000, 0.000000000000000000 ) ) ;
#11278=EDGE_CURVE ( 'NONE', #1151, #2847, #15469, .T. ) ;
#11279=EDGE_CURVE ( 'NONE', #1151, #7965, #6653, .T. ) ;
#11280=CARTESIAN_POINT ( 'NONE',  ( -129.6868978415389222, 52.87694723226520210, 33.99445347032297349 ) ) ;
#11281=ADVANCED_FACE ( 'NONE', ( #6175 ), #10855, .T. ) ;
#11283=CARTESIAN_POINT ( 'NONE',  ( -149.5153435750498829, 12.29774247357356565, -1.337809393647938938 ) ) ;
#11289=CARTESIAN_POINT ( 'NONE',  ( -139.8142396999972163, 1.712230611238718486E-14, -13.33333333333329307 ) ) ;
#11294=ORIENTED_EDGE ( 'NONE', *, *, #3128, .T. ) ;
#11295=CARTESIAN_POINT ( 'NONE',  ( 82.03125000000004263, -125.5821405433013780, 10.00000000000000178 ) ) ;
#11298=DIRECTION ( 'NONE',  ( -0.000000000000000000, -0.000000000000000000, -1.000000000000000000 ) ) ;
#11301=CARTESIAN_POINT ( 'NONE',  ( 71.18887634719571622, -147.8252249328912740, 49.99999999999999289 ) ) ;
#11302=CARTESIAN_POINT ( 'NONE',  ( -136.4621351594848875, -31.11743562882559644, -11.66901485073876010 ) ) ;
#11307=DIRECTION ( 'NONE',  ( 1.000000000000000000, 0.000000000000000000, 0.000000000000000000 ) ) ;
#11311=CARTESIAN_POINT ( 'NONE',  ( 132.8189972983174414, -84.37332251142814243, 39.04785267872424726 ) ) ;
#11316=ORIENTED_EDGE ( 'NONE', *, *, #14021, .F. ) ;
#11322=CARTESIAN_POINT ( 'NONE',  ( -103.6579813550139875, -125.0534741538843804, 39.24896055728943622 ) ) ;
#11325=ORIENTED_EDGE ( 'NONE', *, *, #11246, .T. ) ;
#11326=CARTESIAN_POINT ( 'NONE',  ( 135.0159133995099410, -65.35183200177810647, 7.107308349490855548 ) ) ;
#11331=DIRECTION ( 'NONE',  ( 0.000000000000000000, 0.000000000000000000, 1.000000000000000000 ) ) ;
#11334=EDGE_CURVE ( 'NONE', #18649, #14660, #13696, .T. ) ;
#11336=CIRCLE ( 'NONE', #9696, 7.500000000000007105 ) ;
#11339=CARTESIAN_POINT ( 'NONE',  ( -77.67451021423168811, 116.4791384160827192, -8.518550530975769419 ) ) ;
#11344=DIRECTION ( 'NONE',  ( 1.000000000000000000, 1.613511099790691498E-16, -0.000000000000000000 ) ) ;
#11352=CARTESIAN_POINT ( 'NONE',  ( 166.7850001792985495, -189.9999999999999432, 40.00000000000000000 ) ) ;
#11353=CYLINDRICAL_SURFACE ( 'NONE', #19880, 15.91767397667354089 ) ;
#11358=CYLINDRICAL_SURFACE ( 'NONE', #19064, 7.500000000000002665 ) ;
#11361=CARTESIAN_POINT ( 'NONE',  ( -140.0000000000000000, 1.714505518806294914E-14, 49.99999999999999289 ) ) ;
#11362=AXIS2_PLACEMENT_3D ( 'NONE', #1193, #7437, #12549 ) ;
#11373=VERTEX_POINT ( 'NONE', #13187 ) ;
#11376=CARTESIAN_POINT ( 'NONE',  ( -148.3536700004592319, 22.27615101400069264, 16.41737317648027883 ) ) ;
#11379=DIRECTION ( 'NONE',  ( 0.3427509529624101492, -0.9394263059140720573, 0.000000000000000000 ) ) ;
#11380=CARTESIAN_POINT ( 'NONE',  ( -103.0386482854710977, -126.0278359105729891, 1.045141973220539811 ) ) ;
#11382=EDGE_CURVE ( 'NONE', #10980, #11724, #2920, .T. ) ;
#11383=CARTESIAN_POINT ( 'NONE',  ( -136.5225140300081534, 31.06975746072189892, 27.84628854908055118 ) ) ;
#11385=CARTESIAN_POINT ( 'NONE',  ( -148.0615764913603698, 24.55031428987399522, -7.575931336099094970 ) ) ;
#11386=DIRECTION ( 'NONE',  ( 0.4338837391175654479, -0.9009688679024155933, 0.000000000000000000 ) ) ;
#11388=ORIENTED_EDGE ( 'NONE', *, *, #18242, .T. ) ;
#11389=CARTESIAN_POINT ( 'NONE',  ( -122.3581121773129183, 55.09912925957832641, -27.76044880785753577 ) ) ;
#11390=AXIS2_PLACEMENT_3D ( 'NONE', #16985, #17299, #10935 ) ;
#11393=AXIS2_PLACEMENT_3D ( 'NONE', #3849, #2328, #8556 ) ;
#11395=EDGE_CURVE ( 'NONE', #16596, #2991, #14742, .T. ) ;
#11396=EDGE_LOOP ( 'NONE', ( #13327, #17160, #471, #16873 ) ) ;
#11400=DIRECTION ( 'NONE',  ( 0.000000000000000000, 1.000000000000000000, 0.000000000000000000 ) ) ;
#11422=ORIENTED_EDGE ( 'NONE', *, *, #19231, .T. ) ;
#11424=DIRECTION ( 'NONE',  ( 0.000000000000000000, 0.000000000000000000, 1.000000000000000000 ) ) ;
#11430=CARTESIAN_POINT ( 'NONE',  ( 134.3888575020695555, -66.63121209263867684, 2.991575443300840575 ) ) ;
#11432=EDGE_LOOP ( 'NONE', ( #1593, #19546, #9942, #20012 ) ) ;
#11433=DIRECTION ( 'NONE',  ( 0.000000000000000000, 1.000000000000000000, 0.000000000000000000 ) ) ;
#11439=CARTESIAN_POINT ( 'NONE',  ( 82.89467276472738888, -125.0139572091429869, 36.00987770447442671 ) ) ;
#11445=EDGE_LOOP ( 'NONE', ( #14976, #6595, #9638, #16564 ) ) ;
#11449=CARTESIAN_POINT ( 'NONE',  ( 0.000000000000000000, 0.000000000000000000, 49.99999999999999289 ) ) ;
#11450=CARTESIAN_POINT ( 'NONE',  ( 0.000000000000000000, 0.000000000000000000, 39.99999999999999289 ) ) ;
#11453=LINE ( 'NONE', #16271, #4796 ) ;
#11454=CARTESIAN_POINT ( 'NONE',  ( 100.4560359297608585, -129.9019447003570349, 2.893739865237928033 ) ) ;
#11457=DIRECTION ( 'NONE',  ( -0.000000000000000000, -0.000000000000000000, 1.000000000000000000 ) ) ;
#11458=DIRECTION ( 'NONE',  ( 1.000000000000000000, 0.000000000000000000, 0.000000000000000000 ) ) ;
#11459=CARTESIAN_POINT ( 'NONE',  ( 91.69207598197974107, -118.7138234487252078, -7.504338834299504768 ) ) ;
#11460=CIRCLE ( 'NONE', #1324, 7.500000000000001776 ) ;
#11463=DIRECTION ( 'NONE',  ( 1.000000000000000000, 3.129754055707530415E-16, -0.000000000000000000 ) ) ;
#11464=CARTESIAN_POINT ( 'NONE',  ( -110.0000000000000284, 101.9803902718557111, 44.99999999999998579 ) ) ;
#11471=DIRECTION ( 'NONE',  ( -1.000000000000000000, 0.000000000000000000, 0.000000000000000000 ) ) ;
#11475=CARTESIAN_POINT ( 'NONE',  ( -96.93610878393819519, -115.7104363121878094, 10.35199856087829673 ) ) ;
#11481=ADVANCED_FACE ( 'NONE', ( #2768 ), #19737, .T. ) ;
#11485=VERTEX_POINT ( 'NONE', #7176 ) ;
#11490=EDGE_CURVE ( 'NONE', #14482, #8290, #19907, .T. ) ;
#11491=ORIENTED_EDGE ( 'NONE', *, *, #12661, .F. ) ;
#11492=DIRECTION ( 'NONE',  ( 0.2225209339563044841, 0.9749279121818258398, 0.000000000000000000 ) ) ;
#11493=B_SPLINE_CURVE_WITH_KNOTS ( 'NONE', 3,
 ( #11900, #12003, #9149, #18261, #12102, #5992, #2512, #15390, #18362, #4340, #12211, #10675, #16930, #18781, #251, #8021, #11189, #4762, #4553, #9356, #17454, #152, #8122, #3326, #4658, #17140, #11086, #51, #12621, #14268, #15707, #12309, #1583, #18882, #13952, #14063, #10984, #9564, #6503, #15496, #1483, #18987 ),
 .UNSPECIFIED., .F., .F.,
 ( 4, 2, 2, 2, 2, 2, 2, 2, 2, 2, 2, 2, 2, 2, 2, 2, 2, 2, 2, 2, 4 ),
 ( -0.03221374292090079666, -0.02616091102393758305, -0.02464770304969675710, -0.02313449507545593115, -0.02010807912697429312, -0.01708166317849265509, -0.01556845520425183260, -0.01405524723001101359, -0.01102883128152938250, -0.009515623307288563482, -0.008002415333047747936, -0.004975999384566141132, -0.001949583436084537796, 0.001076832512397069008, 0.004103248460878679282, 0.007129664409360289556, 0.008642872383601091224, 0.01015608035784189289, 0.01318249630632349623, 0.01469570428056430483, 0.01620891225480510650 ),
 .UNSPECIFIED. ) ;
#11494=CARTESIAN_POINT ( 'NONE',  ( -131.6317334595287605, -71.92650142027846982, -4.251463035882792063 ) ) ;
#11499=CARTESIAN_POINT ( 'NONE',  ( -123.3142212418527350, -85.40728428758222890, -0.3493686248430047381 ) ) ;
#11500=EDGE_CURVE ( 'NONE', #6137, #2972, #18317, .T. ) ;
#11505=CARTESIAN_POINT ( 'NONE',  ( 102.1629267457074519, -127.3823967956316210, 38.47850501251131305 ) ) ;
#11513=CARTESIAN_POINT ( 'NONE',  ( -166.7850001792984926, -200.0000000000000284, 40.00000000000000000 ) ) ;
#11517=ORIENTED_EDGE ( 'NONE', *, *, #762, .T. ) ;
#11519=DIRECTION ( 'NONE',  ( 0.000000000000000000, 0.000000000000000000, 1.000000000000000000 ) ) ;
#11523=CARTESIAN_POINT ( 'NONE',  ( 0.000000000000000000, 0.000000000000000000, -115.0000000000000142 ) ) ;
#11524=CARTESIAN_POINT ( 'NONE',  ( -97.49999999999998579, -113.9901311517800337, 10.00000000000000178 ) ) ;
#11525=EDGE_LOOP ( 'NONE', ( #3340, #10696 ) ) ;
#11532=CARTESIAN_POINT ( 'NONE',  ( -137.8571306610627971, -24.85219049267718106, -16.19534811600425428 ) ) ;
#11537=DIRECTION ( 'NONE',  ( -1.000000000000000000, 0.000000000000000000, 0.000000000000000000 ) ) ;
#11538=EDGE_CURVE ( 'NONE', #7342, #10874, #2565, .T. ) ;
#11543=CIRCLE ( 'NONE', #14811, 110.0000000000000142 ) ;
#11546=CARTESIAN_POINT ( 'NONE',  ( -93.79892245610578527, -117.0565612855932329, 48.57152639572796460 ) ) ;
#11548=DIRECTION ( 'NONE',  ( -0.000000000000000000, -0.000000000000000000, 1.000000000000000000 ) ) ;
#11556=ORIENTED_EDGE ( 'NONE', *, *, #12097, .T. ) ;
#11559=CARTESIAN_POINT ( 'NONE',  ( 93.26156191356916736, -117.4850166029420535, -8.331654811393381266 ) ) ;
#11560=LINE ( 'NONE', #11257, #5327 ) ;
#11570=DIRECTION ( 'NONE',  ( 0.000000000000000000, 0.000000000000000000, -1.000000000000000000 ) ) ;
#11576=CARTESIAN_POINT ( 'NONE',  ( -96.67218534448896605, -115.8154871359607796, 10.27722555384923098 ) ) ;
#11580=FACE_BOUND ( 'NONE', #9728, .T. ) ;
#11583=CARTESIAN_POINT ( 'NONE',  ( 0.000000000000000000, 0.000000000000000000, -10.00000000000000178 ) ) ;
#11591=ORIENTED_EDGE ( 'NONE', *, *, #18680, .F. ) ;
#11593=DIRECTION ( 'NONE',  ( 0.000000000000000000, 0.000000000000000000, 1.000000000000000000 ) ) ;
#11597=CARTESIAN_POINT ( 'NONE',  ( -87.49999999999998579, -133.9542832461881687, 49.99999999999999289 ) ) ;
#11598=CARTESIAN_POINT ( 'NONE',  ( -129.7881937802468428, -75.28665481071030285, 0.5105156109461032043 ) ) ;
#11600=CARTESIAN_POINT ( 'NONE',  ( 0.000000000000000000, 0.000000000000000000, 49.99999999999999289 ) ) ;
#11603=EDGE_CURVE ( 'NONE', #13285, #5634, #11736, .T. ) ;
#11607=CIRCLE ( 'NONE', #10621, 160.0000000000000284 ) ;
#11608=ORIENTED_EDGE ( 'NONE', *, *, #6909, .T. ) ;
#11613=EDGE_CURVE ( 'NONE', #65, #11160, #10396, .T. ) ;
#11616=PLANE ( 'NONE',  #9417 ) ;
#11626=EDGE_CURVE ( 'NONE', #16701, #19189, #9751, .T. ) ;
#11631=CARTESIAN_POINT ( 'NONE',  ( 138.2024300533213932, 89.85329105948596862, 39.99999999999999289 ) ) ;
#11639=LINE ( 'NONE', #303, #15964 ) ;
#11641=CARTESIAN_POINT ( 'NONE',  ( -87.79934266039366264, -121.6207432329495788, 44.44620747261014770 ) ) ;
#11642=CARTESIAN_POINT ( 'NONE',  ( 87.10655032386927132, -147.8252249328912740, 49.99999999999999289 ) ) ;
#11643=CARTESIAN_POINT ( 'NONE',  ( -135.1060089022256818, -65.16414933467417825, 49.99999999999999289 ) ) ;
#11647=CARTESIAN_POINT ( 'NONE',  ( 97.63639055817486678, -133.7757280588254218, 8.337148639838481756 ) ) ;
#11649=DIRECTION ( 'NONE',  ( -0.4338837391175651703, 0.9009688679024158153, -0.000000000000000000 ) ) ;
#11653=CARTESIAN_POINT ( 'NONE',  ( 82.39904996721719499, -125.3411509769705674, 6.041691364002039322 ) ) ;
#11664=CARTESIAN_POINT ( 'NONE',  ( 4.189777606611760026E-13, -60.00000000000000000, -105.0000000000000142 ) ) ;
#11667=CARTESIAN_POINT ( 'NONE',  ( 102.7594822686537128, -126.4624059756590526, 1.189579947717209096 ) ) ;
#11668=CARTESIAN_POINT ( 'NONE',  ( -90.39157087501804710, -119.7120742831093452, -6.695055702633337269 ) ) ;
#11672=CARTESIAN_POINT ( 'NONE',  ( -82.89467276472737467, -125.0139572091430722, 3.990122295525602603 ) ) ;
#11679=ORIENTED_EDGE ( 'NONE', *, *, #18359, .T. ) ;
#11686=CARTESIAN_POINT ( 'NONE',  ( -140.0000000000000284, 1.714505518806294914E-14, -115.0000000000000142 ) ) ;
#11692=CARTESIAN_POINT ( 'NONE',  ( -133.0662791979961810, -83.15705346519905561, 1.302451894195027160 ) ) ;
#11693=DIRECTION ( 'NONE',  ( -0.3427509529624095941, -0.9394263059140722794, 0.000000000000000000 ) ) ;
#11704=EDGE_CURVE ( 'NONE', #8865, #383, #11639, .T. ) ;
#11707=FACE_BOUND ( 'NONE', #12840, .T. ) ;
#11710=DIRECTION ( 'NONE',  ( -0.000000000000000000, -0.000000000000000000, 1.000000000000000000 ) ) ;
#11713=FACE_OUTER_BOUND ( 'NONE', #7433, .T. ) ;
#11720=DIRECTION ( 'NONE',  ( 0.000000000000000000, 0.000000000000000000, -1.000000000000000000 ) ) ;
#11722=VECTOR ( 'NONE', #4631, 1000.000000000000000 ) ;
#11723=CIRCLE ( 'NONE', #307, 10.00000000000000888 ) ;
#11724=VERTEX_POINT ( 'NONE', #6944 ) ;
#11736=CIRCLE ( 'NONE', #13368, 7.500000000000007994 ) ;
#11749=ADVANCED_FACE ( 'NONE', ( #8474 ), #6556, .T. ) ;
#11754=AXIS2_PLACEMENT_3D ( 'NONE', #11763, #11857, #3804 ) ;
#11756=ORIENTED_EDGE ( 'NONE', *, *, #18359, .F. ) ;
#11761=CARTESIAN_POINT ( 'NONE',  ( 105.2664779077307884, -122.4188771607189636, 0.2361259031218233828 ) ) ;
#11762=CARTESIAN_POINT ( 'NONE',  ( -99.35657680079187060, -131.4542451999402033, 4.193517943865902708 ) ) ;
#11763=CARTESIAN_POINT ( 'NONE',  ( 144.1130761623740568, -69.50842595698583182, 10.00000000000000178 ) ) ;
#11769=EDGE_CURVE ( 'NONE', #14351, #3447, #701, .T. ) ;
#11771=DIRECTION ( 'NONE',  ( 0.000000000000000000, 0.000000000000000000, 1.000000000000000000 ) ) ;
#11772=DIRECTION ( 'NONE',  ( -0.2225209339563195554, 0.9749279121818223981, 0.000000000000000000 ) ) ;
#11774=AXIS2_PLACEMENT_3D ( 'NONE', #8854, #10289, #13246 ) ;
#11778=ORIENTED_EDGE ( 'NONE', *, *, #11500, .T. ) ;
#11781=CARTESIAN_POINT ( 'NONE',  ( 134.2873401242900968, -76.10409495552309522, 4.733913478436992506 ) ) ;
#11782=AXIS2_PLACEMENT_3D ( 'NONE', #6694, #2088, #447 ) ;
#11783=CARTESIAN_POINT ( 'NONE',  ( -130.1925331961320751, -74.50863253846083012, -6.296416515224506405 ) ) ;
#11787=CARTESIAN_POINT ( 'NONE',  ( 159.9599531637113330, -36.50981547336952104, 39.99999999999999289 ) ) ;
#11789=CARTESIAN_POINT ( 'NONE',  ( 134.5816389422699899, -73.99824545063979997, 6.893745202855313003 ) ) ;
#11793=CARTESIAN_POINT ( 'NONE',  ( -133.1725405177978985, -69.15900471360698987, 32.12259856486934240 ) ) ;
#11794=ORIENTED_EDGE ( 'NONE', *, *, #11395, .T. ) ;
#11797=ORIENTED_EDGE ( 'NONE', *, *, #16504, .F. ) ;
#11803=CARTESIAN_POINT ( 'NONE',  ( -110.0000000000000142, 265.0000000000000000, -34.99999999999997868 ) ) ;
#11808=CARTESIAN_POINT ( 'NONE',  ( -134.6712220124679220, -73.31159846691423354, 8.086032381974947114 ) ) ;
#11810=CARTESIAN_POINT ( 'NONE',  ( 128.4575182282473804, -77.52436737398417677, 40.44800108617082657 ) ) ;
#11825=CARTESIAN_POINT ( 'NONE',  ( -82.76227416097489709, -125.1020663115147755, 35.71415065638597497 ) ) ;
#11828=EDGE_CURVE ( 'NONE', #3875, #5457, #1242, .T. ) ;
#11832=CIRCLE ( 'NONE', #5650, 7.500000000000006217 ) ;
#11833=VECTOR ( 'NONE', #15258, 1000.000000000000000 ) ;
#11844=CARTESIAN_POINT ( 'NONE',  ( -110.0000000000000142, 86.60254037844390496, 39.99999999999997868 ) ) ;
#11845=AXIS2_PLACEMENT_3D ( 'NONE', #9096, #20048, #4710 ) ;
#11854=CIRCLE ( 'NONE', #13172, 42.50000000000000000 ) ;
#11856=CARTESIAN_POINT ( 'NONE',  ( -107.4999999999999716, -118.5063289449133777, -6.938893903907228378E-15 ) ) ;
#11857=DIRECTION ( 'NONE',  ( -8.294538580027652572E-17, 2.273402209432136919E-16, -1.000000000000000000 ) ) ;
#11859=CARTESIAN_POINT ( 'NONE',  ( 87.50000000000005684, -133.9542832461881403, 30.00000000000000000 ) ) ;
#11866=VERTEX_POINT ( 'NONE', #5510 ) ;
#11868=VERTEX_POINT ( 'NONE', #8573 ) ;
#11877=DIRECTION ( 'NONE',  ( -0.000000000000000000, -0.000000000000000000, -1.000000000000000000 ) ) ;
#11878=ADVANCED_FACE ( 'NONE', ( #17995 ), #12030, .T. ) ;
#11881=CARTESIAN_POINT ( 'NONE',  ( -106.9434277526348183, -119.5160896407976736, 40.00000000000000711 ) ) ;
#11885=CARTESIAN_POINT ( 'NONE',  ( 171.6840451157850111, -203.4275095296241318, 0.000000000000000000 ) ) ;
#11886=CARTESIAN_POINT ( 'NONE',  ( 134.5432410141372941, -66.31847138156594212, 3.787490405755995937 ) ) ;
#11888=CYLINDRICAL_SURFACE ( 'NONE', #6913, 150.0000000000000284 ) ;
#11890=CARTESIAN_POINT ( 'NONE',  ( -132.8875376985349135, -69.70168330572197135, 33.61525977266834531 ) ) ;
#11894=ORIENTED_EDGE ( 'NONE', *, *, #9024, .F. ) ;
#11900=CARTESIAN_POINT ( 'NONE',  ( -136.4994460260996902, -31.11111111111111427, 27.86436879316430648 ) ) ;
#11901=FACE_BOUND ( 'NONE', #15904, .T. ) ;
#11904=AXIS2_PLACEMENT_3D ( 'NONE', #12137, #5713, #15317 ) ;
#11911=CARTESIAN_POINT ( 'NONE',  ( -133.9050245804181714, -78.55577302928912786, 3.168096144027441774 ) ) ;
#11912=CIRCLE ( 'NONE', #15529, 7.500000000000007105 ) ;
#11914=FACE_OUTER_BOUND ( 'NONE', #9504, .T. ) ;
#11927=EDGE_CURVE ( 'NONE', #5660, #12327, #6543, .T. ) ;
#11934=ORIENTED_EDGE ( 'NONE', *, *, #16862, .F. ) ;
#11935=CARTESIAN_POINT ( 'NONE',  ( -189.9999999999988916, 275.0000000000000000, -2.499999999999734879 ) ) ;
#11936=CARTESIAN_POINT ( 'NONE',  ( -132.8201933467846061, -84.36756360499408913, 39.04630981318919680 ) ) ;
#11938=EDGE_LOOP ( 'NONE', ( #3645, #19614, #8406, #11517 ) ) ;
#11951=EDGE_LOOP ( 'NONE', ( #9381, #2042, #18878, #3962 ) ) ;
#11952=DIRECTION ( 'NONE',  ( -0.000000000000000000, -0.000000000000000000, 1.000000000000000000 ) ) ;
#11953=CARTESIAN_POINT ( 'NONE',  ( -100.7812499999999716, -111.0996833858562951, -10.00000000000000533 ) ) ;
#11957=CARTESIAN_POINT ( 'NONE',  ( -79.05640494597938073, -127.4758205975444270, 49.99999999999999289 ) ) ;
#11971=ORIENTED_EDGE ( 'NONE', *, *, #1033, .F. ) ;
#11982=CARTESIAN_POINT ( 'NONE',  ( -97.52493780042978244, -113.9981091059117233, 37.52868439553851232 ) ) ;
#11983=CYLINDRICAL_SURFACE ( 'NONE', #5118, 7.500000000000007105 ) ;
#11987=CARTESIAN_POINT ( 'NONE',  ( -134.9866372717062859, -65.41115948453617079, 7.014368073914691415 ) ) ;
#11988=CARTESIAN_POINT ( 'NONE',  ( 132.1020537416659693, -71.17237643005199743, 3.900420950673862741 ) ) ;
#11991=CARTESIAN_POINT ( 'NONE',  ( -134.6257061167729603, -73.66332987390026688, 32.57991584872674196 ) ) ;
#12003=CARTESIAN_POINT ( 'NONE',  ( -136.9392167837085310, -29.18162474279422725, 27.35468135938761591 ) ) ;
#12007=ORIENTED_EDGE ( 'NONE', *, *, #19765, .F. ) ;
#12008=CARTESIAN_POINT ( 'NONE',  ( -139.0264712516304826, -13.50756410634541993, -14.56951644170016458 ) ) ;
#12010=CIRCLE ( 'NONE', #13306, 150.0000000000000284 ) ;
#12013=AXIS2_PLACEMENT_3D ( 'NONE', #10723, #6138, #16975 ) ;
#12019=CARTESIAN_POINT ( 'NONE',  ( -101.6421356237309226, -200.0000000000000000, 3.469446951953614189E-15 ) ) ;
#12020=VERTEX_POINT ( 'NONE', #6328 ) ;
#12023=ORIENTED_EDGE ( 'NONE', *, *, #6161, .T. ) ;
#12030=PLANE ( 'NONE',  #17607 ) ;
#12032=EDGE_LOOP ( 'NONE', ( #2311, #13209, #7635, #3518 ) ) ;
#12035=CARTESIAN_POINT ( 'NONE',  ( -131.0911649403506658, -72.90709374210203464, 45.08599941119474863 ) ) ;
#12039=DIRECTION ( 'NONE',  ( 0.000000000000000000, 0.000000000000000000, 1.000000000000000000 ) ) ;
#12043=CARTESIAN_POINT ( 'NONE',  ( -189.9999999999988916, 275.0000000000000000, 12.50000000000027178 ) ) ;
#12046=CYLINDRICAL_SURFACE ( 'NONE', #6825, 10.00000000000000888 ) ;
#12050=CARTESIAN_POINT ( 'NONE',  ( -97.49999999999997158, -133.9542832461881972, 30.00000000000000711 ) ) ;
#12057=CARTESIAN_POINT ( 'NONE',  ( 95.49511753039645612, -115.9200926447949627, 6.565580923201594921 ) ) ;
#12058=CARTESIAN_POINT ( 'NONE',  ( -99.34007343275230539, -112.3954413154799710, 0.8360693818916272724 ) ) ;
#12062=CARTESIAN_POINT ( 'NONE',  ( 122.8001410695374602, -86.14014948502067170, -10.00000000000000178 ) ) ;
#12082=CARTESIAN_POINT ( 'NONE',  ( 130.9868171408399462, -91.88282611735539263, -10.00000000000000000 ) ) ;
#12088=CARTESIAN_POINT ( 'NONE',  ( -134.7188131032835940, -72.93593548674768101, 9.625079458299000024 ) ) ;
#12089=CARTESIAN_POINT ( 'NONE',  ( 132.0512179319785844, -87.77725330521087699, 0.2892730586186746389 ) ) ;
#12092=DIRECTION ( 'NONE',  ( -1.000000000000000000, 0.000000000000000000, 0.000000000000000000 ) ) ;
#12097=EDGE_CURVE ( 'NONE', #9886, #7766, #18342, .T. ) ;
#12102=CARTESIAN_POINT ( 'NONE',  ( -138.4878096489830170, -24.82274991483212290, 25.33558894580708198 ) ) ;
#12107=ORIENTED_EDGE ( 'NONE', *, *, #5993, .F. ) ;
#12110=DIRECTION ( 'NONE',  ( -0.5742676632334706710, 0.8186676071302499968, -0.000000000000000000 ) ) ;
#12116=CARTESIAN_POINT ( 'NONE',  ( -132.1955596402976028, -87.17962382538664201, 0.3691654002908723586 ) ) ;
#12119=DIRECTION ( 'NONE',  ( 1.000000000000000000, 0.000000000000000000, 0.000000000000000000 ) ) ;
#12120=CARTESIAN_POINT ( 'NONE',  ( -174.2942412179009466, -197.9050378206823382, 40.00000000000000000 ) ) ;
#12129=ORIENTED_EDGE ( 'NONE', *, *, #15135, .F. ) ;
#12135=EDGE_CURVE ( 'NONE', #9853, #10824, #15368, .T. ) ;
#12137=CARTESIAN_POINT ( 'NONE',  ( 0.000000000000000000, 60.00000000000000000, -105.0000000000000142 ) ) ;
#12141=CARTESIAN_POINT ( 'NONE',  ( 152.4599531637113330, -36.50981547336952104, 39.99999999999999289 ) ) ;
#12147=DIRECTION ( 'NONE',  ( 1.000000000000000000, 0.000000000000000000, 0.000000000000000000 ) ) ;
#12148=CARTESIAN_POINT ( 'NONE',  ( -107.8696296321708843, 89.24609338212388820, 39.93925132900347563 ) ) ;
#12151=DIRECTION ( 'NONE',  ( -0.3427509529624101492, 0.9394263059140720573, 0.000000000000000000 ) ) ;
#12154=AXIS2_PLACEMENT_3D ( 'NONE', #14022, #16998, #7570 ) ;
#12156=CARTESIAN_POINT ( 'NONE',  ( -82.07017599500312599, -125.5567397147592743, 31.48836724268550569 ) ) ;
#12163=LINE ( 'NONE', #5125, #2158 ) ;
#12165=AXIS2_PLACEMENT_3D ( 'NONE', #9910, #888, #2340 ) ;
#12169=DIRECTION ( 'NONE',  ( 1.000000000000000000, 0.000000000000000000, 0.000000000000000000 ) ) ;
#12173=CARTESIAN_POINT ( 'NONE',  ( 98.61625419099860324, -132.4696700755205256, 34.60511644944756426 ) ) ;
#12177=VECTOR ( 'NONE', #696, 1000.000000000000227 ) ;
#12187=CARTESIAN_POINT ( 'NONE',  ( 134.7188131032333729, -72.93593548660996362, 9.503255316708910883 ) ) ;
#12191=CARTESIAN_POINT ( 'NONE',  ( -141.6227766016837961, -18.73072656238141320, -9.999999999999985789 ) ) ;
#12192=DIRECTION ( 'NONE',  ( -0.7818314824680221431, -0.6234898018587431423, -0.000000000000000000 ) ) ;
#12195=CARTESIAN_POINT ( 'NONE',  ( -159.9599531637108782, -36.50981547337168109, 39.99999999999999289 ) ) ;
#12197=CARTESIAN_POINT ( 'NONE',  ( 127.3242258594541880, -79.35722205891387659, -0.8910983717930788250 ) ) ;
#12201=CARTESIAN_POINT ( 'NONE',  ( -134.7188131035389063, -72.93593548744735244, 30.76221486496924129 ) ) ;
#12203=CARTESIAN_POINT ( 'NONE',  ( -107.4999999999999716, -200.0000000000000000, 0.000000000000000000 ) ) ;
#12207=EDGE_LOOP ( 'NONE', ( #13180, #20194, #1707, #9065 ) ) ;
#12208=ORIENTED_EDGE ( 'NONE', *, *, #15528, .F. ) ;
#12211=CARTESIAN_POINT ( 'NONE',  ( -141.0318087585327476, -19.69042926485499478, 21.20820817219406251 ) ) ;
#12215=ORIENTED_EDGE ( 'NONE', *, *, #592, .T. ) ;
#12216=CARTESIAN_POINT ( 'NONE',  ( -136.4054103849693149, -26.47474353714355999, -17.99508669766643365 ) ) ;
#12220=CARTESIAN_POINT ( 'NONE',  ( -91.05432085726285152, 101.4279772787430574, -24.43173415096923407 ) ) ;
#12222=DIRECTION ( 'NONE',  ( 0.9009688679024154823, 0.4338837391175657809, 0.000000000000000000 ) ) ;
#12228=ORIENTED_EDGE ( 'NONE', *, *, #11828, .T. ) ;
#12229=ADVANCED_FACE ( 'NONE', ( #4581 ), #10808, .T. ) ;
#12231=EDGE_LOOP ( 'NONE', ( #1756, #7112 ) ) ;
#12234=LINE ( 'NONE', #7633, #5017 ) ;
#12235=ORIENTED_EDGE ( 'NONE', *, *, #13900, .F. ) ;
#12238=DIRECTION ( 'NONE',  ( 0.3427509529624101492, -0.9394263059140721683, 0.000000000000000000 ) ) ;
#12250=CARTESIAN_POINT ( 'NONE',  ( -134.0425641885189805, -77.70550467234690473, 36.35194583547913538 ) ) ;
#12257=EDGE_CURVE ( 'NONE', #5706, #13158, #9403, .T. ) ;
#12265=DIRECTION ( 'NONE',  ( -0.9009688679024212554, 0.4338837391175534575, 0.000000000000000000 ) ) ;
#12266=CARTESIAN_POINT ( 'NONE',  ( -181.0783081749256382, -200.0000000000000284, 40.00000000000000000 ) ) ;
#12269=CARTESIAN_POINT ( 'NONE',  ( 97.38440206417672584, -115.5262529913685654, 10.24763045490705693 ) ) ;
#12273=FACE_BOUND ( 'NONE', #10371, .T. ) ;
#12276=FACE_OUTER_BOUND ( 'NONE', #13869, .T. ) ;
#12277=CARTESIAN_POINT ( 'NONE',  ( 83.29234334534426409, -124.7495837542613799, 37.24802726318616664 ) ) ;
#12283=ORIENTED_EDGE ( 'NONE', *, *, #16466, .T. ) ;
#12285=VERTEX_POINT ( 'NONE', #16657 ) ;
#12288=CARTESIAN_POINT ( 'NONE',  ( -181.0783081749256382, -200.0000000000000284, 0.000000000000000000 ) ) ;
#12289=ORIENTED_EDGE ( 'NONE', *, *, #5, .F. ) ;
#12290=FACE_OUTER_BOUND ( 'NONE', #1502, .T. ) ;
#12292=CARTESIAN_POINT ( 'NONE',  ( -15.91767397667354800, 141.9028892025177413, 39.99999999999999289 ) ) ;
#12298=FACE_OUTER_BOUND ( 'NONE', #318, .T. ) ;
#12299=CARTESIAN_POINT ( 'NONE',  ( -134.6268015237251632, -73.65543454550571312, 7.414222461414868626 ) ) ;
#12300=CARTESIAN_POINT ( 'NONE',  ( 133.5474595738625680, -68.30173510457201758, -0.05649235984010308326 ) ) ;
#12302=CARTESIAN_POINT ( 'NONE',  ( -127.0298602564943735, -79.77387071030869947, 48.90123617796809441 ) ) ;
#12309=CARTESIAN_POINT ( 'NONE',  ( -144.1596479796006349, -15.14334797026772783, -2.639547494419652196 ) ) ;
#12310=CARTESIAN_POINT ( 'NONE',  ( 0.000000000000000000, 0.000000000000000000, -105.0000000000000142 ) ) ;
#12318=DIRECTION ( 'NONE',  ( -1.000000000000000000, 0.000000000000000000, 0.000000000000000000 ) ) ;
#12327=VERTEX_POINT ( 'NONE', #10496 ) ;
#12330=ADVANCED_FACE ( 'NONE', ( #2744 ), #8965, .F. ) ;
#12337=SURFACE_STYLE_FILL_AREA ( #1192 ) ;
#12344=EDGE_CURVE ( 'NONE', #13855, #4859, #8248, .T. ) ;
#12346=FACE_BOUND ( 'NONE', #10758, .T. ) ;
#12349=EDGE_CURVE ( 'NONE', #17792, #13097, #1816, .T. ) ;
#12350=DIRECTION ( 'NONE',  ( 1.000000000000000000, 0.000000000000000000, 0.000000000000000000 ) ) ;
#12353=CARTESIAN_POINT ( 'NONE',  ( -134.7088403748421399, -73.01573503433813528, 30.97892361658604443 ) ) ;
#12354=CARTESIAN_POINT ( 'NONE',  ( -107.3244020400115062, 89.90100472445219282, 39.90192053207060496 ) ) ;
#12355=AXIS2_PLACEMENT_3D ( 'NONE', #12082, #5969, #7491 ) ;
#12362=VERTEX_POINT ( 'NONE', #18705 ) ;
#12369=CARTESIAN_POINT ( 'NONE',  ( 96.12355554546724079, -116.0165654454190047, 9.818202592590962396 ) ) ;
#12372=AXIS2_PLACEMENT_3D ( 'NONE', #9495, #17068, #18708 ) ;
#12374=EDGE_CURVE ( 'NONE', #1323, #5389, #18215, .T. ) ;
#12376=CARTESIAN_POINT ( 'NONE',  ( -140.7803916714547086, -18.74395295176650578, -17.77646390483898386 ) ) ;
#12382=CARTESIAN_POINT ( 'NONE',  ( 96.05955731895404881, -115.3262050113700496, 35.20779912320998761 ) ) ;
#12387=AXIS2_PLACEMENT_3D ( 'NONE', #11095, #7826, #17358 ) ;
#12392=VERTEX_POINT ( 'NONE', #76 ) ;
#12393=CARTESIAN_POINT ( 'NONE',  ( -103.6585128263304938, -125.0478522927852794, 0.7634766421525948088 ) ) ;
#12395=VERTEX_POINT ( 'NONE', #17275 ) ;
#12396=DIRECTION ( 'NONE',  ( 0.6234898018587442525, -0.7818314824680211439, 0.000000000000000000 ) ) ;
#12398=CARTESIAN_POINT ( 'NONE',  ( 132.4160198941376620, -70.47193775266622140, 42.82081320361049137 ) ) ;
#12399=CARTESIAN_POINT ( 'NONE',  ( -93.44030642264235098, -117.3428525121095447, 48.41348831998372049 ) ) ;
#12406=CARTESIAN_POINT ( 'NONE',  ( -134.7188131032333445, -72.93593548660992099, 10.00000000000000533 ) ) ;
#12407=CARTESIAN_POINT ( 'NONE',  ( 123.8565975624208733, -84.62454961665271469, -0.6152758568786554916 ) ) ;
#12409=FACE_OUTER_BOUND ( 'NONE', #147, .T. ) ;
#12410=CARTESIAN_POINT ( 'NONE',  ( -132.5080654097351953, -70.41765848030097175, 35.03383174997027538 ) ) ;
#12412=ORIENTED_EDGE ( 'NONE', *, *, #18916, .T. ) ;
#12413=CARTESIAN_POINT ( 'NONE',  ( 156.4179374840099683, -52.02840013023883614, 49.99999999999999289 ) ) ;
#12416=VERTEX_POINT ( 'NONE', #15730 ) ;
#12421=DIRECTION ( 'NONE',  ( -0.000000000000000000, -0.000000000000000000, 1.000000000000000000 ) ) ;
#12423=DIRECTION ( 'NONE',  ( 1.000000000000000000, 0.000000000000000000, 0.000000000000000000 ) ) ;
#12426=CARTESIAN_POINT ( 'NONE',  ( -107.2897435581724608, 77.67224767425115317, -29.92169227468260573 ) ) ;
#12428=CARTESIAN_POINT ( 'NONE',  ( -110.0000000000000000, 275.0000000000000000, 104.9999999999999858 ) ) ;
#12432=CARTESIAN_POINT ( 'NONE',  ( 133.8517991834422105, -78.87665408946898538, 36.99948406166920023 ) ) ;
#12440=EDGE_LOOP ( 'NONE', ( #10659, #16467, #19278, #11934, #4443, #18729, #13607, #10426, #7607, #11294, #17721, #674, #3499, #9119, #10725, #17818 ) ) ;
#12444=CARTESIAN_POINT ( 'NONE',  ( -52.50000000000000000, -2.094888803305880013E-13, -105.0000000000000142 ) ) ;
#12450=CARTESIAN_POINT ( 'NONE',  ( -73.42392789539788112, 130.8023724896636679, -11.24819646464914413 ) ) ;
#12452=ADVANCED_FACE ( 'NONE', ( #7844 ), #12755, .T. ) ;
#12453=CARTESIAN_POINT ( 'NONE',  ( 176.1792632384392334, -186.5724904703758682, 10.00000000000000178 ) ) ;
#12456=CARTESIAN_POINT ( 'NONE',  ( -94.22720848804412697, 103.5554077689919410, 36.27354526481243369 ) ) ;
#12460=VERTEX_POINT ( 'NONE', #11216 ) ;
#12461=CARTESIAN_POINT ( 'NONE',  ( -63.68887634719365565, -147.8252249328922687, 49.99999999999999289 ) ) ;
#12466=PLANE ( 'NONE',  #17761 ) ;
#12474=VERTEX_POINT ( 'NONE', #8152 ) ;
#12478=CARTESIAN_POINT ( 'NONE',  ( 95.50801338652755135, -116.1654322105723480, 31.50148117855486518 ) ) ;
#12479=ORIENTED_EDGE ( 'NONE', *, *, #8530, .F. ) ;
#12483=ORIENTED_EDGE ( 'NONE', *, *, #17244, .T. ) ;
#12491=CARTESIAN_POINT ( 'NONE',  ( -105.6220017318342315, -121.8343408522481468, 0.1250734579962385629 ) ) ;
#12498=CARTESIAN_POINT ( 'NONE',  ( -100.3336596192664416, -130.0766330734951453, 36.97651187266671258 ) ) ;
#12500=CYLINDRICAL_SURFACE ( 'NONE', #8820, 42.50000000000000000 ) ;
#12502=CARTESIAN_POINT ( 'NONE',  ( 71.18887634719571622, -147.8252249328912740, 39.99999999999999289 ) ) ;
#12503=VECTOR ( 'NONE', #836, 1000.000000000000000 ) ;
#12505=DIRECTION ( 'NONE',  ( -1.000000000000000000, 0.000000000000000000, 0.000000000000000000 ) ) ;
#12507=CARTESIAN_POINT ( 'NONE',  ( -128.0993248974477581, -78.05374007935974134, 48.25206861699041383 ) ) ;
#12510=AXIS2_PLACEMENT_3D ( 'NONE', #17369, #6222, #18699 ) ;
#12517=( BOUNDED_CURVE ( )  B_SPLINE_CURVE ( 3, ( #4233, #19879, #13530, #15275 ),
 .UNSPECIFIED., .F., .F. ) 
 B_SPLINE_CURVE_WITH_KNOTS ( ( 4, 4 ),
 ( 1.570796326794896780, 3.141592653589793116 ),
 .UNSPECIFIED. ) 
 CURVE ( )  GEOMETRIC_REPRESENTATION_ITEM ( )  RATIONAL_B_SPLINE_CURVE ( ( 1.000000000000000000, 0.8047378541243650485, 0.8047378541243650485, 1.000000000000000000 ) ) 
 REPRESENTATION_ITEM ( '' )  );
#12518=B_SPLINE_CURVE_WITH_KNOTS ( 'NONE', 3,
 ( #4448, #1489, #3028, #10679, #12008, #18467, #13752, #15503, #5791, #12216, #6097, #16831 ),
 .UNSPECIFIED., .F., .F.,
 ( 4, 2, 2, 2, 2, 4 ),
 ( 0.1419734016336355320, 0.1501012059599697024, 0.1582290102863038450, 0.1622929124494709163, 0.1663568146126380154, 0.1744846189389721580 ),
 .UNSPECIFIED. ) ;
#12523=AXIS2_PLACEMENT_3D ( 'NONE', #13433, #5888, #1279 ) ;
#12529=COLOUR_RGB ( '', 0.66274510, 0.83137255, 0.94901961) ;
#12533=CARTESIAN_POINT ( 'NONE',  ( 132.8916714744556771, -69.69402298600660117, 33.62506225554120221 ) ) ;
#12536=ORIENTED_EDGE ( 'NONE', *, *, #15149, .F. ) ;
#12546=CARTESIAN_POINT ( 'NONE',  ( -97.83396368271628774, -133.5156904852161404, 32.57277006560284605 ) ) ;
#12549=DIRECTION ( 'NONE',  ( 0.000000000000000000, 0.000000000000000000, -1.000000000000000000 ) ) ;
#12551=CARTESIAN_POINT ( 'NONE',  ( 166.7850001792985495, -199.9999999999999716, 40.00000000000000000 ) ) ;
#12554=CARTESIAN_POINT ( 'NONE',  ( -84.56545567830508503, 119.8977594044767159, -25.88840230773694628 ) ) ;
#12556=CIRCLE ( 'NONE', #16166, 140.0000000000000000 ) ;
#12558=DIRECTION ( 'NONE',  ( -0.9394263059140721683, -0.3427509529624100937, 0.000000000000000000 ) ) ;
#12560=CARTESIAN_POINT ( 'NONE',  ( -84.10089422706629136, 111.9261769101578352, 28.55442653938981579 ) ) ;
#12561=ORIENTED_EDGE ( 'NONE', *, *, #18529, .T. ) ;
#12572=CARTESIAN_POINT ( 'NONE',  ( 97.26553299953100407, -115.5756973141527197, 10.32009213879923060 ) ) ;
#12575=CIRCLE ( 'NONE', #8980, 150.0000000000000284 ) ;
#12581=DIRECTION ( 'NONE',  ( 0.000000000000000000, 1.000000000000000000, 0.000000000000000000 ) ) ;
#12582=CARTESIAN_POINT ( 'NONE',  ( 97.05807359152579750, -115.6610107838044286, 29.63931307426926409 ) ) ;
#12585=CARTESIAN_POINT ( 'NONE',  ( -72.90901369577932201, 131.0915673072731806, 20.08013286166580613 ) ) ;
#12586=ORIENTED_EDGE ( 'NONE', *, *, #15653, .F. ) ;
#12588=VERTEX_POINT ( 'NONE', #17773 ) ;
#12592=ADVANCED_FACE ( 'NONE', ( #8649 ), #11616, .T. ) ;
#12593=CARTESIAN_POINT ( 'NONE',  ( -97.49999999999998579, -133.9542832461881687, 10.00000000000000178 ) ) ;
#12600=CARTESIAN_POINT ( 'NONE',  ( -87.56486837567058501, -121.7886324248894141, 44.19056895215663161 ) ) ;
#12603=CARTESIAN_POINT ( 'NONE',  ( -93.80830170559219994, -117.0490297264385617, -8.575456544257738400 ) ) ;
#12605=EDGE_CURVE ( 'NONE', #12395, #6900, #7125, .T. ) ;
#12606=CARTESIAN_POINT ( 'NONE',  ( -150.0000000000000284, 0.6141387166827441124, 4.682860153518817015 ) ) ;
#12607=EDGE_CURVE ( 'NONE', #2991, #11485, #13236, .T. ) ;
#12610=CARTESIAN_POINT ( 'NONE',  ( -131.5402663983530545, -89.84204999193647723, 39.94380265023705334 ) ) ;
#12613=AXIS2_PLACEMENT_3D ( 'NONE', #4794, #17277, #2026 ) ;
#12616=AXIS2_PLACEMENT_3D ( 'NONE', #20129, #10711, #15320 ) ;
#12617=EDGE_LOOP ( 'NONE', ( #4963, #2981, #2858, #8737 ) ) ;
#12621=CARTESIAN_POINT ( 'NONE',  ( -144.8652878778347599, -14.27854090756834360, 1.773752675255029221 ) ) ;
#12625=CARTESIAN_POINT ( 'NONE',  ( 141.8871031824808995, -16.05777877957299538, 49.99999999999999289 ) ) ;
#12631=CARTESIAN_POINT ( 'NONE',  ( 107.5000000000000142, -118.5063289449133492, 40.00000000000000000 ) ) ;
#12638=CARTESIAN_POINT ( 'NONE',  ( 134.3415992761220537, -66.72651222969517448, 37.22595600140377314 ) ) ;
#12639=CARTESIAN_POINT ( 'NONE',  ( -97.49999999999997158, -190.0000000000000000, 10.00000000000000178 ) ) ;
#12640=VERTEX_POINT ( 'NONE', #6095 ) ;
#12642=ORIENTED_EDGE ( 'NONE', *, *, #3017, .F. ) ;
#12656=ORIENTED_EDGE ( 'NONE', *, *, #4402, .F. ) ;
#12659=FACE_OUTER_BOUND ( 'NONE', #13626, .T. ) ;
#12661=EDGE_CURVE ( 'NONE', #3447, #6649, #1415, .T. ) ;
#12665=CARTESIAN_POINT ( 'NONE',  ( 83.45731665390675857, -124.6394201399246384, 37.68269516323560708 ) ) ;
#12675=CARTESIAN_POINT ( 'NONE',  ( -110.0000000000000000, 88.56916956954178488, -34.99999999999998579 ) ) ;
#12681=TOROIDAL_SURFACE ( 'NONE', #19549, 160.0000000000000284, 10.00000000000000000 ) ;
#12688=DIRECTION ( 'NONE',  ( 1.000000000000000000, 0.000000000000000000, 0.000000000000000000 ) ) ;
#12692=CARTESIAN_POINT ( 'NONE',  ( -74.02035518193302721, 130.4651978231461271, 22.50008790841033246 ) ) ;
#12697=AXIS2_PLACEMENT_3D ( 'NONE', #83, #10815, #17071 ) ;
#12700=CARTESIAN_POINT ( 'NONE',  ( -99.31036107808984070, -131.5192173896794259, 4.249900520663169701 ) ) ;
#12701=CARTESIAN_POINT ( 'NONE',  ( -146.8042373995521359, 31.12389395497865152, 20.84144971791933898 ) ) ;
#12706=CARTESIAN_POINT ( 'NONE',  ( -86.69744916218965614, -122.4084679129078381, 43.21999601890001230 ) ) ;
#12708=DIRECTION ( 'NONE',  ( -0.6234898018587431423, 0.7818314824680221431, 0.000000000000000000 ) ) ;
#12709=CARTESIAN_POINT ( 'NONE',  ( -110.0000000000000142, 265.0000000000000000, 5.000000000000000888 ) ) ;
#12712=FACE_OUTER_BOUND ( 'NONE', #7438, .T. ) ;
#12719=CARTESIAN_POINT ( 'NONE',  ( -119.5654528471588804, 59.37188176266256079, -28.72509277297836050 ) ) ;
#12720=ORIENTED_EDGE ( 'NONE', *, *, #1271, .F. ) ;
#12725=AXIS2_PLACEMENT_3D ( 'NONE', #17110, #3097, #3304 ) ;
#12726=AXIS2_PLACEMENT_3D ( 'NONE', #4047, #8653, #16539 ) ;
#12730=CARTESIAN_POINT ( 'NONE',  ( 135.7779226595531270, 102.2982297021113141, 39.99999999999999289 ) ) ;
#12742=CARTESIAN_POINT ( 'NONE',  ( 134.7088667886417284, -73.01552020433992141, 30.97729717505477609 ) ) ;
#12743=ORIENTED_EDGE ( 'NONE', *, *, #1121, .F. ) ;
#12744=ORIENTED_EDGE ( 'NONE', *, *, #19893, .T. ) ;
#12749=ORIENTED_EDGE ( 'NONE', *, *, #1979, .T. ) ;
#12752=ADVANCED_FACE ( 'NONE', ( #19990 ), #5995, .F. ) ;
#12753=CARTESIAN_POINT ( 'NONE',  ( -98.02376510503428619, -133.2645000753679199, 33.22592433350098418 ) ) ;
#12754=AXIS2_PLACEMENT_3D ( 'NONE', #2164, #14728, #5428 ) ;
#12755=CYLINDRICAL_SURFACE ( 'NONE', #10362, 10.00000000000000888 ) ;
#12758=CARTESIAN_POINT ( 'NONE',  ( 133.1207282269168388, -69.13111487717777948, -1.233265334176270267 ) ) ;
#12760=ORIENTED_EDGE ( 'NONE', *, *, #19857, .T. ) ;
#12763=PLANE ( 'NONE',  #3634 ) ;
#12767=CARTESIAN_POINT ( 'NONE',  ( 98.09575606592596841, -113.4800522715664357, 49.80233479404960661 ) ) ;
#12768=ORIENTED_EDGE ( 'NONE', *, *, #7720, .T. ) ;
#12771=ORIENTED_EDGE ( 'NONE', *, *, #10251, .F. ) ;
#12776=EDGE_LOOP ( 'NONE', ( #19690, #4313, #6842, #12743 ) ) ;
#12780=CARTESIAN_POINT ( 'NONE',  ( 85.53020504959901871, -140.9188050298377846, 39.99999999999999289 ) ) ;
#12781=ORIENTED_EDGE ( 'NONE', *, *, #4048, .T. ) ;
#12786=FACE_BOUND ( 'NONE', #476, .T. ) ;
#12793=CARTESIAN_POINT ( 'NONE',  ( -110.0000000000000142, 275.0000000000000000, -94.99999999999997158 ) ) ;
#12794=CARTESIAN_POINT ( 'NONE',  ( 96.59694518724899126, -114.7646842535148153, 49.52850901074234713 ) ) ;
#12797=CARTESIAN_POINT ( 'NONE',  ( -69.99888493010092816, 132.6655879535290694, 4.135031488835064550 ) ) ;
#12803=CARTESIAN_POINT ( 'NONE',  ( -97.49999999999998579, -133.9542832461881687, 40.00000000000000711 ) ) ;
#12804=CARTESIAN_POINT ( 'NONE',  ( -135.8037181376398905, 63.74087463549686561, 35.59253210415056401 ) ) ;
#12807=CYLINDRICAL_SURFACE ( 'NONE', #3776, 15.91767397667354800 ) ;
#12809=CARTESIAN_POINT ( 'NONE',  ( 135.1060089022256818, -65.16414933467422088, 30.00000000000000000 ) ) ;
#12812=CARTESIAN_POINT ( 'NONE',  ( -150.0000000000000000, 0.000000000000000000, 5.000000000000011546 ) ) ;
#12814=CARTESIAN_POINT ( 'NONE',  ( 0.000000000000000000, 0.000000000000000000, 40.00000000000000000 ) ) ;
#12816=EDGE_LOOP ( 'NONE', ( #7044, #8218, #19997, #2339 ) ) ;
#12825=EDGE_CURVE ( 'NONE', #19010, #17599, #5488, .T. ) ;
#12836=EDGE_LOOP ( 'NONE', ( #6877, #986, #7936, #13304, #3026, #17187, #17868 ) ) ;
#12837=EDGE_CURVE ( 'NONE', #10824, #8865, #12010, .T. ) ;
#12839=CARTESIAN_POINT ( 'NONE',  ( 131.4992782843382031, -89.99675518205300762, 39.95150868674688382 ) ) ;
#12840=EDGE_LOOP ( 'NONE', ( #4148, #16953 ) ) ;
#12847=EDGE_LOOP ( 'NONE', ( #9510, #9529, #1040, #2945, #9094 ) ) ;
#12849=CIRCLE ( 'NONE', #4028, 15.91767397667355510 ) ;
#12852=EDGE_CURVE ( 'NONE', #17320, #6137, #4661, .T. ) ;
#12857=CARTESIAN_POINT ( 'NONE',  ( 135.1060089022257102, -65.16414933467427772, 8.535171964306037751 ) ) ;
#12865=DIRECTION ( 'NONE',  ( 1.000000000000000000, 0.000000000000000000, 0.000000000000000000 ) ) ;
#12867=FACE_OUTER_BOUND ( 'NONE', #2194, .T. ) ;
#12871=CARTESIAN_POINT ( 'NONE',  ( 175.7155416004667075, -197.3864744618498719, 39.99999999999998579 ) ) ;
#12872=CIRCLE ( 'NONE', #10893, 7.500000000000020428 ) ;
#12875=DIRECTION ( 'NONE',  ( -0.4338837391175651703, 0.9009688679024157043, 0.000000000000000000 ) ) ;
#12876=ORIENTED_EDGE ( 'NONE', *, *, #5379, .F. ) ;
#12882=DIRECTION ( 'NONE',  ( 0.000000000000000000, 0.000000000000000000, 1.000000000000000000 ) ) ;
#12890=DIRECTION ( 'NONE',  ( 0.000000000000000000, 0.000000000000000000, -1.000000000000000000 ) ) ;
#12891=CARTESIAN_POINT ( 'NONE',  ( 95.54911406155098064, -115.6381493486011038, 49.24202537208733332 ) ) ;
#12892=ORIENTED_EDGE ( 'NONE', *, *, #9117, .T. ) ;
#12895=CARTESIAN_POINT ( 'NONE',  ( -75.70966155199126035, 129.4926211727434691, 25.61389564976846955 ) ) ;
#12897=AXIS2_PLACEMENT_3D ( 'NONE', #7398, #7301, #2810 ) ;
#12898=ORIENTED_EDGE ( 'NONE', *, *, #15405, .T. ) ;
#12903=CARTESIAN_POINT ( 'NONE',  ( -141.9765511393755730, 48.62330750269219237, 29.16259186082552191 ) ) ;
#12905=VECTOR ( 'NONE', #12882, 1000.000000000000000 ) ;
#12908=CARTESIAN_POINT ( 'NONE',  ( -97.78884382572438483, -133.5751867743630612, 7.606766122678530806 ) ) ;
#12911=DIRECTION ( 'NONE',  ( 1.000000000000000000, 0.000000000000000000, 0.000000000000000000 ) ) ;
#12915=CARTESIAN_POINT ( 'NONE',  ( 0.000000000000000000, 0.000000000000000000, 49.99999999999999289 ) ) ;
#12917=EDGE_LOOP ( 'NONE', ( #1512, #2708, #2579, #19436 ) ) ;
#12918=PRODUCT_DEFINITION_SHAPE ( 'NONE', 'NONE',  #17155 ) ;
#12919=CARTESIAN_POINT ( 'NONE',  ( -139.8142396999972732, 3.521345544950314377, -13.33333333333314918 ) ) ;
#12925=CYLINDRICAL_SURFACE ( 'NONE', #2092, 7.500000000000020428 ) ;
#12927=CARTESIAN_POINT ( 'NONE',  ( -135.1060089022256818, -65.16414933467419246, 9.266975799117242119 ) ) ;
#12930=CARTESIAN_POINT ( 'NONE',  ( -152.4599531637108498, -36.50981547337168109, 39.99999999999999289 ) ) ;
#12938=AXIS2_PLACEMENT_3D ( 'NONE', #18865, #6386, #15788 ) ;
#12947=CARTESIAN_POINT ( 'NONE',  ( 175.8776271403848739, -36.50981547336952104, 39.99999999999999289 ) ) ;
#12948=CARTESIAN_POINT ( 'NONE',  ( 71.18887634719571622, -147.8252249328912740, 39.99999999999999289 ) ) ;
#12950=DIRECTION ( 'NONE',  ( -1.000000000000000000, 0.000000000000000000, 0.000000000000000000 ) ) ;
#12952=CARTESIAN_POINT ( 'NONE',  ( 124.4476442249721941, -83.75451619235310829, -9.879193670931774918 ) ) ;
#12953=DIRECTION ( 'NONE',  ( 0.000000000000000000, 1.000000000000000000, 0.000000000000000000 ) ) ;
#12955=AXIS2_PLACEMENT_3D ( 'NONE', #5245, #11471, #3501 ) ;
#12962=CARTESIAN_POINT ( 'NONE',  ( 100.7812500000000000, -111.0996833858562525, 49.99999999999999289 ) ) ;
#12967=ORIENTED_EDGE ( 'NONE', *, *, #7118, .F. ) ;
#12969=CARTESIAN_POINT ( 'NONE',  ( 107.5000000000000142, -118.5063289449133492, 40.00000000000000000 ) ) ;
#12972=VECTOR ( 'NONE', #9297, 1000.000000000000000 ) ;
#12978=DIRECTION ( 'NONE',  ( 0.000000000000000000, 0.000000000000000000, -1.000000000000000000 ) ) ;
#12979=EDGE_CURVE ( 'NONE', #17599, #5045, #10067, .T. ) ;
#12981=CARTESIAN_POINT ( 'NONE',  ( 101.1837452960046875, -128.8430157189652618, 2.240558877795664205 ) ) ;
#12983=DIRECTION ( 'NONE',  ( -2.775557561562892929E-15, -1.000000000000000000, -1.734723475976808080E-16 ) ) ;
#12988=CARTESIAN_POINT ( 'NONE',  ( 82.76227416097492551, -125.1020663115147755, 4.285849343614037465 ) ) ;
#12989=CARTESIAN_POINT ( 'NONE',  ( 93.97987429418127192, -116.9112352313885026, 48.64721126355986058 ) ) ;
#12995=CARTESIAN_POINT ( 'NONE',  ( -75.26293162660911662, 129.7525693666177915, 24.85252474122213684 ) ) ;
#13001=CARTESIAN_POINT ( 'NONE',  ( -138.1756879020936424, 58.38534797887673733, 33.39972604561270941 ) ) ;
#13004=DIRECTION ( 'NONE',  ( -0.000000000000000000, -1.000000000000000000, -0.000000000000000000 ) ) ;
#13006=CARTESIAN_POINT ( 'NONE',  ( -82.95463716431548562, -124.9741831325247148, 3.790176040462246654 ) ) ;
#13007=ORIENTED_EDGE ( 'NONE', *, *, #13616, .T. ) ;
#13009=ADVANCED_FACE ( 'NONE', ( #14671 ), #12681, .F. ) ;
#13013=CARTESIAN_POINT ( 'NONE',  ( 56.84754764479240663, -154.7316448359447634, 39.99999999999999289 ) ) ;
#13015=DIRECTION ( 'NONE',  ( 0.000000000000000000, 0.000000000000000000, 1.000000000000000000 ) ) ;
#13021=ORIENTED_EDGE ( 'NONE', *, *, #14979, .T. ) ;
#13027=CARTESIAN_POINT ( 'NONE',  ( -134.6604885881914413, -66.08112487034745186, 4.281233480891749821 ) ) ;
#13034=VECTOR ( 'NONE', #4123, 1000.000000000000114 ) ;
#13035=CARTESIAN_POINT ( 'NONE',  ( 132.9399949862693404, -69.60197982539588679, 6.632446261229627993 ) ) ;
#13038=CARTESIAN_POINT ( 'NONE',  ( 99.31036107808986912, -131.5192173896793690, 35.75009947933683208 ) ) ;
#13039=DIRECTION ( 'NONE',  ( -1.000000000000000000, 0.000000000000000000, 0.000000000000000000 ) ) ;
#13042=ORIENTED_EDGE ( 'NONE', *, *, #5, .T. ) ;
#13051=VERTEX_POINT ( 'NONE', #3724 ) ;
#13052=LINE ( 'NONE', #13239, #1500 ) ;
#13056=CARTESIAN_POINT ( 'NONE',  ( -106.6474863415760979, 92.74702262351860327, -34.89460852530158519 ) ) ;
#13060=DIRECTION ( 'NONE',  ( -0.000000000000000000, 0.000000000000000000, -1.000000000000000000 ) ) ;
#13066=VECTOR ( 'NONE', #14311, 1000.000000000000000 ) ;
#13071=CARTESIAN_POINT ( 'NONE',  ( -85.34080972464063564, -123.3578596465555819, 41.36707920009423844 ) ) ;
#13077=DIRECTION ( 'NONE',  ( 0.000000000000000000, 0.000000000000000000, 1.000000000000000000 ) ) ;
#13083=CARTESIAN_POINT ( 'NONE',  ( 92.20932192393671301, -118.3126747524535602, -7.798439241158999558 ) ) ;
#13088=CARTESIAN_POINT ( 'NONE',  ( 63.68887634719570912, -147.8252249328912740, 49.99999999999999289 ) ) ;
#13096=CARTESIAN_POINT ( 'NONE',  ( 0.000000000000000000, 0.000000000000000000, 49.99999999999999289 ) ) ;
#13097=VERTEX_POINT ( 'NONE', #7588 ) ;
#13100=CARTESIAN_POINT ( 'NONE',  ( -97.37676942331958685, -115.5300780475897398, 10.30568642992988515 ) ) ;
#13108=EDGE_CURVE ( 'NONE', #16722, #18380, #20074, .T. ) ;
#13110=ADVANCED_FACE ( 'NONE', ( #13831 ), #4221, .F. ) ;
#13113=LINE ( 'NONE', #9759, #8928 ) ;
#13115=CARTESIAN_POINT ( 'NONE',  ( -123.6381990918736449, -84.94542618836281633, -9.999999999999998224 ) ) ;
#13118=CARTESIAN_POINT ( 'NONE',  ( -135.3391293778863087, -31.30995385105789808, -18.16960702786510140 ) ) ;
#13120=CARTESIAN_POINT ( 'NONE',  ( -133.5342034995409790, -80.71481093437574827, 2.145336860065035989 ) ) ;
#13122=CYLINDRICAL_SURFACE ( 'NONE', #6585, 7.500000000000001776 ) ;
#13126=EDGE_CURVE ( 'NONE', #2863, #3875, #16911, .T. ) ;
#13127=EDGE_CURVE ( 'NONE', #4551, #7267, #15292, .T. ) ;
#13130=VERTEX_POINT ( 'NONE', #12191 ) ;
#13136=EDGE_LOOP ( 'NONE', ( #7192, #13163 ) ) ;
#13137=EDGE_CURVE ( 'NONE', #18566, #17239, #18247, .T. ) ;
#13138=DIRECTION ( 'NONE',  ( 0.000000000000000000, 0.000000000000000000, 1.000000000000000000 ) ) ;
#13139=CARTESIAN_POINT ( 'NONE',  ( 122.8001410695374744, -86.14014948502065749, 49.99999999999999289 ) ) ;
#13143=AXIS2_PLACEMENT_3D ( 'NONE', #7755, #7859, #13687 ) ;
#13152=EDGE_CURVE ( 'NONE', #13130, #11373, #9435, .T. ) ;
#13154=CARTESIAN_POINT ( 'NONE',  ( -85.53020504959707182, -140.9188050298390067, 39.99999999999999289 ) ) ;
#13155=DIRECTION ( 'NONE',  ( 1.000000000000000000, 0.000000000000000000, 0.000000000000000000 ) ) ;
#13158=VERTEX_POINT ( 'NONE', #2901 ) ;
#13161=ORIENTED_EDGE ( 'NONE', *, *, #3259, .T. ) ;
#13163=ORIENTED_EDGE ( 'NONE', *, *, #5936, .F. ) ;
#13171=CARTESIAN_POINT ( 'NONE',  ( 98.51475352695847221, -132.6070668284232568, 5.590591466758980665 ) ) ;
#13172=AXIS2_PLACEMENT_3D ( 'NONE', #1041, #18444, #7384 ) ;
#13176=VECTOR ( 'NONE', #14088, 1000.000000000000000 ) ;
#13180=ORIENTED_EDGE ( 'NONE', *, *, #9252, .T. ) ;
#13187=CARTESIAN_POINT ( 'NONE',  ( -136.4994460260996902, -31.11111111111111782, -9.999999999999987566 ) ) ;
#13189=VECTOR ( 'NONE', #5685, 1000.000000000000000 ) ;
#13191=FACE_OUTER_BOUND ( 'NONE', #5753, .T. ) ;
#13193=CARTESIAN_POINT ( 'NONE',  ( -99.06221739375143898, -131.8607669219689171, 4.630169983262292455 ) ) ;
#13195=CARTESIAN_POINT ( 'NONE',  ( -137.0737990618249853, -28.59114739397107741, 27.19870260277823348 ) ) ;
#13198=CARTESIAN_POINT ( 'NONE',  ( -159.9599531637108782, -36.50981547337168109, 39.99999999999999289 ) ) ;
#13203=ORIENTED_EDGE ( 'NONE', *, *, #9894, .T. ) ;
#13206=ADVANCED_FACE ( 'NONE', ( #10553 ), #6388, .F. ) ;
#13208=ORIENTED_EDGE ( 'NONE', *, *, #3109, .F. ) ;
#13209=ORIENTED_EDGE ( 'NONE', *, *, #16283, .T. ) ;
#13212=CARTESIAN_POINT ( 'NONE',  ( 159.9599531637113330, -36.50981547336952104, 49.99999999999999289 ) ) ;
#13213=CARTESIAN_POINT ( 'NONE',  ( -132.6585078626522147, -70.01400725886476550, -2.312657259978039725 ) ) ;
#13222=CARTESIAN_POINT ( 'NONE',  ( -131.2732777714346923, -90.85536658133409560, 4.758170025484766625E-15 ) ) ;
#13226=CARTESIAN_POINT ( 'NONE',  ( -29.99999999999887379, 275.0000000000000000, 4.999999999999158007 ) ) ;
#13233=EDGE_LOOP ( 'NONE', ( #3420, #14491, #7145, #4968 ) ) ;
#13236=LINE ( 'NONE', #9988, #8747 ) ;
#13239=CARTESIAN_POINT ( 'NONE',  ( 107.5000000000000000, 1.734524432274993541E-14, 40.00000000000000000 ) ) ;
#13243=CARTESIAN_POINT ( 'NONE',  ( 144.1955966362266679, 102.2982297021113141, 39.99999999999999289 ) ) ;
#13246=DIRECTION ( 'NONE',  ( -0.6718750000000006661, 0.7406645559057077888, -6.938893903907224433E-16 ) ) ;
#13253=CARTESIAN_POINT ( 'NONE',  ( -109.9999999999983515, 265.0000000000000000, 85.00000000000001421 ) ) ;
#13254=VERTEX_POINT ( 'NONE', #7357 ) ;
#13258=AXIS2_PLACEMENT_3D ( 'NONE', #16141, #2130, #8354 ) ;
#13260=VECTOR ( 'NONE', #11424, 1000.000000000000000 ) ;
#13263=DIRECTION ( 'NONE',  ( -0.000000000000000000, -1.000000000000000000, -0.000000000000000000 ) ) ;
#13268=CARTESIAN_POINT ( 'NONE',  ( -176.1792632384392050, -186.5724904703759535, 30.00000000000000000 ) ) ;
#13274=ADVANCED_FACE ( 'NONE', ( #3470 ), #14419, .T. ) ;
#13283=( BOUNDED_CURVE ( )  B_SPLINE_CURVE ( 3, ( #14959, #15265, #15370, #10349 ),
 .UNSPECIFIED., .F., .F. ) 
 B_SPLINE_CURVE_WITH_KNOTS ( ( 4, 4 ),
 ( 1.570796326794896558, 3.141592653589793116 ),
 .UNSPECIFIED. ) 
 CURVE ( )  GEOMETRIC_REPRESENTATION_ITEM ( )  RATIONAL_B_SPLINE_CURVE ( ( 1.000000000000000000, 0.8047378541243649375, 0.8047378541243649375, 1.000000000000000000 ) ) 
 REPRESENTATION_ITEM ( '' )  );
#13284=AXIS2_PLACEMENT_3D ( 'NONE', #17205, #4720, #11050 ) ;
#13285=VERTEX_POINT ( 'NONE', #12461 ) ;
#13289=CARTESIAN_POINT ( 'NONE',  ( 95.44915936928622102, -116.0550301922294665, 7.385628739980171886 ) ) ;
#13290=CARTESIAN_POINT ( 'NONE',  ( -82.65886493343872132, -125.1699850288409408, 4.855373681067642444 ) ) ;
#13292=LINE ( 'NONE', #5641, #19298 ) ;
#13296=DIRECTION ( 'NONE',  ( 0.000000000000000000, 0.000000000000000000, 1.000000000000000000 ) ) ;
#13301=ORIENTED_EDGE ( 'NONE', *, *, #1147, .F. ) ;
#13304=ORIENTED_EDGE ( 'NONE', *, *, #11613, .F. ) ;
#13306=AXIS2_PLACEMENT_3D ( 'NONE', #6506, #11298, #3428 ) ;
#13308=AXIS2_PLACEMENT_3D ( 'NONE', #19096, #935, #5551 ) ;
#13309=CARTESIAN_POINT ( 'NONE',  ( -176.7850001792984926, -190.0000000000000284, 6.572490470375933036 ) ) ;
#13314=DIRECTION ( 'NONE',  ( 0.000000000000000000, 0.000000000000000000, 1.000000000000000000 ) ) ;
#13316=ADVANCED_FACE ( 'NONE', ( #14211 ), #4875, .F. ) ;
#13319=CARTESIAN_POINT ( 'NONE',  ( -132.0570769712681169, -87.76803911442084427, 0.2774143636855481709 ) ) ;
#13325=CARTESIAN_POINT ( 'NONE',  ( -132.7096788433825907, -70.03826381905778931, 34.33854327515700788 ) ) ;
#13327=ORIENTED_EDGE ( 'NONE', *, *, #220, .F. ) ;
#13341=ORIENTED_EDGE ( 'NONE', *, *, #5007, .F. ) ;
#13344=ADVANCED_FACE ( 'NONE', ( #11238 ), #6651, .T. ) ;
#13350=VECTOR ( 'NONE', #15999, 1000.000000000000000 ) ;
#13358=VERTEX_POINT ( 'NONE', #17496 ) ;
#13368=AXIS2_PLACEMENT_3D ( 'NONE', #18726, #3074, #12265 ) ;
#13371=EDGE_CURVE ( 'NONE', #14025, #18229, #15656, .T. ) ;
#13372=CARTESIAN_POINT ( 'NONE',  ( -135.0159133995099126, -65.35183200177806384, 32.89269165050915689 ) ) ;
#13377=DIRECTION ( 'NONE',  ( -1.613511099790691498E-16, 1.000000000000000000, -0.000000000000000000 ) ) ;
#13379=CARTESIAN_POINT ( 'NONE',  ( -150.0000000000000284, 0.000000000000000000, 49.99999999999999289 ) ) ;
#13381=AXIS2_PLACEMENT_3D ( 'NONE', #7348, #13790, #12147 ) ;
#13390=CARTESIAN_POINT ( 'NONE',  ( -133.2435246741110006, -68.89240257401093004, 30.00000000000000000 ) ) ;
#13392=ORIENTED_EDGE ( 'NONE', *, *, #17400, .T. ) ;
#13393=CARTESIAN_POINT ( 'NONE',  ( 103.0319911124603323, -126.0382377111977092, 1.048486719239181131 ) ) ;
#13394=CARTESIAN_POINT ( 'NONE',  ( -104.7095274995498357, -123.3473593051618451, 0.3789873141021475322 ) ) ;
#13399=CARTESIAN_POINT ( 'NONE',  ( 128.2779226595531270, 102.2982297021113141, 39.99999999999999289 ) ) ;
#13404=CARTESIAN_POINT ( 'NONE',  ( -109.9999999999983515, 275.0000000000000000, 85.00000000000001421 ) ) ;
#13409=ORIENTED_EDGE ( 'NONE', *, *, #4389, .T. ) ;
#13411=ADVANCED_FACE ( 'NONE', ( #11138 ), #17396, .F. ) ;
#13420=FACE_OUTER_BOUND ( 'NONE', #15018, .T. ) ;
#13433=CARTESIAN_POINT ( 'NONE',  ( 107.5000000000000000, -118.5063289449133350, -10.00000000000000355 ) ) ;
#13434=LINE ( 'NONE', #4341, #13189 ) ;
#13438=DIRECTION ( 'NONE',  ( 1.613511099790691498E-16, -1.000000000000000000, 0.000000000000000000 ) ) ;
#13441=DIRECTION ( 'NONE',  ( 1.000000000000000000, 0.000000000000000000, 0.000000000000000000 ) ) ;
#13442=EDGE_CURVE ( 'NONE', #17764, #6419, #6971, .T. ) ;
#13452=EDGE_LOOP ( 'NONE', ( #16085, #10297, #3540, #14003, #8453 ) ) ;
#13455=DIRECTION ( 'NONE',  ( -0.3427509529624095941, -0.9394263059140722794, 0.000000000000000000 ) ) ;
#13461=CARTESIAN_POINT ( 'NONE',  ( -95.40880945838063099, -115.7543288757354389, 49.20016699389176296 ) ) ;
#13466=CARTESIAN_POINT ( 'NONE',  ( -122.8001410695374460, -86.14014948502065749, 49.99999999999999289 ) ) ;
#13468=CIRCLE ( 'NONE', #7595, 150.0000000000000284 ) ;
#13472=EDGE_CURVE ( 'NONE', #18388, #5457, #14615, .T. ) ;
#13474=LINE ( 'NONE', #11935, #14305 ) ;
#13478=VERTEX_POINT ( 'NONE', #12969 ) ;
#13481=ORIENTED_EDGE ( 'NONE', *, *, #1328, .T. ) ;
#13484=CARTESIAN_POINT ( 'NONE',  ( -97.38440206417406841, -115.5262529913582341, 29.75236954509034248 ) ) ;
#13492=CARTESIAN_POINT ( 'NONE',  ( -98.69108797088911444, -112.9688971639520219, -9.907602633159209304 ) ) ;
#13495=ADVANCED_FACE ( 'NONE', ( #19429 ), #2243, .T. ) ;
#13497=DIRECTION ( 'NONE',  ( 0.000000000000000000, 1.000000000000000000, 0.000000000000000000 ) ) ;
#13500=DIRECTION ( 'NONE',  ( 1.000000000000000000, 0.000000000000000000, 0.000000000000000000 ) ) ;
#13506=ORIENTED_EDGE ( 'NONE', *, *, #5390, .T. ) ;
#13508=EDGE_LOOP ( 'NONE', ( #3049, #3469, #17114, #10440, #3883 ) ) ;
#13513=CARTESIAN_POINT ( 'NONE',  ( 42.50000000000000000, 0.000000000000000000, -100.0000000000000000 ) ) ;
#13515=CARTESIAN_POINT ( 'NONE',  ( 134.4452567384424242, -75.00213249385288350, 5.696041659366085419 ) ) ;
#13524=CARTESIAN_POINT ( 'NONE',  ( 0.000000000000000000, 164.0736214083062805, 39.99999999999999289 ) ) ;
#13525=CARTESIAN_POINT ( 'NONE',  ( -128.4575182282473804, -77.52436737398411992, -0.4480010861637727104 ) ) ;
#13526=CARTESIAN_POINT ( 'NONE',  ( 125.8775035253788843, -81.60755858752881409, -1.037139294228612618 ) ) ;
#13530=CARTESIAN_POINT ( 'NONE',  ( 101.6421356237309652, -199.9999999999999716, 39.99999999999999289 ) ) ;
#13535=ORIENTED_EDGE ( 'NONE', *, *, #10648, .T. ) ;
#13539=ORIENTED_EDGE ( 'NONE', *, *, #3498, .T. ) ;
#13540=FACE_BOUND ( 'NONE', #19099, .T. ) ;
#13545=CARTESIAN_POINT ( 'NONE',  ( -159.9599531637108782, -36.50981547337168109, 39.99999999999999289 ) ) ;
#13548=CARTESIAN_POINT ( 'NONE',  ( -110.0000000000000142, 275.0000000000000000, -67.49999999999997158 ) ) ;
#13549=CARTESIAN_POINT ( 'NONE',  ( -47.22802745636877120, -134.7565053399285091, 49.99999999999999289 ) ) ;
#13553=CARTESIAN_POINT ( 'NONE',  ( 129.0037046021668914, -76.61892870329793936, 40.13063405744939161 ) ) ;
#13560=DIRECTION ( 'NONE',  ( -1.000000000000000000, 8.881784197001252323E-16, 0.000000000000000000 ) ) ;
#13564=( NAMED_UNIT ( * ) SI_UNIT ( $, .STERADIAN. ) SOLID_ANGLE_UNIT ( ) );
#13573=EDGE_CURVE ( 'NONE', #6720, #17320, #9064, .T. ) ;
#13575=FACE_OUTER_BOUND ( 'NONE', #10005, .T. ) ;
#13580=ORIENTED_EDGE ( 'NONE', *, *, #5175, .F. ) ;
#13592=CARTESIAN_POINT ( 'NONE',  ( 71.18887634719571622, -147.8252249328912740, 49.99999999999999289 ) ) ;
#13595=CARTESIAN_POINT ( 'NONE',  ( 103.8658874391963707, -124.7161237612890687, 0.6789692764135434322 ) ) ;
#13601=CARTESIAN_POINT ( 'NONE',  ( 79.05640494598115708, -127.4758205975433043, 39.99999999999999289 ) ) ;
#13604=DIRECTION ( 'NONE',  ( 0.000000000000000000, 0.000000000000000000, 1.000000000000000000 ) ) ;
#13606=CARTESIAN_POINT ( 'NONE',  ( 107.5000000000000284, -189.9999999999999716, 40.00000000000000000 ) ) ;
#13607=ORIENTED_EDGE ( 'NONE', *, *, #14972, .T. ) ;
#13610=DIRECTION ( 'NONE',  ( 1.000000000000000000, 0.000000000000000000, 0.000000000000000000 ) ) ;
#13615=EDGE_CURVE ( 'NONE', #1562, #7965, #7602, .T. ) ;
#13616=EDGE_CURVE ( 'NONE', #2847, #6649, #12234, .T. ) ;
#13622=CARTESIAN_POINT ( 'NONE',  ( 163.5019688434126977, -20.99123081650019529, 39.99999999999999289 ) ) ;
#13623=CIRCLE ( 'NONE', #2866, 10.00000000000000888 ) ;
#13624=DIRECTION ( 'NONE',  ( 0.7818314824680220321, 0.6234898018587433643, 0.000000000000000000 ) ) ;
#13626=EDGE_LOOP ( 'NONE', ( #14725, #8585, #17093, #15869, #2741 ) ) ;
#13628=CARTESIAN_POINT ( 'NONE',  ( -132.8916714744451610, -69.69402298601710299, 6.374937744456566691 ) ) ;
#13630=CARTESIAN_POINT ( 'NONE',  ( 130.6561114389107274, -73.68416578909177872, -5.683737997257604313 ) ) ;
#13631=DIRECTION ( 'NONE',  ( 0.000000000000000000, 0.000000000000000000, -1.000000000000000000 ) ) ;
#13634=ORIENTED_EDGE ( 'NONE', *, *, #16730, .F. ) ;
#13637=AXIS2_PLACEMENT_3D ( 'NONE', #3857, #11720, #10192 ) ;
#13643=EDGE_LOOP ( 'NONE', ( #1061, #12561, #11080, #15294 ) ) ;
#13646=FACE_BOUND ( 'NONE', #7703, .T. ) ;
#13648=EDGE_LOOP ( 'NONE', ( #8534, #6920, #6412, #983 ) ) ;
#13649=CARTESIAN_POINT ( 'NONE',  ( 77.50000000000000000, 0.000000000000000000, -105.0000000000000142 ) ) ;
#13653=CARTESIAN_POINT ( 'NONE',  ( -88.33722569973700445, 105.0987966894255550, -22.54091672644404909 ) ) ;
#13657=CARTESIAN_POINT ( 'NONE',  ( -132.8189972983174698, -84.37332251142817086, 0.9521473212757564086 ) ) ;
#13659=CARTESIAN_POINT ( 'NONE',  ( 123.8648416762537039, -84.61253400034586036, 40.61864639473208172 ) ) ;
#13660=CYLINDRICAL_SURFACE ( 'NONE', #10645, 10.00000000000000888 ) ;
#13664=ORIENTED_EDGE ( 'NONE', *, *, #5833, .T. ) ;
#13667=VERTEX_POINT ( 'NONE', #8864 ) ;
#13671=DIRECTION ( 'NONE',  ( 0.000000000000000000, 0.000000000000000000, 1.000000000000000000 ) ) ;
#13673=DIRECTION ( 'NONE',  ( 0.7818314824680220321, 0.6234898018587433643, 0.000000000000000000 ) ) ;
#13675=CARTESIAN_POINT ( 'NONE',  ( 107.5000000000000284, -199.9999999999999716, 10.00000000000000178 ) ) ;
#13678=DIRECTION ( 'NONE',  ( 0.000000000000000000, 1.000000000000000000, 0.000000000000000000 ) ) ;
#13686=DIRECTION ( 'NONE',  ( 0.000000000000000000, 0.000000000000000000, 1.000000000000000000 ) ) ;
#13687=DIRECTION ( 'NONE',  ( 1.000000000000000000, 0.000000000000000000, 0.000000000000000000 ) ) ;
#13690=CYLINDRICAL_SURFACE ( 'NONE', #7953, 39.99999999999997868 ) ;
#13693=ORIENTED_EDGE ( 'NONE', *, *, #398, .F. ) ;
#13696=CIRCLE ( 'NONE', #2598, 110.0000000000000142 ) ;
#13701=VERTEX_POINT ( 'NONE', #16745 ) ;
#13702=CARTESIAN_POINT ( 'NONE',  ( 82.23581699221259100, -125.4482974261017745, 7.029979419219573700 ) ) ;
#13704=CARTESIAN_POINT ( 'NONE',  ( -136.2020012053989433, -31.16171794781974214, -14.16315223586064498 ) ) ;
#13706=FACE_BOUND ( 'NONE', #5192, .T. ) ;
#13712=CARTESIAN_POINT ( 'NONE',  ( 95.72167172977059124, -116.1306513017061519, 30.88982041833051539 ) ) ;
#13716=EDGE_LOOP ( 'NONE', ( #1296, #14338, #15247, #14833, #15332, #19816, #10812, #3825, #4711, #14112, #11422 ) ) ;
#13725=CARTESIAN_POINT ( 'NONE',  ( 134.6261364156840159, -73.66016459667361005, 7.423013666676803624 ) ) ;
#13732=CARTESIAN_POINT ( 'NONE',  ( -132.3557670345054191, -70.70247614046988360, 4.526726988747244107 ) ) ;
#13733=ADVANCED_FACE ( 'NONE', ( #20220 ), #3051, .F. ) ;
#13734=CARTESIAN_POINT ( 'NONE',  ( 130.0531662534324937, -74.83651286709024930, 0.7279510403262877682 ) ) ;
#13737=CARTESIAN_POINT ( 'NONE',  ( -132.7722305162506302, -69.92010858955688946, 34.10135643643651093 ) ) ;
#13740=FACE_OUTER_BOUND ( 'NONE', #17585, .T. ) ;
#13743=ORIENTED_EDGE ( 'NONE', *, *, #4016, .F. ) ;
#13750=ORIENTED_EDGE ( 'NONE', *, *, #5310, .F. ) ;
#13752=CARTESIAN_POINT ( 'NONE',  ( -138.1826048463154279, -18.76197922584882960, -15.75885094356106464 ) ) ;
#13754=ORIENTED_EDGE ( 'NONE', *, *, #19486, .T. ) ;
#13755=CARTESIAN_POINT ( 'NONE',  ( -93.08628513671655469, 98.60439646660965707, -25.65138098760644425 ) ) ;
#13757=CARTESIAN_POINT ( 'NONE',  ( -133.3649390995068984, -81.63041515106807822, 1.796504641981583550 ) ) ;
#13763=UNCERTAINTY_MEASURE_WITH_UNIT (LENGTH_MEASURE( 1.000000000000000082E-05 ), #3711, 'distance_accuracy_value', 'NONE');
#13764=CARTESIAN_POINT ( 'NONE',  ( 131.5441688916729390, -89.82688951536542277, 39.94263630573486523 ) ) ;
#13777=DIRECTION ( 'NONE',  ( -0.9749279121818226201, -0.2225209339563185285, 0.000000000000000000 ) ) ;
#13781=DIRECTION ( 'NONE',  ( 1.000000000000000000, 0.000000000000000000, 0.000000000000000000 ) ) ;
#13782=ORIENTED_EDGE ( 'NONE', *, *, #17006, .T. ) ;
#13785=EDGE_CURVE ( 'NONE', #11258, #2863, #1810, .T. ) ;
#13786=DIRECTION ( 'NONE',  ( -0.4338837391175651703, 0.9009688679024158153, -0.000000000000000000 ) ) ;
#13788=CIRCLE ( 'NONE', #11193, 10.00000000000000711 ) ;
#13790=DIRECTION ( 'NONE',  ( 0.000000000000000000, 0.000000000000000000, 1.000000000000000000 ) ) ;
#13794=DIRECTION ( 'NONE',  ( 0.000000000000000000, 0.000000000000000000, 1.000000000000000000 ) ) ;
#13799=CARTESIAN_POINT ( 'NONE',  ( -82.35314629726805435, -125.3713054028917071, 33.70901503745690064 ) ) ;
#13803=CIRCLE ( 'NONE', #3043, 7.500000000000007105 ) ;
#13806=CARTESIAN_POINT ( 'NONE',  ( 82.42180963433075647, -125.3261898519401001, 5.922222528876336156 ) ) ;
#13808=VECTOR ( 'NONE', #13455, 1000.000000000000114 ) ;
#13809=CARTESIAN_POINT ( 'NONE',  ( -141.4430087160396283, -18.68139018776262006, -13.92791448115454678 ) ) ;
#13814=CARTESIAN_POINT ( 'NONE',  ( 89.41572940475639086, -120.4415366094430482, 45.96144366595092379 ) ) ;
#13817=DIRECTION ( 'NONE',  ( -0.6234898018587431423, 0.7818314824680221431, 0.000000000000000000 ) ) ;
#13818=AXIS2_PLACEMENT_3D ( 'NONE', #9803, #4915, #8265 ) ;
#13826=LINE ( 'NONE', #18657, #3378 ) ;
#13827=DIRECTION ( 'NONE',  ( 0.4338837391175654479, -0.9009688679024155933, 0.000000000000000000 ) ) ;
#13829=DIRECTION ( 'NONE',  ( -0.000000000000000000, -0.000000000000000000, -1.000000000000000000 ) ) ;
#13830=CIRCLE ( 'NONE', #8611, 7.500000000000020428 ) ;
#13831=FACE_OUTER_BOUND ( 'NONE', #19068, .T. ) ;
#13836=CARTESIAN_POINT ( 'NONE',  ( 129.7375433114042096, -75.28992114163500560, -6.767788122726502209 ) ) ;
#13837=ADVANCED_BREP_SHAPE_REPRESENTATION ( '', ( #1054, #18639 ), #15396 ) ;
#13838=CIRCLE ( 'NONE', #1437, 39.99999999999997868 ) ;
#13841=CARTESIAN_POINT ( 'NONE',  ( -132.3553460543473932, -70.70324312376081366, 35.47401752195474245 ) ) ;
#13843=VERTEX_POINT ( 'NONE', #1611 ) ;
#13844=PLANE ( 'NONE',  #16103 ) ;
#13854=CARTESIAN_POINT ( 'NONE',  ( -97.49999999999997158, -195.8578643762690206, 35.85786437626905609 ) ) ;
#13855=VERTEX_POINT ( 'NONE', #17164 ) ;
#13857=CYLINDRICAL_SURFACE ( 'NONE', #9463, 77.50000000000000000 ) ;
#13858=ORIENTED_EDGE ( 'NONE', *, *, #15106, .T. ) ;
#13861=CARTESIAN_POINT ( 'NONE',  ( 176.1792632384392334, -186.5724904703758682, 10.00000000000000178 ) ) ;
#13864=EDGE_CURVE ( 'NONE', #13158, #5706, #15138, .T. ) ;
#13865=CARTESIAN_POINT ( 'NONE',  ( 123.6158562626681032, -84.97727779989052976, 49.99999999947959139 ) ) ;
#13869=EDGE_LOOP ( 'NONE', ( #14463, #18933 ) ) ;
#13884=DIRECTION ( 'NONE',  ( 0.000000000000000000, -1.000000000000000000, -3.469446951953611231E-16 ) ) ;
#13885=CARTESIAN_POINT ( 'NONE',  ( 97.50000000000002842, -189.9999999999999716, 30.00000000000000000 ) ) ;
#13887=PLANE ( 'NONE',  #12616 ) ;
#13892=CARTESIAN_POINT ( 'NONE',  ( -134.3956174703911017, -75.35551001548425631, 34.63745171344068297 ) ) ;
#13895=CARTESIAN_POINT ( 'NONE',  ( -110.0000000000000142, 275.0000000000000000, 5.000000000000000888 ) ) ;
#13900=EDGE_CURVE ( 'NONE', #12588, #16701, #5290, .T. ) ;
#13902=AXIS2_PLACEMENT_3D ( 'NONE', #1182, #7428, #7234 ) ;
#13917=CARTESIAN_POINT ( 'NONE',  ( 97.49999999944091655, -115.4778303847715790, 29.84273253271013360 ) ) ;
#13918=AXIS2_PLACEMENT_3D ( 'NONE', #11301, #17558, #6706 ) ;
#13922=DIRECTION ( 'NONE',  ( -0.000000000000000000, 0.000000000000000000, -1.000000000000000000 ) ) ;
#13923=ORIENTED_EDGE ( 'NONE', *, *, #10212, .T. ) ;
#13928=CARTESIAN_POINT ( 'NONE',  ( -102.1629267457074093, -127.3823967956317347, 1.521494987488698269 ) ) ;
#13930=VERTEX_POINT ( 'NONE', #17575 ) ;
#13933=CARTESIAN_POINT ( 'NONE',  ( -82.03124999999998579, -125.5821405433014348, 9.999999999999991118 ) ) ;
#13936=CARTESIAN_POINT ( 'NONE',  ( -85.50395135567417526, -123.2448845699152002, 41.61540074481813178 ) ) ;
#13937=CARTESIAN_POINT ( 'NONE',  ( -130.9868171408399462, -91.88282611735537841, 40.00000000000000000 ) ) ;
#13941=CARTESIAN_POINT ( 'NONE',  ( 125.9179923520548954, -81.51769904231269948, -9.421453882809895930 ) ) ;
#13944=CARTESIAN_POINT ( 'NONE',  ( -132.0132531075724671, -71.33615934021206328, 36.30293437782199106 ) ) ;
#13952=CARTESIAN_POINT ( 'NONE',  ( -143.6837422564963163, -15.75497795184483962, -4.519904249420592102 ) ) ;
#13960=CARTESIAN_POINT ( 'NONE',  ( -104.5717993161247676, 81.74765234771037115, -29.58341083972238295 ) ) ;
#13967=EDGE_CURVE ( 'NONE', #7556, #18388, #12849, .T. ) ;
#13968=CARTESIAN_POINT ( 'NONE',  ( 130.0420013710427156, -74.85033908745178621, 39.25082761537147036 ) ) ;
#13970=ORIENTED_EDGE ( 'NONE', *, *, #7661, .T. ) ;
#13971=EDGE_CURVE ( 'NONE', #10778, #1323, #8344, .T. ) ;
#13974=VERTEX_POINT ( 'NONE', #15183 ) ;
#13979=EDGE_CURVE ( 'NONE', #961, #10982, #15810, .T. ) ;
#13983=CARTESIAN_POINT ( 'NONE',  ( 0.000000000000000000, 0.000000000000000000, -105.0000000000000142 ) ) ;
#13996=CARTESIAN_POINT ( 'NONE',  ( -75.21424932920895401, 118.0797154971734386, 8.890256474989355340 ) ) ;
#14000=EDGE_CURVE ( 'NONE', #17652, #5526, #4699, .T. ) ;
#14003=ORIENTED_EDGE ( 'NONE', *, *, #14979, .F. ) ;
#14006=ORIENTED_EDGE ( 'NONE', *, *, #4478, .F. ) ;
#14007=CARTESIAN_POINT ( 'NONE',  ( -137.1611395155196931, 53.79589955330019535, -24.36911571694407996 ) ) ;
#14009=DIRECTION ( 'NONE',  ( -3.320906611023727849E-16, 1.000000000000000000, 0.000000000000000000 ) ) ;
#14011=CARTESIAN_POINT ( 'NONE',  ( 85.50395135567664795, -123.2448845699134807, -1.615400744817004464 ) ) ;
#14021=EDGE_CURVE ( 'NONE', #4416, #13130, #11493, .T. ) ;
#14022=CARTESIAN_POINT ( 'NONE',  ( 0.000000000000000000, 0.000000000000000000, -49.99999999999999289 ) ) ;
#14023=CARTESIAN_POINT ( 'NONE',  ( 97.78884382572414324, -133.5751867743630328, 32.39323387732022752 ) ) ;
#14025=VERTEX_POINT ( 'NONE', #11295 ) ;
#14026=EDGE_CURVE ( 'NONE', #9222, #15878, #8221, .T. ) ;
#14031=VECTOR ( 'NONE', #14471, 1000.000000000000000 ) ;
#14037=CARTESIAN_POINT ( 'NONE',  ( 15.91767397667354800, 164.0736214083062805, 39.99999999999999289 ) ) ;
#14038=EDGE_CURVE ( 'NONE', #796, #19032, #13113, .T. ) ;
#14044=CARTESIAN_POINT ( 'NONE',  ( -88.24590234222469576, -121.2961002105598141, 44.87695375404122444 ) ) ;
#14047=CARTESIAN_POINT ( 'NONE',  ( -99.70727046260189752, -112.0668231182906283, -9.975445138866367856 ) ) ;
#14048=DIRECTION ( 'NONE',  ( 0.000000000000000000, 1.000000000000000000, 0.000000000000000000 ) ) ;
#14053=CARTESIAN_POINT ( 'NONE',  ( -131.7304022393908269, -71.85445963696412264, 36.89128936748223708 ) ) ;
#14056=EDGE_CURVE ( 'NONE', #12474, #14128, #10887, .T. ) ;
#14060=AXIS2_PLACEMENT_3D ( 'NONE', #18972, #12708, #4957 ) ;
#14061=VERTEX_POINT ( 'NONE', #17950 ) ;
#14063=CARTESIAN_POINT ( 'NONE',  ( -143.2800199296550829, -16.29095325894156332, -5.878076611359963621 ) ) ;
#14075=CARTESIAN_POINT ( 'NONE',  ( 134.7188131032758349, -72.93593548672635052, 30.37492054169907618 ) ) ;
#14077=VERTEX_POINT ( 'NONE', #6602 ) ;
#14079=EDGE_LOOP ( 'NONE', ( #9788, #15521, #4677, #2583 ) ) ;
#14088=DIRECTION ( 'NONE',  ( 0.000000000000000000, 0.000000000000000000, 1.000000000000000000 ) ) ;
#14093=ORIENTED_EDGE ( 'NONE', *, *, #7118, .T. ) ;
#14094=CARTESIAN_POINT ( 'NONE',  ( -83.77529404233767707, 120.7950752208005696, -25.22193715514223200 ) ) ;
#14098=DIRECTION ( 'NONE',  ( 1.000000000000000000, 0.000000000000000000, 0.000000000000000000 ) ) ;
#14103=CARTESIAN_POINT ( 'NONE',  ( 178.1870518357299602, -192.0755223619198944, 35.85786437626904899 ) ) ;
#14105=ORIENTED_EDGE ( 'NONE', *, *, #16504, .T. ) ;
#14108=ADVANCED_FACE ( 'NONE', ( #6703 ), #12925, .F. ) ;
#14109=CARTESIAN_POINT ( 'NONE',  ( -116.9645463067439124, 79.99640762678326666, -34.39232645276845801 ) ) ;
#14112=ORIENTED_EDGE ( 'NONE', *, *, #19423, .T. ) ;
#14114=CARTESIAN_POINT ( 'NONE',  ( 95.47048624633011116, -116.1260213179369316, 8.021552276157979833 ) ) ;
#14123=DIRECTION ( 'NONE',  ( -0.2225209339563047894, -0.9749279121818258398, 0.000000000000000000 ) ) ;
#14127=CARTESIAN_POINT ( 'NONE',  ( -70.93787238057718980, 132.1659262131047967, 13.62312833148349434 ) ) ;
#14128=VERTEX_POINT ( 'NONE', #8428 ) ;
#14129=EDGE_LOOP ( 'NONE', ( #16259, #13750, #8018, #18437 ) ) ;
#14133=AXIS2_PLACEMENT_3D ( 'NONE', #546, #18030, #19272 ) ;
#14142=CARTESIAN_POINT ( 'NONE',  ( 135.1060089022256818, -65.16414933467422088, 30.73302420088275966 ) ) ;
#14144=EDGE_CURVE ( 'NONE', #14128, #15721, #14493, .T. ) ;
#14145=CARTESIAN_POINT ( 'NONE',  ( -95.52811048055527010, -116.1520858409645314, 31.53047640601787194 ) ) ;
#14149=CARTESIAN_POINT ( 'NONE',  ( -149.9810182027019891, 2.464479588725518866, 3.727447874301266673 ) ) ;
#14154=CARTESIAN_POINT ( 'NONE',  ( -124.3929425833997300, -83.83509237770859102, 49.88760530048027420 ) ) ;
#14159=B_SPLINE_CURVE_WITH_KNOTS ( 'NONE', 3,
 ( #2551, #810, #19443, #909, #714, #18102, #11653, #12988, #8787, #17910, #4076, #10311, #3977, #19630, #5524, #8589, #3688, #8685, #7061, #6765, #19535, #11459, #13083, #11559, #18009, #17714, #3887, #10217, #10129, #8491 ),
 .UNSPECIFIED., .F., .F.,
 ( 4, 2, 2, 2, 2, 2, 2, 2, 2, 2, 2, 2, 2, 2, 4 ),
 ( 0.000000000000000000, 0.002172065812121079086, 0.003258098718181618413, 0.004344131624242158173, 0.008688263248484319815, 0.009774296154544852636, 0.01086032906060538719, 0.01303239487272645457, 0.01520446068484752195, 0.01737652649696859106, 0.02172065812121067377, 0.02389272393333173247, 0.02606478974545278771, 0.03040892136969489123, 0.03475305299393700170 ),
 .UNSPECIFIED. ) ;
#14161=ORIENTED_EDGE ( 'NONE', *, *, #10251, .T. ) ;
#14167=EDGE_CURVE ( 'NONE', #2173, #4551, #16144, .T. ) ;
#14172=LINE ( 'NONE', #12625, #19477 ) ;
#14179=LINE ( 'NONE', #14580, #29 ) ;
#14182=CARTESIAN_POINT ( 'NONE',  ( 135.0821395827860272, -65.21370709269135091, 31.49693204037136596 ) ) ;
#14183=CARTESIAN_POINT ( 'NONE',  ( 133.6066233479226071, -80.29760051435188473, 37.66252863624313818 ) ) ;
#14185=ORIENTED_EDGE ( 'NONE', *, *, #2295, .F. ) ;
#14187=ORIENTED_EDGE ( 'NONE', *, *, #14835, .F. ) ;
#14190=VERTEX_POINT ( 'NONE', #4017 ) ;
#14195=CARTESIAN_POINT ( 'NONE',  ( 148.9554720520395108, -17.67108784863215121, 49.99999999999999289 ) ) ;
#14196=ORIENTED_EDGE ( 'NONE', *, *, #1788, .F. ) ;
#14197=LINE ( 'NONE', #9494, #14209 ) ;
#14205=CARTESIAN_POINT ( 'NONE',  ( 100.2452644940503461, -111.5858889953167363, 50.00000000000000000 ) ) ;
#14209=VECTOR ( 'NONE', #9889, 1000.000000000000000 ) ;
#14210=ORIENTED_EDGE ( 'NONE', *, *, #10581, .F. ) ;
#14211=FACE_OUTER_BOUND ( 'NONE', #5170, .T. ) ;
#14220=DIRECTION ( 'NONE',  ( 0.000000000000000000, 0.000000000000000000, -1.000000000000000000 ) ) ;
#14223=LINE ( 'NONE', #15558, #672 ) ;
#14225=ORIENTED_EDGE ( 'NONE', *, *, #12605, .F. ) ;
#14229=CARTESIAN_POINT ( 'NONE',  ( 107.5000000000000142, -118.5063289449133492, 40.00000000000000000 ) ) ;
#14231=EDGE_CURVE ( 'NONE', #5623, #18014, #11854, .T. ) ;
#14233=CARTESIAN_POINT ( 'NONE',  ( -70.22158424196186388, 132.5482456588196669, 9.581993153685951725 ) ) ;
#14236=AXIS2_PLACEMENT_3D ( 'NONE', #12709, #14048, #9448 ) ;
#14239=ORIENTED_EDGE ( 'NONE', *, *, #1147, .T. ) ;
#14243=CARTESIAN_POINT ( 'NONE',  ( -138.6264652121188590, 57.30678207472260510, 32.94515158125864218 ) ) ;
#14247=CARTESIAN_POINT ( 'NONE',  ( 128.2054629363889831, -77.87043913366069603, 48.14259967130468709 ) ) ;
#14249=CARTESIAN_POINT ( 'NONE',  ( -83.97601510866861929, -124.2902204837763378, 38.87704193713654632 ) ) ;
#14252=CARTESIAN_POINT ( 'NONE',  ( -110.0000000000000142, 86.60254037844390496, 39.99999999999997868 ) ) ;
#14254=CARTESIAN_POINT ( 'NONE',  ( -148.7883939290497608, 19.65460682028593808, -5.098580071606036768 ) ) ;
#14256=LINE ( 'NONE', #11178, #13350 ) ;
#14257=CARTESIAN_POINT ( 'NONE',  ( -134.2478682171874027, -76.37034190854926408, 35.46671602548207858 ) ) ;
#14258=ORIENTED_EDGE ( 'NONE', *, *, #7642, .F. ) ;
#14260=CARTESIAN_POINT ( 'NONE',  ( -125.9580719609004973, 49.35695123619169777, -26.15414125452645067 ) ) ;
#14261=EDGE_CURVE ( 'NONE', #12460, #8838, #225, .T. ) ;
#14266=CIRCLE ( 'NONE', #16876, 15.91767397667354444 ) ;
#14268=CARTESIAN_POINT ( 'NONE',  ( -144.6246557071403060, -14.56788443266039579, -0.2086646817306959945 ) ) ;
#14279=DIRECTION ( 'NONE',  ( 0.000000000000000000, 0.000000000000000000, -1.000000000000000000 ) ) ;
#14283=CARTESIAN_POINT ( 'NONE',  ( 132.7769743428758886, -69.91161917917226276, 34.10605816523012379 ) ) ;
#14289=ORIENTED_EDGE ( 'NONE', *, *, #3259, .F. ) ;
#14297=CARTESIAN_POINT ( 'NONE',  ( -105.6231002115456903, -121.8324894761443886, 39.87517067041968488 ) ) ;
#14301=DIRECTION ( 'NONE',  ( 0.000000000000000000, 1.000000000000000000, 0.000000000000000000 ) ) ;
#14302=CARTESIAN_POINT ( 'NONE',  ( -189.9999999999988916, 265.0000000000000000, 5.000000000000268230 ) ) ;
#14305=VECTOR ( 'NONE', #10818, 1000.000000000000000 ) ;
#14307=CARTESIAN_POINT ( 'NONE',  ( -98.33690426217857805, 103.1883475260306398, -33.27187555683841680 ) ) ;
#14311=DIRECTION ( 'NONE',  ( -0.000000000000000000, -1.000000000000000000, -0.000000000000000000 ) ) ;
#14312=DIRECTION ( 'NONE',  ( 0.9749279121818227312, 0.2225209339563182509, 0.000000000000000000 ) ) ;
#14322=DIRECTION ( 'NONE',  ( -3.129754055707530415E-16, 1.000000000000000000, -0.000000000000000000 ) ) ;
#14326=DIRECTION ( 'NONE',  ( 1.000000000000000000, 0.000000000000000000, 0.000000000000000000 ) ) ;
#14330=DIRECTION ( 'NONE',  ( -1.000000000000000000, 0.000000000000000000, 0.000000000000000000 ) ) ;
#14335=FACE_OUTER_BOUND ( 'NONE', #15453, .T. ) ;
#14336=LINE ( 'NONE', #9527, #6872 ) ;
#14338=ORIENTED_EDGE ( 'NONE', *, *, #19019, .T. ) ;
#14341=ORIENTED_EDGE ( 'NONE', *, *, #9279, .F. ) ;
#14347=VERTEX_POINT ( 'NONE', #17015 ) ;
#14348=AXIS2_PLACEMENT_3D ( 'NONE', #7589, #18345, #514 ) ;
#14351=VERTEX_POINT ( 'NONE', #4846 ) ;
#14356=VECTOR ( 'NONE', #3809, 1000.000000000000000 ) ;
#14357=CARTESIAN_POINT ( 'NONE',  ( -98.09575606592595420, -113.4800522715664641, -9.802334794049597733 ) ) ;
#14362=VECTOR ( 'NONE', #17923, 1000.000000000000000 ) ;
#14363=CARTESIAN_POINT ( 'NONE',  ( 0.000000000000000000, 0.000000000000000000, -39.99999999999999289 ) ) ;
#14368=EDGE_LOOP ( 'NONE', ( #9196, #19427, #12760, #14829, #12235, #12479 ) ) ;
#14369=ORIENTED_EDGE ( 'NONE', *, *, #8360, .T. ) ;
#14372=AXIS2_PLACEMENT_3D ( 'NONE', #13545, #4346, #19794 ) ;
#14374=ADVANCED_FACE ( 'NONE', ( #31 ), #1358, .F. ) ;
#14375=DIRECTION ( 'NONE',  ( 1.000000000000000000, 0.000000000000000000, 0.000000000000000000 ) ) ;
#14378=CARTESIAN_POINT ( 'NONE',  ( 0.000000000000000000, 0.000000000000000000, 39.99999999999999289 ) ) ;
#14381=CARTESIAN_POINT ( 'NONE',  ( 106.5742148451190019, -120.1859338240075203, 39.99999999999999289 ) ) ;
#14382=CARTESIAN_POINT ( 'NONE',  ( -189.9999999999988916, 275.0000000000000000, 12.50000000000027178 ) ) ;
#14385=CARTESIAN_POINT ( 'NONE',  ( 132.5095042660555293, -70.41495930837207595, 35.02927749617933273 ) ) ;
#14386=CARTESIAN_POINT ( 'NONE',  ( 0.000000000000000000, 0.000000000000000000, -105.0000000000000142 ) ) ;
#14387=ORIENTED_EDGE ( 'NONE', *, *, #6031, .F. ) ;
#14395=DIRECTION ( 'NONE',  ( -0.000000000000000000, -0.000000000000000000, 1.000000000000000000 ) ) ;
#14396=CARTESIAN_POINT ( 'NONE',  ( -166.7850001792984926, -190.0000000000000284, 40.00000000000000000 ) ) ;
#14398=EDGE_CURVE ( 'NONE', #5578, #2667, #13838, .T. ) ;
#14399=VECTOR ( 'NONE', #10993, 1000.000000000000000 ) ;
#14400=CARTESIAN_POINT ( 'NONE',  ( 129.8775639978177026, -75.04816271247871384, -6.616949551716221123 ) ) ;
#14404=LINE ( 'NONE', #6637, #7077 ) ;
#14417=CIRCLE ( 'NONE', #4951, 15.91767397667354444 ) ;
#14419=CYLINDRICAL_SURFACE ( 'NONE', #17288, 150.0000000000000284 ) ;
#14426=CARTESIAN_POINT ( 'NONE',  ( 144.1130761623740568, -69.50842595698583182, 30.00000000000000000 ) ) ;
#14445=ORIENTED_EDGE ( 'NONE', *, *, #17235, .T. ) ;
#14447=CARTESIAN_POINT ( 'NONE',  ( -148.9537812787172300, 17.82720812061743842, 14.16315103253250918 ) ) ;
#14448=EDGE_LOOP ( 'NONE', ( #20064, #20190, #11797, #7706 ) ) ;
#14452=CARTESIAN_POINT ( 'NONE',  ( -103.8725996235353222, -124.7053175801541158, 0.6763943681471633607 ) ) ;
#14453=CARTESIAN_POINT ( 'NONE',  ( -133.5605114351387499, 42.14324244569257871, 30.93267679371781043 ) ) ;
#14457=DIRECTION ( 'NONE',  ( -1.000000000000000000, 0.000000000000000000, 0.000000000000000000 ) ) ;
#14459=EDGE_LOOP ( 'NONE', ( #15256, #19515 ) ) ;
#14460=CARTESIAN_POINT ( 'NONE',  ( -134.1501013333374033, 33.24937751378277540, -20.37878451202398367 ) ) ;
#14463=ORIENTED_EDGE ( 'NONE', *, *, #2284, .T. ) ;
#14466=CARTESIAN_POINT ( 'NONE',  ( 159.9599531637113330, -36.50981547336952104, 49.99999999999999289 ) ) ;
#14471=DIRECTION ( 'NONE',  ( 0.000000000000000000, 0.000000000000000000, 1.000000000000000000 ) ) ;
#14478=CYLINDRICAL_SURFACE ( 'NONE', #14942, 7.500000000000000000 ) ;
#14482=VERTEX_POINT ( 'NONE', #6973 ) ;
#14491=ORIENTED_EDGE ( 'NONE', *, *, #20172, .F. ) ;
#14493=CIRCLE ( 'NONE', #8603, 15.91767397667354444 ) ;
#14497=CARTESIAN_POINT ( 'NONE',  ( 0.000000000000000000, 164.0736214083062805, 49.99999999999999289 ) ) ;
#14499=CARTESIAN_POINT ( 'NONE',  ( 127.1451880273207280, -79.59002392720331898, -8.837124157530666935 ) ) ;
#14507=CARTESIAN_POINT ( 'NONE',  ( 107.5000000000000284, -199.9999999999999716, 40.00000000000000000 ) ) ;
#14510=CARTESIAN_POINT ( 'NONE',  ( 96.48501399889538277, -114.8592206156971116, 49.50259502882540374 ) ) ;
#14512=CARTESIAN_POINT ( 'NONE',  ( 170.2125097089226529, -199.3942630591406839, 40.00000000000000000 ) ) ;
#14515=ADVANCED_FACE ( 'NONE', ( #436 ), #19160, .F. ) ;
#14519=ORIENTED_EDGE ( 'NONE', *, *, #9915, .T. ) ;
#14520=CARTESIAN_POINT ( 'NONE',  ( 71.18887634719571622, -147.8252249328912740, 39.99999999999999289 ) ) ;
#14530=DIRECTION ( 'NONE',  ( 1.000000000000000000, 0.000000000000000000, 0.000000000000000000 ) ) ;
#14535=EDGE_LOOP ( 'NONE', ( #3579, #7328, #17144, #18316 ) ) ;
#14537=DIRECTION ( 'NONE',  ( 0.000000000000000000, 0.000000000000000000, 1.000000000000000000 ) ) ;
#14547=CARTESIAN_POINT ( 'NONE',  ( -139.9266654873503626, 54.05438215086714848, 31.54788804351212761 ) ) ;
#14553=CARTESIAN_POINT ( 'NONE',  ( -102.7654166546896732, -126.4532151214411755, 1.186365931940917440 ) ) ;
#14555=VECTOR ( 'NONE', #17734, 1000.000000000000000 ) ;
#14559=CYLINDRICAL_SURFACE ( 'NONE', #14133, 7.500000000000007105 ) ;
#14560=DIRECTION ( 'NONE',  ( -0.2225209339563185562, 0.9749279121818227312, 0.000000000000000000 ) ) ;
#14574=LINE ( 'NONE', #12730, #11087 ) ;
#14575=EDGE_LOOP ( 'NONE', ( #14093, #10007, #14185, #8718 ) ) ;
#14577=DIRECTION ( 'NONE',  ( 0.000000000000000000, 0.000000000000000000, 1.000000000000000000 ) ) ;
#14580=CARTESIAN_POINT ( 'NONE',  ( -50.37374754117255549, -141.2886604036510221, 49.99999999999999289 ) ) ;
#14591=DIRECTION ( 'NONE',  ( 0.000000000000000000, 0.000000000000000000, 1.000000000000000000 ) ) ;
#14598=EDGE_LOOP ( 'NONE', ( #8567, #4045, #18011, #16484 ) ) ;
#14599=AXIS2_PLACEMENT_3D ( 'NONE', #16779, #20242, #6253 ) ;
#14606=AXIS2_PLACEMENT_3D ( 'NONE', #2677, #10742, #18221 ) ;
#14608=CARTESIAN_POINT ( 'NONE',  ( 0.000000000000000000, 0.000000000000000000, 40.00000000000000000 ) ) ;
#14609=CARTESIAN_POINT ( 'NONE',  ( 90.67862352884074539, -119.4897427140443966, 46.86044588094818408 ) ) ;
#14615=LINE ( 'NONE', #19328, #19390 ) ;
#14620=VECTOR ( 'NONE', #6190, 1000.000000000000114 ) ;
#14622=DIRECTION ( 'NONE',  ( -0.000000000000000000, -1.000000000000000000, -0.000000000000000000 ) ) ;
#14632=CARTESIAN_POINT ( 'NONE',  ( -82.03124999999998579, -125.5821405433014064, 10.00000000000000178 ) ) ;
#14635=CIRCLE ( 'NONE', #13308, 7.500000000000007105 ) ;
#14640=EDGE_LOOP ( 'NONE', ( #16868, #9977, #11491, #10593 ) ) ;
#14648=CARTESIAN_POINT ( 'NONE',  ( -96.87131796860795419, -115.7364764686971625, 10.33971351605897304 ) ) ;
#14651=CIRCLE ( 'NONE', #18930, 15.91767397667354267 ) ;
#14654=DIRECTION ( 'NONE',  ( -0.000000000000000000, -0.000000000000000000, -1.000000000000000000 ) ) ;
#14657=DIRECTION ( 'NONE',  ( 1.000000000000000000, 0.000000000000000000, 0.000000000000000000 ) ) ;
#14659=CARTESIAN_POINT ( 'NONE',  ( -123.3088579006944769, -85.41493018853608987, 40.34572370108148931 ) ) ;
#14660=VERTEX_POINT ( 'NONE', #18121 ) ;
#14666=ORIENTED_EDGE ( 'NONE', *, *, #2753, .F. ) ;
#14670=CARTESIAN_POINT ( 'NONE',  ( -127.8482905096655315, -78.45565238711304801, -8.397827111051714866 ) ) ;
#14671=FACE_OUTER_BOUND ( 'NONE', #4717, .T. ) ;
#14675=AXIS2_PLACEMENT_3D ( 'NONE', #14302, #12953, #5202 ) ;
#14677=CARTESIAN_POINT ( 'NONE',  ( -125.5756761630928366, -82.07265954314213730, -1.047228856968852817 ) ) ;
#14679=CARTESIAN_POINT ( 'NONE',  ( 133.2712073787624547, -68.96827650412444655, 8.924580230359330457 ) ) ;
#14680=DIRECTION ( 'NONE',  ( 1.000000000000000000, 0.000000000000000000, 0.000000000000000000 ) ) ;
#14681=DIRECTION ( 'NONE',  ( -0.000000000000000000, -0.000000000000000000, 1.000000000000000000 ) ) ;
#14683=EDGE_CURVE ( 'NONE', #13051, #10874, #19462, .T. ) ;
#14697=VERTEX_POINT ( 'NONE', #13601 ) ;
#14705=ORIENTED_EDGE ( 'NONE', *, *, #12852, .T. ) ;
#14707=EDGE_LOOP ( 'NONE', ( #7380, #7074 ) ) ;
#14708=EDGE_LOOP ( 'NONE', ( #1377, #11263, #14445 ) ) ;
#14709=AXIS2_PLACEMENT_3D ( 'NONE', #1827, #15947, #291 ) ;
#14715=CARTESIAN_POINT ( 'NONE',  ( -98.63424005417270735, -113.0189783045208571, 49.90251308629520111 ) ) ;
#14725=ORIENTED_EDGE ( 'NONE', *, *, #5310, .T. ) ;
#14726=CYLINDRICAL_SURFACE ( 'NONE', #4326, 7.500000000000007105 ) ;
#14728=DIRECTION ( 'NONE',  ( -0.000000000000000000, -0.000000000000000000, -1.000000000000000000 ) ) ;
#14742=LINE ( 'NONE', #722, #14362 ) ;
#14746=CARTESIAN_POINT ( 'NONE',  ( 96.05623471150424564, -115.3294058443303669, 4.799833099651143797 ) ) ;
#14748=CARTESIAN_POINT ( 'NONE',  ( -97.93656923779387569, -133.3799209237830041, 7.071677858121607763 ) ) ;
#14749=EDGE_CURVE ( 'NONE', #3424, #7495, #10051, .T. ) ;
#14750=CARTESIAN_POINT ( 'NONE',  ( -83.21341172527399976, -124.8022162803316348, 2.974423032988927407 ) ) ;
#14753=DIRECTION ( 'NONE',  ( 0.000000000000000000, 0.000000000000000000, 1.000000000000000000 ) ) ;
#14759=ORIENTED_EDGE ( 'NONE', *, *, #15623, .T. ) ;
#14762=EDGE_LOOP ( 'NONE', ( #9332, #12215, #12283, #3839 ) ) ;
#14764=CARTESIAN_POINT ( 'NONE',  ( -130.7934332354521132, -73.44669674648567081, -5.542612327196102306 ) ) ;
#14766=CARTESIAN_POINT ( 'NONE',  ( -60.00000000000000000, -2.094888803305880013E-13, -100.0000000000000000 ) ) ;
#14770=CARTESIAN_POINT ( 'NONE',  ( 134.6257061167716813, -73.66332987389617415, 7.420084151274023654 ) ) ;
#14780=ADVANCED_FACE ( 'NONE', ( #9207, #13706, #18525, #1545, #4613, #16889, #10836, #12273 ), #1229, .T. ) ;
#14785=ORIENTED_EDGE ( 'NONE', *, *, #6031, .T. ) ;
#14787=DIRECTION ( 'NONE',  ( 1.000000000000000000, 0.000000000000000000, 0.000000000000000000 ) ) ;
#14809=EDGE_LOOP ( 'NONE', ( #11679, #19687, #11004, #16182, #10497 ) ) ;
#14811=AXIS2_PLACEMENT_3D ( 'NONE', #5945, #7768, #7562 ) ;
#14813=ORIENTED_EDGE ( 'NONE', *, *, #18242, .F. ) ;
#14823=DIRECTION ( 'NONE',  ( 0.000000000000000000, 0.000000000000000000, 1.000000000000000000 ) ) ;
#14829=ORIENTED_EDGE ( 'NONE', *, *, #11626, .F. ) ;
#14830=CARTESIAN_POINT ( 'NONE',  ( 156.4179374840099683, -52.02840013023883614, 39.99999999999999289 ) ) ;
#14833=ORIENTED_EDGE ( 'NONE', *, *, #3226, .T. ) ;
#14835=EDGE_CURVE ( 'NONE', #2991, #10778, #15166, .T. ) ;
#14837=AXIS2_PLACEMENT_3D ( 'NONE', #458, #11400, #10066 ) ;
#14839=CARTESIAN_POINT ( 'NONE',  ( 87.56486837567058501, -121.7886324248894141, -4.190568952157736504 ) ) ;
#14840=CARTESIAN_POINT ( 'NONE',  ( -95.87737486567888823, -116.0928213521003869, 9.446122864778402572 ) ) ;
#14842=CARTESIAN_POINT ( 'NONE',  ( -82.03124999999998579, -125.5821405433014064, 10.00000000000000178 ) ) ;
#14847=DIRECTION ( 'NONE',  ( 1.000000000000000000, 0.000000000000000000, 0.000000000000000000 ) ) ;
#14852=CARTESIAN_POINT ( 'NONE',  ( -144.1130761623740568, -69.50842595698578918, 30.00000000000000000 ) ) ;
#14858=CARTESIAN_POINT ( 'NONE',  ( -176.7850001792984926, -188.8278678429259685, 7.673622252739133565 ) ) ;
#14866=CARTESIAN_POINT ( 'NONE',  ( -71.18887634719365565, -147.8252249328922687, 39.99999999999999289 ) ) ;
#14869=EDGE_CURVE ( 'NONE', #18649, #2503, #5061, .T. ) ;
#14871=VECTOR ( 'NONE', #16364, 1000.000000000000000 ) ;
#14874=ORIENTED_EDGE ( 'NONE', *, *, #8592, .T. ) ;
#14876=VERTEX_POINT ( 'NONE', #309 ) ;
#14881=AXIS2_PLACEMENT_3D ( 'NONE', #15531, #18494, #13884 ) ;
#14891=CARTESIAN_POINT ( 'NONE',  ( -134.5351519296995662, -74.34771143809115301, 6.414883565331459536 ) ) ;
#14895=CIRCLE ( 'NONE', #2815, 9.999999999999992895 ) ;
#14897=AXIS2_PLACEMENT_3D ( 'NONE', #1917, #15626, #11008 ) ;
#14898=CYLINDRICAL_SURFACE ( 'NONE', #14940, 7.500000000000002665 ) ;
#14901=CIRCLE ( 'NONE', #3812, 32.50000000000000000 ) ;
#14902=DIRECTION ( 'NONE',  ( 1.224646799147353207E-16, 1.000000000000000000, -0.000000000000000000 ) ) ;
#14904=ORIENTED_EDGE ( 'NONE', *, *, #12257, .F. ) ;
#14906=ORIENTED_EDGE ( 'NONE', *, *, #12374, .T. ) ;
#14908=CARTESIAN_POINT ( 'NONE',  ( 128.2779226595531270, 102.2982297021113141, 49.99999999999999289 ) ) ;
#14910=B_SPLINE_CURVE_WITH_KNOTS ( 'NONE', 3,
 ( #7518, #2721, #1172, #1594, #15400, #7418, #10791, #1386, #2825, #4561, #10682, #10477, #13653, #17147, #17046, #12220, #16939, #3031, #13755, #56, #20204, #15506, #16732, #1492, #6209, #13960, #18688, #12426, #19900, #7824 ),
 .UNSPECIFIED., .F., .F.,
 ( 4, 2, 2, 2, 2, 2, 2, 2, 2, 2, 2, 2, 2, 2, 4 ),
 ( 2.251336500357276218E-07, 0.003672487653379172701, 0.007344750173108309521, 0.009180881432972864270, 0.01101701269283741902, 0.01468927521256654586, 0.02203380025202480302, 0.02386993151188936471, 0.02570606277175392293, 0.02937832529148303590, 0.03672285033094124795, 0.04406737537039945307, 0.04773963789012858339, 0.05141190040985771370, 0.05875642544931597433 ),
 .UNSPECIFIED. ) ;
#14911=CARTESIAN_POINT ( 'NONE',  ( -96.48429163929540664, -114.8598460512868940, 49.50248771032619288 ) ) ;
#14912=FACE_OUTER_BOUND ( 'NONE', #6345, .T. ) ;
#14915=CARTESIAN_POINT ( 'NONE',  ( -123.6373235125731753, -84.94667440144655757, 50.00000000000000000 ) ) ;
#14918=DIRECTION ( 'NONE',  ( 0.000000000000000000, 0.000000000000000000, -1.000000000000000000 ) ) ;
#14925=ORIENTED_EDGE ( 'NONE', *, *, #6394, .F. ) ;
#14926=LINE ( 'NONE', #14830, #15969 ) ;
#14928=ORIENTED_EDGE ( 'NONE', *, *, #1795, .F. ) ;
#14930=AXIS2_PLACEMENT_3D ( 'NONE', #519, #616, #6860 ) ;
#14934=CARTESIAN_POINT ( 'NONE',  ( 106.3851141486848064, -120.5004170265810330, 0.04616215448129540322 ) ) ;
#14935=CARTESIAN_POINT ( 'NONE',  ( -105.2683707665257629, -122.4156632037601611, 0.2357454945587965922 ) ) ;
#14940=AXIS2_PLACEMENT_3D ( 'NONE', #881, #10290, #12119 ) ;
#14942=AXIS2_PLACEMENT_3D ( 'NONE', #8333, #3640, #11307 ) ;
#14956=CARTESIAN_POINT ( 'NONE',  ( -152.4599531637108498, -36.50981547337168109, 39.99999999999999289 ) ) ;
#14958=CARTESIAN_POINT ( 'NONE',  ( 134.6804726163186956, -73.23883837743916558, 8.316693297614211389 ) ) ;
#14959=CARTESIAN_POINT ( 'NONE',  ( 97.50000000000002842, -189.9999999999999716, 10.00000000000000178 ) ) ;
#14960=DIRECTION ( 'NONE',  ( -0.3427509529624101492, 0.9394263059140720573, 0.000000000000000000 ) ) ;
#14964=CARTESIAN_POINT ( 'NONE',  ( -126.6692879288293341, -80.35371549668381874, -9.119744649247303769 ) ) ;
#14965=CARTESIAN_POINT ( 'NONE',  ( 135.1060089016586119, -65.16414933584998437, 8.475570270055174049 ) ) ;
#14967=FACE_OUTER_BOUND ( 'NONE', #6359, .T. ) ;
#14972=EDGE_CURVE ( 'NONE', #12460, #4464, #1846, .T. ) ;
#14974=AXIS2_PLACEMENT_3D ( 'NONE', #14378, #9767, #6709 ) ;
#14976=ORIENTED_EDGE ( 'NONE', *, *, #5553, .F. ) ;
#14979=EDGE_CURVE ( 'NONE', #2173, #7363, #7015, .T. ) ;
#14987=DIRECTION ( 'NONE',  ( 0.000000000000000000, 0.000000000000000000, -1.000000000000000000 ) ) ;
#14994=CYLINDRICAL_SURFACE ( 'NONE', #9764, 15.91767397667355510 ) ;
#14995=CARTESIAN_POINT ( 'NONE',  ( -85.53020504959707182, -140.9188050298390067, 39.99999999999999289 ) ) ;
#15000=AXIS2_PLACEMENT_3D ( 'NONE', #9571, #58, #20104 ) ;
#15001=CIRCLE ( 'NONE', #12726, 39.99999999999997868 ) ;
#15005=EDGE_LOOP ( 'NONE', ( #18067, #8179, #19095, #3270 ) ) ;
#15007=ORIENTED_EDGE ( 'NONE', *, *, #19996, .T. ) ;
#15009=EDGE_CURVE ( 'NONE', #11373, #2503, #12556, .T. ) ;
#15014=CARTESIAN_POINT ( 'NONE',  ( -82.03124999999998579, -125.5821405433014064, 30.00000000000000000 ) ) ;
#15017=AXIS2_PLACEMENT_3D ( 'NONE', #14766, #19870, #5767 ) ;
#15018=EDGE_LOOP ( 'NONE', ( #3299, #19265, #14341, #18258 ) ) ;
#15019=CARTESIAN_POINT ( 'NONE',  ( -124.4476442249722226, -83.75451619235309408, 49.87919367093176959 ) ) ;
#15026=CARTESIAN_POINT ( 'NONE',  ( -132.6218665116185491, -85.29503539049817107, 39.26870858449429846 ) ) ;
#15033=VECTOR ( 'NONE', #19948, 1000.000000000000000 ) ;
#15035=CARTESIAN_POINT ( 'NONE',  ( -97.47038759843736955, -115.4903015188566826, 29.84619916992285837 ) ) ;
#15038=ORIENTED_EDGE ( 'NONE', *, *, #9102, .T. ) ;
#15042=CARTESIAN_POINT ( 'NONE',  ( 91.89277925368698163, -118.5585056022113832, -7.620840104674680759 ) ) ;
#15046=CARTESIAN_POINT ( 'NONE',  ( 120.7779226595531128, 102.2982297021113141, 39.99999999999999289 ) ) ;
#15048=DIRECTION ( 'NONE',  ( 0.7406645559057084549, -0.6718749999999998890, -9.546468602532142825E-17 ) ) ;
#15051=CYLINDRICAL_SURFACE ( 'NONE', #10858, 9.999999999999994671 ) ;
#15054=CARTESIAN_POINT ( 'NONE',  ( 159.9599531637113330, -36.50981547336952104, 39.99999999999999289 ) ) ;
#15061=CARTESIAN_POINT ( 'NONE',  ( 133.6865796038707117, -79.84358686291109564, 2.536759214717485111 ) ) ;
#15062=CARTESIAN_POINT ( 'NONE',  ( -32.50000000000000000, 0.000000000000000000, 49.99999999999999289 ) ) ;
#15064=CARTESIAN_POINT ( 'NONE',  ( -105.2664779077412192, -122.4188771607292949, 39.76387409687995245 ) ) ;
#15067=DIRECTION ( 'NONE',  ( -0.000000000000000000, -0.000000000000000000, -1.000000000000000000 ) ) ;
#15068=CARTESIAN_POINT ( 'NONE',  ( -132.9648440817100266, -83.65857578542973272, 1.155905617014955755 ) ) ;
#15069=CARTESIAN_POINT ( 'NONE',  ( 132.7722305162506302, -69.92010858955958952, 5.898643563562469438 ) ) ;
#15070=DIRECTION ( 'NONE',  ( -0.000000000000000000, -0.000000000000000000, -1.000000000000000000 ) ) ;
#15072=CARTESIAN_POINT ( 'NONE',  ( -134.7747342791601000, -65.84665809079258736, 34.80178653497117125 ) ) ;
#15076=ORIENTED_EDGE ( 'NONE', *, *, #8528, .F. ) ;
#15079=EDGE_CURVE ( 'NONE', #6085, #17491, #5697, .T. ) ;
#15093=CARTESIAN_POINT ( 'NONE',  ( 133.0662791979978863, -83.15705346520361729, 38.69754810580496951 ) ) ;
#15100=ORIENTED_EDGE ( 'NONE', *, *, #11279, .F. ) ;
#15103=ORIENTED_EDGE ( 'NONE', *, *, #12825, .F. ) ;
#15106=EDGE_CURVE ( 'NONE', #870, #14697, #2450, .T. ) ;
#15108=CYLINDRICAL_SURFACE ( 'NONE', #11234, 10.00000000000000000 ) ;
#15110=LINE ( 'NONE', #1091, #823 ) ;
#15113=CARTESIAN_POINT ( 'NONE',  ( -128.2293354902420504, -77.84035270136639895, 48.15785137238516711 ) ) ;
#15115=CIRCLE ( 'NONE', #1399, 9.999999999999994671 ) ;
#15122=VECTOR ( 'NONE', #6425, 1000.000000000000000 ) ;
#15123=LINE ( 'NONE', #2960, #4250 ) ;
#15126=ADVANCED_FACE ( 'NONE', ( #13575 ), #7345, .F. ) ;
#15128=DIRECTION ( 'NONE',  ( -0.000000000000000000, -1.000000000000000000, -0.000000000000000000 ) ) ;
#15135=EDGE_CURVE ( 'NONE', #12020, #9612, #5819, .T. ) ;
#15138=CIRCLE ( 'NONE', #18423, 77.50000000000000000 ) ;
#15140=CARTESIAN_POINT ( 'NONE',  ( -110.0000000000000142, 265.0000000000000000, -82.50000000000001421 ) ) ;
#15141=CARTESIAN_POINT ( 'NONE',  ( -136.4994460260982407, -31.11111111111750915, -10.83150941965273262 ) ) ;
#15149=EDGE_CURVE ( 'NONE', #17276, #17652, #19117, .T. ) ;
#15151=CARTESIAN_POINT ( 'NONE',  ( 181.0783081749256951, -199.9999999999999716, 40.00000000000000000 ) ) ;
#15158=ADVANCED_FACE ( 'NONE', ( #2958 ), #3062, .T. ) ;
#15159=ORIENTED_EDGE ( 'NONE', *, *, #4093, .F. ) ;
#15160=DIRECTION ( 'NONE',  ( 0.2225209339563044841, 0.9749279121818258398, 0.000000000000000000 ) ) ;
#15162=CARTESIAN_POINT ( 'NONE',  ( 132.1979689506645173, -87.16940599486623853, 0.3707483414095501528 ) ) ;
#15165=DIRECTION ( 'NONE',  ( 0.000000000000000000, 0.000000000000000000, -1.000000000000000000 ) ) ;
#15166=CIRCLE ( 'NONE', #4394, 150.0000000000000284 ) ;
#15169=CYLINDRICAL_SURFACE ( 'NONE', #19920, 7.500000000000003553 ) ;
#15170=CARTESIAN_POINT ( 'NONE',  ( -134.5985778548204905, -73.87143572891798726, 7.065257048864122424 ) ) ;
#15171=CARTESIAN_POINT ( 'NONE',  ( 132.2954651231882792, -86.73864221000000896, 0.4534272278281766266 ) ) ;
#15174=CARTESIAN_POINT ( 'NONE',  ( -134.6956030146838259, -73.12307453599522944, 31.50188018822290559 ) ) ;
#15183=CARTESIAN_POINT ( 'NONE',  ( -110.0000000000000142, 275.0000000000000000, 39.99999999999997868 ) ) ;
#15194=CARTESIAN_POINT ( 'NONE',  ( -189.9999999999988916, 275.0000000000000000, -2.499999999999734879 ) ) ;
#15199=CARTESIAN_POINT ( 'NONE',  ( -176.1792632384392050, -186.5724904703759535, 30.00000000000000000 ) ) ;
#15201=ORIENTED_EDGE ( 'NONE', *, *, #14749, .T. ) ;
#15207=FILL_AREA_STYLE_COLOUR ( '', #12529 ) ;
#15213=ORIENTED_EDGE ( 'NONE', *, *, #4883, .F. ) ;
#15214=FACE_BOUND ( 'NONE', #15395, .T. ) ;
#15220=CARTESIAN_POINT ( 'NONE',  ( -134.6804726163186388, -73.23883837743913716, 31.68330670238580282 ) ) ;
#15221=CARTESIAN_POINT ( 'NONE',  ( -90.70229574719763832, 106.6474785866378312, 34.20743887950242623 ) ) ;
#15227=AXIS2_PLACEMENT_3D ( 'NONE', #18001, #4070, #5612 ) ;
#15229=CARTESIAN_POINT ( 'NONE',  ( -98.53720805795876458, -132.5762351826747931, 34.43852096856275580 ) ) ;
#15231=EDGE_LOOP ( 'NONE', ( #12656, #3456, #18481, #18567 ) ) ;
#15236=VERTEX_POINT ( 'NONE', #12453 ) ;
#15237=CARTESIAN_POINT ( 'NONE',  ( 95.87485967515245022, -116.0949201519035370, 9.456033085400639138 ) ) ;
#15241=CARTESIAN_POINT ( 'NONE',  ( -136.1355222778962570, -24.69918106743299901, -20.28146826871829589 ) ) ;
#15247=ORIENTED_EDGE ( 'NONE', *, *, #8468, .T. ) ;
#15252=ORIENTED_EDGE ( 'NONE', *, *, #14869, .T. ) ;
#15253=ORIENTED_EDGE ( 'NONE', *, *, #5772, .F. ) ;
#15256=ORIENTED_EDGE ( 'NONE', *, *, #17111, .F. ) ;
#15258=DIRECTION ( 'NONE',  ( 0.000000000000000000, 0.000000000000000000, 1.000000000000000000 ) ) ;
#15259=CARTESIAN_POINT ( 'NONE',  ( 134.5748517645101572, -74.05062141148569310, 6.795614893174752424 ) ) ;
#15263=( BOUNDED_SURFACE ( )  B_SPLINE_SURFACE ( 3, 2, ( 
 ( #13933, #20178, #4847 ),
 ( #18761, #11069, #17224 ),
 ( #3205, #13100, #9839 ),
 ( #6688, #6880, #12908 ),
 ( #13290, #19458, #10047 ),
 ( #19358, #11475, #14748 ),
 ( #13006, #14648, #19161 ),
 ( #2183, #11576, #437 ),
 ( #19268, #17828, #16092 ),
 ( #8306, #17729, #8408 ),
 ( #3706, #8605, #17636 ),
 ( #3800, #6974, #13193 ),
 ( #2081, #14840, #19548 ),
 ( #16392, #729, #11762 ),
 ( #18024, #9945, #10140 ),
 ( #3993, #5441, #5249 ),
 ( #6784, #16195, #825 ),
 ( #3901, #637, #10234 ),
 ( #11668, #5346, #16296 ),
 ( #8508, #2280, #14553 ),
 ( #5155, #17929, #11380 ),
 ( #5541, #2371, #7076 ),
 ( #16490, #8206, #14452 ),
 ( #3607, #540, #13394 ),
 ( #16685, #5839, #14935 ),
 ( #13492, #12058, #10327 ),
 ( #2567, #5741, #2672 ),
 ( #11953, #2873, #11856 ) ),
 .UNSPECIFIED., .F., .F., .F. ) 
 B_SPLINE_SURFACE_WITH_KNOTS ( ( 4, 2, 2, 2, 2, 2, 2, 2, 2, 2, 2, 2, 2, 4 ),
 ( 3, 3 ),
 ( 0.01172725363905311943, 0.01619455768277540397, 0.01731138369370597424, 0.01842820970463654451, 0.02066186172649768504, 0.02289551374835882558, 0.02401233975928939585, 0.02512916577021996958, 0.02959646981394225412, 0.03406377385766454213, 0.03629742587952568267, 0.03853107790138682320, 0.04299838194510910427, 0.04746568598883138534 ),
 ( 0.000000000000000000, 1.000000000000000000 ),
 .UNSPECIFIED. ) 
 GEOMETRIC_REPRESENTATION_ITEM ( )  RATIONAL_B_SPLINE_SURFACE ( (
 ( 1.000000000000000000, 0.4759858191164941243, 1.000000000000000000),
 ( 1.000000000000000000, 0.4759956267211572500, 1.000000000000000000),
 ( 1.000000000000000000, 0.4778541562213696192, 1.000000000000000000),
 ( 1.000000000000000000, 0.4823973722701895839, 1.000000000000000000),
 ( 1.000000000000000000, 0.4834178931535008661, 1.000000000000000000),
 ( 1.000000000000000000, 0.4856852555523819004, 1.000000000000000000),
 ( 1.000000000000000000, 0.4869309269816905483, 1.000000000000000000),
 ( 1.000000000000000000, 0.4909487690765744761, 1.000000000000000000),
 ( 1.000000000000000000, 0.4940161083580011936, 1.000000000000000000),
 ( 1.000000000000000000, 0.5008835903390457256, 1.000000000000000000),
 ( 1.000000000000000000, 0.5046839780478528104, 1.000000000000000000),
 ( 1.000000000000000000, 0.5109205925582557262, 1.000000000000000000),
 ( 1.000000000000000000, 0.5130943221002354226, 1.000000000000000000),
 ( 1.000000000000000000, 0.5175691686948765691, 1.000000000000000000),
 ( 1.000000000000000000, 0.5198746620754810532, 1.000000000000000000),
 ( 1.000000000000000000, 0.5317265360209684211, 1.000000000000000000),
 ( 1.000000000000000000, 0.5422380167215470337, 1.000000000000000000),
 ( 1.000000000000000000, 0.5650731438342535551, 1.000000000000000000),
 ( 1.000000000000000000, 0.5770759225151705918, 1.000000000000000000),
 ( 1.000000000000000000, 0.5957780208533434152, 1.000000000000000000),
 ( 1.000000000000000000, 0.6021295156452242114, 1.000000000000000000),
 ( 1.000000000000000000, 0.6150481322456406996, 1.000000000000000000),
 ( 1.000000000000000000, 0.6215784740531448138, 1.000000000000000000),
 ( 1.000000000000000000, 0.6411710492557047836, 1.000000000000000000),
 ( 1.000000000000000000, 0.6543107498251993226, 1.000000000000000000),
 ( 1.000000000000000000, 0.6806663510245557491, 1.000000000000000000),
 ( 1.000000000000000000, 0.6938871677785066749, 1.000000000000000000),
 ( 1.000000000000000000, 0.7071067811865475727, 1.000000000000000000) ) ) 
 REPRESENTATION_ITEM ( '' )  SURFACE ( )  );
#15264=AXIS2_PLACEMENT_3D ( 'NONE', #17285, #15540, #12558 ) ;
#15265=CARTESIAN_POINT ( 'NONE',  ( 97.50000000000002842, -195.8578643762690206, 4.142135623730952787 ) ) ;
#15267=CARTESIAN_POINT ( 'NONE',  ( -100.7812499999999716, -111.0996833858562951, 50.00000000000000000 ) ) ;
#15271=CARTESIAN_POINT ( 'NONE',  ( -131.8415137303880726, -71.65490762083834397, 3.257559711240717526 ) ) ;
#15272=CARTESIAN_POINT ( 'NONE',  ( 131.4291603288649242, -72.40192386451009554, 2.550978253286948938 ) ) ;
#15273=CARTESIAN_POINT ( 'NONE',  ( 0.000000000000000000, 0.000000000000000000, 49.99999999999999289 ) ) ;
#15275=CARTESIAN_POINT ( 'NONE',  ( 107.5000000000000284, -199.9999999999999716, 40.00000000000000000 ) ) ;
#15276=ORIENTED_EDGE ( 'NONE', *, *, #1081, .T. ) ;
#15278=CARTESIAN_POINT ( 'NONE',  ( 0.000000000000000000, 0.000000000000000000, 0.000000000000000000 ) ) ;
#15290=PLANE ( 'NONE',  #10981 ) ;
#15291=DIRECTION ( 'NONE',  ( -0.000000000000000000, -0.000000000000000000, 1.000000000000000000 ) ) ;
#15292=CIRCLE ( 'NONE', #12355, 10.00000000000000178 ) ;
#15294=ORIENTED_EDGE ( 'NONE', *, *, #19486, .F. ) ;
#15298=CARTESIAN_POINT ( 'NONE',  ( -134.1103769904814840, -77.28650662340044164, 3.884190938604082266 ) ) ;
#15303=VERTEX_POINT ( 'NONE', #9500 ) ;
#15317=DIRECTION ( 'NONE',  ( 1.000000000000000000, 0.000000000000000000, 0.000000000000000000 ) ) ;
#15318=VECTOR ( 'NONE', #9953, 1000.000000000000000 ) ;
#15320=DIRECTION ( 'NONE',  ( -1.000000000000000000, 0.000000000000000000, -0.000000000000000000 ) ) ;
#15325=DIRECTION ( 'NONE',  ( -0.9009688679024160374, -0.4338837391175646707, 0.000000000000000000 ) ) ;
#15327=CARTESIAN_POINT ( 'NONE',  ( -95.40135526861702431, 102.4752410541829306, 36.83510734335156656 ) ) ;
#15332=ORIENTED_EDGE ( 'NONE', *, *, #1752, .F. ) ;
#15340=CARTESIAN_POINT ( 'NONE',  ( 96.05830942202625522, -116.0381168402492023, 9.733529271712557218 ) ) ;
#15343=CARTESIAN_POINT ( 'NONE',  ( -141.3095340546368277, -18.69392313914324788, -14.89730798426476888 ) ) ;
#15346=DIRECTION ( 'NONE',  ( 0.6234898018587442525, -0.7818314824680211439, 0.000000000000000000 ) ) ;
#15348=PLANE ( 'NONE',  #14606 ) ;
#15349=DIRECTION ( 'NONE',  ( 0.000000000000000000, 0.000000000000000000, 1.000000000000000000 ) ) ;
#15351=CARTESIAN_POINT ( 'NONE',  ( 96.25554516486297985, -115.9717118653463785, 30.02399084163740284 ) ) ;
#15354=FACE_OUTER_BOUND ( 'NONE', #8622, .T. ) ;
#15355=DIRECTION ( 'NONE',  ( 0.000000000000000000, 0.000000000000000000, 1.000000000000000000 ) ) ;
#15359=ORIENTED_EDGE ( 'NONE', *, *, #388, .F. ) ;
#15362=AXIS2_PLACEMENT_3D ( 'NONE', #10027, #16278, #5933 ) ;
#15364=ORIENTED_EDGE ( 'NONE', *, *, #3742, .F. ) ;
#15368=LINE ( 'NONE', #12292, #18877 ) ;
#15370=CARTESIAN_POINT ( 'NONE',  ( 101.6421356237309794, -200.0000000000000000, 4.186828437777334426E-15 ) ) ;
#15376=CARTESIAN_POINT ( 'NONE',  ( 130.0495322079418372, -74.74954793754227467, -6.424697538702346833 ) ) ;
#15377=CARTESIAN_POINT ( 'NONE',  ( -163.5019688434124419, -20.99123081650240863, 39.99999999999999289 ) ) ;
#15378=CYLINDRICAL_SURFACE ( 'NONE', #16063, 34.99999999999997868 ) ;
#15379=CARTESIAN_POINT ( 'NONE',  ( -131.2164711380630990, -72.78471332658050130, 37.79149633612817638 ) ) ;
#15384=AXIS2_PLACEMENT_3D ( 'NONE', #15273, #20082, #1262 ) ;
#15388=CIRCLE ( 'NONE', #18678, 160.0000000000000284 ) ;
#15390=CARTESIAN_POINT ( 'NONE',  ( -139.5534466488780936, -22.43207410479775277, 23.76218694605343984 ) ) ;
#15395=EDGE_LOOP ( 'NONE', ( #6017, #6280 ) ) ;
#15396=( GEOMETRIC_REPRESENTATION_CONTEXT ( 3 ) GLOBAL_UNCERTAINTY_ASSIGNED_CONTEXT ( ( #13763 ) ) GLOBAL_UNIT_ASSIGNED_CONTEXT ( ( #3711, #16305, #19365 ) ) REPRESENTATION_CONTEXT ( 'NONE', 'WORKASPACE' ) );
#15397=DIRECTION ( 'NONE',  ( 0.000000000000000000, 0.000000000000000000, 1.000000000000000000 ) ) ;
#15400=CARTESIAN_POINT ( 'NONE',  ( -81.18278579426254282, 113.5842013066641130, -14.89122930995394256 ) ) ;
#15405=EDGE_CURVE ( 'NONE', #6447, #19359, #1628, .T. ) ;
#15412=EDGE_LOOP ( 'NONE', ( #10798, #20109, #16078, #1164 ) ) ;
#15433=CARTESIAN_POINT ( 'NONE',  ( -134.7188131032333445, -72.93593548660989256, 30.00000000000000000 ) ) ;
#15434=CARTESIAN_POINT ( 'NONE',  ( -87.29829728531822752, 109.4572494691238518, 31.67964062618897003 ) ) ;
#15436=DIRECTION ( 'NONE',  ( 0.000000000000000000, 0.000000000000000000, 1.000000000000000000 ) ) ;
#15442=CARTESIAN_POINT ( 'NONE',  ( -97.70829847158753978, -133.6812691754211926, 32.03888873557544770 ) ) ;
#15449=CARTESIAN_POINT ( 'NONE',  ( 97.52076053070045702, -133.9271890290841611, 9.255816378659050159 ) ) ;
#15450=CARTESIAN_POINT ( 'NONE',  ( 15.91767397667355510, 149.1530343478547422, 39.99999999999999289 ) ) ;
#15453=EDGE_LOOP ( 'NONE', ( #4706, #532, #9303, #16821, #3560, #12536, #483, #15514 ) ) ;
#15457=CARTESIAN_POINT ( 'NONE',  ( 90.39157087502310617, -119.7120742831054372, 46.69505570264369254 ) ) ;
#15467=AXIS2_PLACEMENT_3D ( 'NONE', #7410, #4041, #8841 ) ;
#15469=LINE ( 'NONE', #12803, #8480 ) ;
#15476=ADVANCED_FACE ( 'NONE', ( #8257 ), #18248, .F. ) ;
#15477=CARTESIAN_POINT ( 'NONE',  ( -96.59911734864401467, -114.8254675080908953, 36.23371386736513244 ) ) ;
#15478=CARTESIAN_POINT ( 'NONE',  ( 71.18887634719571622, -147.8252249328912740, 39.99999999999999289 ) ) ;
#15481=CARTESIAN_POINT ( 'NONE',  ( -189.9999999999988916, 275.0000000000000000, 5.000000000000268230 ) ) ;
#15482=CARTESIAN_POINT ( 'NONE',  ( -133.2712073792708907, -68.96827650320689429, 9.471058287156711941 ) ) ;
#15483=CARTESIAN_POINT ( 'NONE',  ( 127.0298602564891013, -79.77387071031716914, -8.901236177966797669 ) ) ;
#15487=CARTESIAN_POINT ( 'NONE',  ( -125.8775035253894146, -81.60755858752349923, 41.03713929422894324 ) ) ;
#15488=ORIENTED_EDGE ( 'NONE', *, *, #4016, .T. ) ;
#15496=CARTESIAN_POINT ( 'NONE',  ( -141.9821482856067689, -18.16655044785428075, -9.224423568343562252 ) ) ;
#15503=CARTESIAN_POINT ( 'NONE',  ( -137.6581377289620320, -21.36537278083219604, -16.45265777907983917 ) ) ;
#15506=CARTESIAN_POINT ( 'NONE',  ( -99.15300337306508993, 89.83204135164545789, -28.30778954837869676 ) ) ;
#15508=CARTESIAN_POINT ( 'NONE',  ( 97.50000000000002842, -189.9999999999999716, 10.00000000000000178 ) ) ;
#15513=CARTESIAN_POINT ( 'NONE',  ( -170.2125097089225960, -199.3942630591408260, 40.00000000000000000 ) ) ;
#15514=ORIENTED_EDGE ( 'NONE', *, *, #3226, .F. ) ;
#15516=ADVANCED_FACE ( 'NONE', ( #19778 ), #1129, .F. ) ;
#15517=ORIENTED_EDGE ( 'NONE', *, *, #1642, .T. ) ;
#15521=ORIENTED_EDGE ( 'NONE', *, *, #12135, .F. ) ;
#15525=DIRECTION ( 'NONE',  ( 0.9394263059140719463, 0.3427509529624103712, 0.000000000000000000 ) ) ;
#15526=DIRECTION ( 'NONE',  ( -1.613511099790691498E-16, 1.000000000000000000, 0.000000000000000000 ) ) ;
#15528=EDGE_CURVE ( 'NONE', #9322, #2029, #12517, .T. ) ;
#15529=AXIS2_PLACEMENT_3D ( 'NONE', #18978, #3419, #4962 ) ;
#15531=CARTESIAN_POINT ( 'NONE',  ( -87.49999999999998579, -133.9542832461881687, 10.00000000000000000 ) ) ;
#15534=EDGE_CURVE ( 'NONE', #3447, #13254, #1157, .T. ) ;
#15536=ADVANCED_FACE ( 'NONE', ( #7501 ), #18817, .F. ) ;
#15540=DIRECTION ( 'NONE',  ( -0.3427509529624101492, 0.9394263059140721683, 0.000000000000000000 ) ) ;
#15543=CARTESIAN_POINT ( 'NONE',  ( -75.26415512511634631, 118.0479206960037288, 9.312873650067192699 ) ) ;
#15550=CARTESIAN_POINT ( 'NONE',  ( -147.0809924354783220, 29.44794838685322702, -9.999999999999978684 ) ) ;
#15552=ORIENTED_EDGE ( 'NONE', *, *, #8275, .F. ) ;
#15554=CARTESIAN_POINT ( 'NONE',  ( 97.70829847158759662, -133.6812691754159630, 7.961111264424513223 ) ) ;
#15555=FACE_OUTER_BOUND ( 'NONE', #12207, .T. ) ;
#15558=CARTESIAN_POINT ( 'NONE',  ( 7.500000000000420997, -60.00000000000000000, -105.0000000000000142 ) ) ;
#15560=ORIENTED_EDGE ( 'NONE', *, *, #5237, .F. ) ;
#15561=LINE ( 'NONE', #4719, #410 ) ;
#15564=CARTESIAN_POINT ( 'NONE',  ( 99.98138848894193131, -130.5820681961301375, 36.62898419040125475 ) ) ;
#15565=CIRCLE ( 'NONE', #18171, 150.0000000000000284 ) ;
#15567=CIRCLE ( 'NONE', #14897, 34.99999999999997868 ) ;
#15569=CARTESIAN_POINT ( 'NONE',  ( 50.37374754117453080, -141.2886604036503115, 49.99999999999999289 ) ) ;
#15582=CARTESIAN_POINT ( 'NONE',  ( -95.87485967515243601, -116.0949201519087666, 30.54396691460070556 ) ) ;
#15584=PLANE ( 'NONE',  #293 ) ;
#15588=CIRCLE ( 'NONE', #9375, 7.500000000000002665 ) ;
#15592=CARTESIAN_POINT ( 'NONE',  ( -128.7754324793921228, -76.93177152330437707, 47.71976547401850866 ) ) ;
#15594=DIRECTION ( 'NONE',  ( 0.9749279121818257288, -0.2225209339563047062, 0.000000000000000000 ) ) ;
#15609=DIRECTION ( 'NONE',  ( 0.000000000000000000, 0.000000000000000000, 1.000000000000000000 ) ) ;
#15621=ADVANCED_FACE ( 'NONE', ( #17446, #17643 ), #19078, .T. ) ;
#15623=EDGE_CURVE ( 'NONE', #5786, #5586, #11912, .T. ) ;
#15624=DIRECTION ( 'NONE',  ( 0.000000000000000000, 0.000000000000000000, -1.000000000000000000 ) ) ;
#15626=DIRECTION ( 'NONE',  ( 0.000000000000000000, 1.000000000000000000, 0.000000000000000000 ) ) ;
#15628=CARTESIAN_POINT ( 'NONE',  ( -97.53506906366366991, -133.9085396777615244, 30.96104885487609337 ) ) ;
#15631=CARTESIAN_POINT ( 'NONE',  ( -109.9999999999983515, 275.0000000000000000, 85.00000000000001421 ) ) ;
#15636=ADVANCED_FACE ( 'NONE', ( #5064 ), #9649, .T. ) ;
#15639=CARTESIAN_POINT ( 'NONE',  ( -79.24532193214523090, 125.6874967381585435, -20.60241429600958085 ) ) ;
#15645=CARTESIAN_POINT ( 'NONE',  ( -104.5696057486236441, 93.10197836950014505, 39.59507579059730631 ) ) ;
#15646=VECTOR ( 'NONE', #752, 1000.000000000000000 ) ;
#15648=VERTEX_POINT ( 'NONE', #6594 ) ;
#15653=EDGE_CURVE ( 'NONE', #4680, #13974, #5258, .T. ) ;
#15656=LINE ( 'NONE', #17192, #16312 ) ;
#15658=CARTESIAN_POINT ( 'NONE',  ( -117.9669857229114314, 78.77317465270277808, -34.20188040274583585 ) ) ;
#15659=FACE_OUTER_BOUND ( 'NONE', #2791, .T. ) ;
#15661=CARTESIAN_POINT ( 'NONE',  ( 85.13411715130894208, -123.5004392096819146, -1.042466200307516466 ) ) ;
#15667=ORIENTED_EDGE ( 'NONE', *, *, #3690, .F. ) ;
#15671=CARTESIAN_POINT ( 'NONE',  ( 96.12039245754215244, -116.0188909747135853, 30.17258640897478372 ) ) ;
#15674=CARTESIAN_POINT ( 'NONE',  ( -87.64225943403401686, 121.7426507922284600, 38.20596441781194130 ) ) ;
#15677=EDGE_LOOP ( 'NONE', ( #7937, #5334, #3466, #18887, #2191 ) ) ;
#15680=ORIENTED_EDGE ( 'NONE', *, *, #9915, .F. ) ;
#15685=CARTESIAN_POINT ( 'NONE',  ( -97.50000000000000000, -133.9542832461881972, 9.514131777208458374 ) ) ;
#15687=ORIENTED_EDGE ( 'NONE', *, *, #4482, .T. ) ;
#15692=CARTESIAN_POINT ( 'NONE',  ( -103.0319911124590533, -126.0382377111977377, 38.95151328076024555 ) ) ;
#15693=CARTESIAN_POINT ( 'NONE',  ( -156.4179374840092862, -52.02840013024096066, 39.99999999999999289 ) ) ;
#15695=CYLINDRICAL_SURFACE ( 'NONE', #9867, 7.500000000000007105 ) ;
#15698=CARTESIAN_POINT ( 'NONE',  ( -133.8370531740368108, -67.73246766859803358, 39.14630742583677403 ) ) ;
#15706=EDGE_LOOP ( 'NONE', ( #12744, #5738, #19468, #6011 ) ) ;
#15707=CARTESIAN_POINT ( 'NONE',  ( -144.4627684701566466, -14.76432773141799260, -1.188257704013451654 ) ) ;
#15717=CARTESIAN_POINT ( 'NONE',  ( -7.500000000000006217, 164.0736214083062805, 39.99999999999999289 ) ) ;
#15721=VERTEX_POINT ( 'NONE', #8903 ) ;
#15730=CARTESIAN_POINT ( 'NONE',  ( -189.9999999999988916, 265.0000000000000000, -2.499999999999734879 ) ) ;
#15734=EDGE_LOOP ( 'NONE', ( #9830, #4974 ) ) ;
#15741=CYLINDRICAL_SURFACE ( 'NONE', #15264, 9.999999999999998224 ) ;
#15743=CARTESIAN_POINT ( 'NONE',  ( -75.81749350294444412, 117.6933339947108976, -2.532388154262697810 ) ) ;
#15745=ORIENTED_EDGE ( 'NONE', *, *, #242, .F. ) ;
#15749=ADVANCED_FACE ( 'NONE', ( #7372 ), #15051, .T. ) ;
#15758=AXIS2_PLACEMENT_3D ( 'NONE', #18355, #20191, #17029 ) ;
#15771=CARTESIAN_POINT ( 'NONE',  ( -93.64123074234042576, 117.1838922457435217, 41.50921557003555051 ) ) ;
#15773=VERTEX_POINT ( 'NONE', #933 ) ;
#15781=ORIENTED_EDGE ( 'NONE', *, *, #3649, .T. ) ;
#15785=DIRECTION ( 'NONE',  ( 0.000000000000000000, 0.000000000000000000, 1.000000000000000000 ) ) ;
#15786=CARTESIAN_POINT ( 'NONE',  ( -96.12355554546984138, -116.0165654454242485, 30.18179740741101114 ) ) ;
#15788=DIRECTION ( 'NONE',  ( 1.000000000000000000, 0.000000000000000000, 0.000000000000000000 ) ) ;
#15791=CARTESIAN_POINT ( 'NONE',  ( -92.21618480002783258, -118.3073397699786540, -7.802271786604253023 ) ) ;
#15792=CARTESIAN_POINT ( 'NONE',  ( 107.5000000000000142, -118.5063289449133492, 0.000000000000000000 ) ) ;
#15799=CARTESIAN_POINT ( 'NONE',  ( -130.9519479124771237, -73.15688856708418086, 45.28395117799519909 ) ) ;
#15810=CIRCLE ( 'NONE', #15467, 40.00000000000000711 ) ;
#15814=CARTESIAN_POINT ( 'NONE',  ( 128.2779226595531270, 102.2982297021113141, 49.99999999999999289 ) ) ;
#15817=CARTESIAN_POINT ( 'NONE',  ( 97.77474281578807336, -133.5937942518637556, 32.33949703673819442 ) ) ;
#15818=DIRECTION ( 'NONE',  ( -1.000000000000000000, 0.000000000000000000, 0.000000000000000000 ) ) ;
#15822=CARTESIAN_POINT ( 'NONE',  ( 135.1060089022256818, -65.16414933467420667, 30.00000000000000000 ) ) ;
#15823=CARTESIAN_POINT ( 'NONE',  ( 133.9050245804181998, -78.55577302928909944, 36.83190385597256977 ) ) ;
#15833=CARTESIAN_POINT ( 'NONE',  ( -97.63639055817483836, -133.7757280588254218, 31.66285136016151114 ) ) ;
#15837=CARTESIAN_POINT ( 'NONE',  ( 0.000000000000000000, 0.000000000000000000, 49.99999999999999289 ) ) ;
#15838=CARTESIAN_POINT ( 'NONE',  ( 0.000000000000000000, 0.000000000000000000, -40.00000000000000000 ) ) ;
#15839=ORIENTED_EDGE ( 'NONE', *, *, #4482, .F. ) ;
#15844=ADVANCED_FACE ( 'NONE', ( #11052 ), #20231, .F. ) ;
#15846=DIRECTION ( 'NONE',  ( 0.000000000000000000, 0.000000000000000000, 1.000000000000000000 ) ) ;
#15848=FACE_OUTER_BOUND ( 'NONE', #1277, .T. ) ;
#15851=ORIENTED_EDGE ( 'NONE', *, *, #19711, .F. ) ;
#15852=CIRCLE ( 'NONE', #12613, 10.00000000000000888 ) ;
#15855=EDGE_CURVE ( 'NONE', #8838, #14482, #11560, .T. ) ;
#15858=CARTESIAN_POINT ( 'NONE',  ( -143.0849254817002816, 42.75236248750393031, -17.56505644796369126 ) ) ;
#15863=DIRECTION ( 'NONE',  ( -1.000000000000000000, 0.000000000000000000, 0.000000000000000000 ) ) ;
#15868=DIRECTION ( 'NONE',  ( 0.000000000000000000, 0.000000000000000000, 1.000000000000000000 ) ) ;
#15869=ORIENTED_EDGE ( 'NONE', *, *, #3649, .F. ) ;
#15875=ORIENTED_EDGE ( 'NONE', *, *, #13472, .F. ) ;
#15876=CARTESIAN_POINT ( 'NONE',  ( 42.50000000000000000, 0.000000000000000000, -49.99999999999999289 ) ) ;
#15878=VERTEX_POINT ( 'NONE', #11361 ) ;
#15880=ORIENTED_EDGE ( 'NONE', *, *, #9145, .T. ) ;
#15881=VERTEX_POINT ( 'NONE', #14632 ) ;
#15883=AXIS2_PLACEMENT_3D ( 'NONE', #2444, #13263, #8674 ) ;
#15886=CARTESIAN_POINT ( 'NONE',  ( 0.000000000000000000, 0.000000000000000000, -39.99999999999999289 ) ) ;
#15887=CARTESIAN_POINT ( 'NONE',  ( -150.0000000000000000, 0.000000000000000000, 5.000000000000011546 ) ) ;
#15890=CARTESIAN_POINT ( 'NONE',  ( 126.7590367374603346, -80.21250349114239953, 49.07649135601570123 ) ) ;
#15892=CARTESIAN_POINT ( 'NONE',  ( -100.2452644940503177, -111.5858889953167790, -10.00000000000000000 ) ) ;
#15895=CARTESIAN_POINT ( 'NONE',  ( -147.0809924354783220, 29.44794838685322702, -9.999999999999978684 ) ) ;
#15898=DIRECTION ( 'NONE',  ( -0.000000000000000000, -0.000000000000000000, 1.000000000000000000 ) ) ;
#15900=CARTESIAN_POINT ( 'NONE',  ( -111.9190551610216744, 70.74871087183512941, -30.00000000000067146 ) ) ;
#15904=EDGE_LOOP ( 'NONE', ( #8369, #424 ) ) ;
#15918=CARTESIAN_POINT ( 'NONE',  ( 105.6220017318342599, -121.8343408522480757, 39.87492654200375597 ) ) ;
#15921=CARTESIAN_POINT ( 'NONE',  ( 134.3599121685105331, -75.61163470463371539, 34.89991303621640384 ) ) ;
#15926=ORIENTED_EDGE ( 'NONE', *, *, #17307, .F. ) ;
#15933=CARTESIAN_POINT ( 'NONE',  ( -98.17567701213376097, -133.0624052623789453, 33.63793053978134395 ) ) ;
#15935=DIRECTION ( 'NONE',  ( 0.000000000000000000, 0.000000000000000000, -1.000000000000000000 ) ) ;
#15936=ORIENTED_EDGE ( 'NONE', *, *, #11927, .F. ) ;
#15937=CARTESIAN_POINT ( 'NONE',  ( 126.0117988550009898, -81.37275256441674287, -9.384899655049048661 ) ) ;
#15940=AXIS2_PLACEMENT_3D ( 'NONE', #8059, #11025, #3265 ) ;
#15947=DIRECTION ( 'NONE',  ( -0.000000000000000000, -0.000000000000000000, -1.000000000000000000 ) ) ;
#15948=CARTESIAN_POINT ( 'NONE',  ( 82.03125000000002842, -125.5821405433014064, 31.45421909404266003 ) ) ;
#15964=VECTOR ( 'NONE', #14322, 1000.000000000000000 ) ;
#15969=VECTOR ( 'NONE', #7065, 1000.000000000000114 ) ;
#15970=EDGE_LOOP ( 'NONE', ( #973, #10902, #19410, #11186 ) ) ;
#15977=CARTESIAN_POINT ( 'NONE',  ( -105.5833827013284179, 106.5503530635426728, 44.76066109344641575 ) ) ;
#15986=VECTOR ( 'NONE', #8750, 1000.000000000000000 ) ;
#15990=FACE_OUTER_BOUND ( 'NONE', #11951, .T. ) ;
#15991=ADVANCED_FACE ( 'NONE', ( #18305 ), #3978, .F. ) ;
#15993=CARTESIAN_POINT ( 'NONE',  ( -131.0756278511784387, 49.33196612817722126, 32.98962906955656393 ) ) ;
#15996=CARTESIAN_POINT ( 'NONE',  ( -149.8786630148831307, 6.156332247747114295, 1.822476016178801173 ) ) ;
#15999=DIRECTION ( 'NONE',  ( -0.000000000000000000, -0.000000000000000000, 1.000000000000000000 ) ) ;
#16005=FACE_OUTER_BOUND ( 'NONE', #505, .T. ) ;
#16009=ORIENTED_EDGE ( 'NONE', *, *, #6362, .T. ) ;
#16010=AXIS2_PLACEMENT_3D ( 'NONE', #14520, #17895, #19037 ) ;
#16015=CIRCLE ( 'NONE', #5001, 110.0000000000000142 ) ;
#16016=CARTESIAN_POINT ( 'NONE',  ( -136.2050403295488081, -31.16119972761966750, -14.14170230107002268 ) ) ;
#16017=VERTEX_POINT ( 'NONE', #13379 ) ;
#16019=DIRECTION ( 'NONE',  ( -0.000000000000000000, -0.000000000000000000, 1.000000000000000000 ) ) ;
#16022=CARTESIAN_POINT ( 'NONE',  ( 103.4088548222097046, -125.4447869035479073, 39.12902662653470287 ) ) ;
#16025=AXIS2_PLACEMENT_3D ( 'NONE', #5011, #17286, #14098 ) ;
#16027=AXIS2_PLACEMENT_3D ( 'NONE', #13524, #19773, #5769 ) ;
#16029=ORIENTED_EDGE ( 'NONE', *, *, #3159, .F. ) ;
#16035=DIRECTION ( 'NONE',  ( -1.000000000000000000, 0.000000000000000000, 0.000000000000000000 ) ) ;
#16050=CARTESIAN_POINT ( 'NONE',  ( 0.000000000000000000, 0.000000000000000000, -9.999999999999987566 ) ) ;
#16052=CARTESIAN_POINT ( 'NONE',  ( -75.01458320008653402, 118.2066678791461953, 6.325805891068640108 ) ) ;
#16058=ORIENTED_EDGE ( 'NONE', *, *, #438, .F. ) ;
#16063=AXIS2_PLACEMENT_3D ( 'NONE', #1263, #10872, #10561 ) ;
#16070=DIRECTION ( 'NONE',  ( -0.000000000000000000, -0.000000000000000000, -1.000000000000000000 ) ) ;
#16071=DIRECTION ( 'NONE',  ( -1.000000000000000000, 0.000000000000000000, 0.000000000000000000 ) ) ;
#16072=CARTESIAN_POINT ( 'NONE',  ( 50.37374754117451658, -141.2886604036502831, 49.99999999999999289 ) ) ;
#16074=DIRECTION ( 'NONE',  ( 0.000000000000000000, 0.000000000000000000, 1.000000000000000000 ) ) ;
#16076=DIRECTION ( 'NONE',  ( 0.000000000000000000, 0.000000000000000000, 1.000000000000000000 ) ) ;
#16078=ORIENTED_EDGE ( 'NONE', *, *, #7854, .T. ) ;
#16085=ORIENTED_EDGE ( 'NONE', *, *, #13127, .T. ) ;
#16087=CARTESIAN_POINT ( 'NONE',  ( -149.2033348278766027, 15.60004678097522657, 13.02734773726837147 ) ) ;
#16091=DIRECTION ( 'NONE',  ( -0.9394263059140720573, -0.3427509529624101492, 0.000000000000000000 ) ) ;
#16092=CARTESIAN_POINT ( 'NONE',  ( -98.30983243222962642, -132.8827373471657722, 6.041609267868833122 ) ) ;
#16093=ORIENTED_EDGE ( 'NONE', *, *, #3781, .F. ) ;
#16094=PLANE ( 'NONE',  #14060 ) ;
#16098=DIRECTION ( 'NONE',  ( 1.000000000000000000, 0.000000000000000000, 0.000000000000000000 ) ) ;
#16099=CARTESIAN_POINT ( 'NONE',  ( -130.9868171408399746, -91.88282611735537841, 40.00000000000000000 ) ) ;
#16100=ADVANCED_FACE ( 'NONE', ( #7654 ), #6241, .T. ) ;
#16102=CARTESIAN_POINT ( 'NONE',  ( -138.1593264817448414, 18.92187976101237368, -15.79357949266177386 ) ) ;
#16103=AXIS2_PLACEMENT_3D ( 'NONE', #15278, #17132, #6086 ) ;
#16104=EDGE_LOOP ( 'NONE', ( #15745, #9960 ) ) ;
#16106=ORIENTED_EDGE ( 'NONE', *, *, #899, .T. ) ;
#16109=EDGE_CURVE ( 'NONE', #12588, #3447, #4593, .T. ) ;
#16118=AXIS2_PLACEMENT_3D ( 'NONE', #3372, #11344, #16458 ) ;
#16120=DIRECTION ( 'NONE',  ( -0.000000000000000000, -1.000000000000000000, -0.000000000000000000 ) ) ;
#16122=VERTEX_POINT ( 'NONE', #90 ) ;
#16129=ORIENTED_EDGE ( 'NONE', *, *, #15079, .T. ) ;
#16132=EDGE_CURVE ( 'NONE', #4680, #5679, #6899, .T. ) ;
#16137=ORIENTED_EDGE ( 'NONE', *, *, #8520, .T. ) ;
#16139=DIRECTION ( 'NONE',  ( -1.613511099790691498E-16, 1.000000000000000000, 0.000000000000000000 ) ) ;
#16140=ORIENTED_EDGE ( 'NONE', *, *, #19033, .F. ) ;
#16141=CARTESIAN_POINT ( 'NONE',  ( 128.2779226595531270, 102.2982297021113141, 39.99999999999999289 ) ) ;
#16144=B_SPLINE_CURVE_WITH_KNOTS ( 'NONE', 3,
 ( #7487, #12187, #19567, #14958, #5560, #16704, #13725, #15259, #2689, #13515, #18137, #11781, #19866, #18043, #4217, #18341, #8821, #15061, #19766, #10446, #8918, #9124, #4315, #15162, #16604, #1144, #18235, #16511 ),
 .UNSPECIFIED., .F., .F.,
 ( 4, 2, 2, 2, 2, 2, 2, 2, 2, 2, 2, 2, 2, 4 ),
 ( 0.000000000000000000, 0.001466376146900906291, 0.002199564220351354991, 0.002932752293801805642, 0.004399128440702712584, 0.005865504587603619958, 0.007331880734504528201, 0.008798256881405435575, 0.01026463302830634382, 0.01173100917520725033, 0.01466376146900906334, 0.01759651376281088156, 0.02052926605661269457, 0.02346201835041451106 ),
 .UNSPECIFIED. ) ;
#16150=CARTESIAN_POINT ( 'NONE',  ( 95.41207185104578059, -115.7515782192335081, 49.20090002619129166 ) ) ;
#16151=ORIENTED_EDGE ( 'NONE', *, *, #3412, .F. ) ;
#16152=B_SPLINE_CURVE_WITH_KNOTS ( 'NONE', 3,
 ( #8223, #12927, #6804, #5176, #19185, #13027, #2300, #17844, #19570, #13213, #2098, #5561, #11494, #14764, #11783, #17745, #3821, #16212, #14670, #751, #657, #6902, #13115, #6996 ),
 .UNSPECIFIED., .F., .F.,
 ( 4, 2, 2, 2, 2, 2, 2, 2, 2, 2, 2, 4 ),
 ( 0.000000000000000000, 0.002185557465519409343, 0.004371114931038821289, 0.008742229862077633903, 0.01311334479311644652, 0.01529890225863585543, 0.01748445972415526087, 0.02185557465519410644, 0.02404113212071354658, 0.02622668958623298671, 0.03059780451727186351, 0.03496891944831072296 ),
 .UNSPECIFIED. ) ;
#16153=CARTESIAN_POINT ( 'NONE',  ( -110.0000000000000142, 1.347111479062088839E-14, -9.999999999999994671 ) ) ;
#16157=DIRECTION ( 'NONE',  ( 0.000000000000000000, 1.000000000000000000, 0.000000000000000000 ) ) ;
#16158=EDGE_LOOP ( 'NONE', ( #13693, #12129, #1299, #13858 ) ) ;
#16159=EDGE_CURVE ( 'NONE', #12285, #18229, #4690, .T. ) ;
#16161=ADVANCED_FACE ( 'NONE', ( #15848 ), #11027, .T. ) ;
#16165=CARTESIAN_POINT ( 'NONE',  ( -82.06839719201970240, -125.5578986320909962, 31.45126808048254219 ) ) ;
#16166=AXIS2_PLACEMENT_3D ( 'NONE', #16569, #14823, #4073 ) ;
#16171=DIRECTION ( 'NONE',  ( 1.000000000000000000, 0.000000000000000000, 0.000000000000000000 ) ) ;
#16172=CARTESIAN_POINT ( 'NONE',  ( 99.30949456653218022, -131.5229532012208722, 4.208660560896509750 ) ) ;
#16180=CARTESIAN_POINT ( 'NONE',  ( -122.8001410695374460, -86.14014948502065749, 49.99999999999999289 ) ) ;
#16182=ORIENTED_EDGE ( 'NONE', *, *, #19259, .T. ) ;
#16190=CARTESIAN_POINT ( 'NONE',  ( -110.0000000000000284, 101.9803902718557111, 44.99999999999998579 ) ) ;
#16195=CARTESIAN_POINT ( 'NONE',  ( -95.42019791134576678, -116.1393900958301231, 7.897240193129543506 ) ) ;
#16198=CARTESIAN_POINT ( 'NONE',  ( -139.6219990602459120, -10.61388033341743942, 23.64454228650399870 ) ) ;
#16203=CARTESIAN_POINT ( 'NONE',  ( -131.2702496982249727, -90.86622748991179321, 40.00000000000000000 ) ) ;
#16205=DIRECTION ( 'NONE',  ( 1.000000000000000000, 0.000000000000000000, 0.000000000000000000 ) ) ;
#16212=CARTESIAN_POINT ( 'NONE',  ( -128.2054629363889831, -77.87043913366071024, -8.142599671304674658 ) ) ;
#16219=CARTESIAN_POINT ( 'NONE',  ( -63.68887634719365565, -147.8252249328922687, 39.99999999999999289 ) ) ;
#16224=ORIENTED_EDGE ( 'NONE', *, *, #6778, .T. ) ;
#16237=CARTESIAN_POINT ( 'NONE',  ( -110.0000000000000142, 275.0000000000000000, 5.000000000000000888 ) ) ;
#16252=CARTESIAN_POINT ( 'NONE',  ( -139.3747594192856525, -22.29693483761631967, -14.06286033225251231 ) ) ;
#16259=ORIENTED_EDGE ( 'NONE', *, *, #4652, .F. ) ;
#16266=CARTESIAN_POINT ( 'NONE',  ( -86.10242266703171765, -122.8274731153598225, 42.46235246160556898 ) ) ;
#16271=CARTESIAN_POINT ( 'NONE',  ( 107.5000000000000142, -113.9901311517800053, 0.000000000000000000 ) ) ;
#16273=DIRECTION ( 'NONE',  ( 0.000000000000000000, 0.000000000000000000, -1.000000000000000000 ) ) ;
#16275=DIRECTION ( 'NONE',  ( -0.000000000000000000, -0.000000000000000000, -1.000000000000000000 ) ) ;
#16278=DIRECTION ( 'NONE',  ( 0.000000000000000000, 0.000000000000000000, -1.000000000000000000 ) ) ;
#16283=EDGE_CURVE ( 'NONE', #16530, #17276, #17215, .T. ) ;
#16284=VECTOR ( 'NONE', #11771, 1000.000000000000000 ) ;
#16286=CARTESIAN_POINT ( 'NONE',  ( -176.7850001792984926, -190.0000000000000284, 40.00000000000000000 ) ) ;
#16296=CARTESIAN_POINT ( 'NONE',  ( -101.9588377999664317, -127.6928792353688209, 1.652472148576846545 ) ) ;
#16299=CARTESIAN_POINT ( 'NONE',  ( -83.45731665390675857, -124.6394201399246384, 2.317304836764386700 ) ) ;
#16305=( NAMED_UNIT ( * ) PLANE_ANGLE_UNIT ( ) SI_UNIT ( $, .RADIAN. ) );
#16309=CARTESIAN_POINT ( 'NONE',  ( 15.91767397667354800, 164.0736214083062805, 39.99999999999999289 ) ) ;
#16310=FACE_OUTER_BOUND ( 'NONE', #4206, .T. ) ;
#16312=VECTOR ( 'NONE', #9405, 1000.000000000000000 ) ;
#16317=CARTESIAN_POINT ( 'NONE',  ( -163.5019688434124419, -20.99123081650240863, 49.99999999999999289 ) ) ;
#16322=CARTESIAN_POINT ( 'NONE',  ( -123.8648416762430884, -84.61253400034597405, -0.6186463947281112263 ) ) ;
#16323=CARTESIAN_POINT ( 'NONE',  ( 134.7747342791600715, -65.84665809079267262, 5.198213465029171587 ) ) ;
#16333=LINE ( 'NONE', #2319, #11833 ) ;
#16334=B_SPLINE_CURVE_WITH_KNOTS ( 'NONE', 3,
 ( #19080, #15900, #17647, #5066, #12719, #11389, #8013, #18980, #4965, #14260, #5167, #6697, #8316, #3623, #14460, #9849, #2193, #16102, #6597, #1881, #2091, #8421, #12919, #11289 ),
 .UNSPECIFIED., .F., .F.,
 ( 4, 2, 2, 2, 2, 2, 2, 2, 2, 2, 2, 4 ),
 ( 0.05875642544931597433, 0.06915854747235597455, 0.07956066949539594702, 0.08476173050691591937, 0.08736226101267591249, 0.08996279151843590560, 0.1003649135414758364, 0.1107670355645157811, 0.1211691575875557259, 0.1263702185990756843, 0.1315712796105956151, 0.1419734016336355320 ),
 .UNSPECIFIED. ) ;
#16338=DIRECTION ( 'NONE',  ( 1.000000000000000000, 0.000000000000000000, 0.000000000000000000 ) ) ;
#16344=VECTOR ( 'NONE', #7, 1000.000000000000000 ) ;
#16346=CARTESIAN_POINT ( 'NONE',  ( -135.2402195529228948, -30.09203172481036503, -19.25660886061671562 ) ) ;
#16349=ORIENTED_EDGE ( 'NONE', *, *, #6778, .F. ) ;
#16352=ORIENTED_EDGE ( 'NONE', *, *, #14398, .F. ) ;
#16361=ADVANCED_FACE ( 'NONE', ( #10691 ), #13660, .F. ) ;
#16362=CARTESIAN_POINT ( 'NONE',  ( -84.98223365279403652, -123.6049511534864962, 40.79306686164451889 ) ) ;
#16364=DIRECTION ( 'NONE',  ( 0.000000000000000000, 0.000000000000000000, 1.000000000000000000 ) ) ;
#16366=EDGE_CURVE ( 'NONE', #13930, #380, #4832, .T. ) ;
#16368=CARTESIAN_POINT ( 'NONE',  ( -128.9113527779074388, -76.70395394680458878, 47.60335545142810076 ) ) ;
#16369=CARTESIAN_POINT ( 'NONE',  ( 97.50000000000001421, -133.9542832461881119, 10.00000000000000178 ) ) ;
#16373=FACE_OUTER_BOUND ( 'NONE', #17695, .T. ) ;
#16374=CARTESIAN_POINT ( 'NONE',  ( 159.9599531637113330, -36.50981547336952104, 39.99999999999999289 ) ) ;
#16380=CARTESIAN_POINT ( 'NONE',  ( 0.000000000000000000, 0.000000000000000000, 49.99999999999999289 ) ) ;
#16387=DIRECTION ( 'NONE',  ( -0.000000000000000000, -0.000000000000000000, -1.000000000000000000 ) ) ;
#16391=CARTESIAN_POINT ( 'NONE',  ( 90.38423273154630522, -119.7175801288824317, -6.689658229812266654 ) ) ;
#16392=CARTESIAN_POINT ( 'NONE',  ( -85.51233150139636052, -123.2383548749651538, -1.612964112344334344 ) ) ;
#16394=CARTESIAN_POINT ( 'NONE',  ( -84.00455766787156620, -124.2712478689755642, 1.041419029133151097 ) ) ;
#16419=CARTESIAN_POINT ( 'NONE',  ( -127.3324793557758596, -79.33838548637069721, -0.8616620075509384691 ) ) ;
#16420=CARTESIAN_POINT ( 'NONE',  ( 135.0085555318104866, -65.36720921928018413, 6.996239623563403676 ) ) ;
#16422=EDGE_CURVE ( 'NONE', #14351, #14876, #3507, .T. ) ;
#16429=ORIENTED_EDGE ( 'NONE', *, *, #10136, .F. ) ;
#16432=DIRECTION ( 'NONE',  ( -0.6234898018587431423, 0.7818314824680221431, 0.000000000000000000 ) ) ;
#16434=CIRCLE ( 'NONE', #8260, 7.500000000000012434 ) ;
#16437=FACE_BOUND ( 'NONE', #18701, .T. ) ;
#16447=CARTESIAN_POINT ( 'NONE',  ( -134.6433994324794412, -73.52870175801841413, 7.634837572223202251 ) ) ;
#16458=DIRECTION ( 'NONE',  ( -1.613511099790691498E-16, 1.000000000000000000, 0.000000000000000000 ) ) ;
#16464=DIRECTION ( 'NONE',  ( 1.000000000000000000, 0.000000000000000000, 0.000000000000000000 ) ) ;
#16465=CARTESIAN_POINT ( 'NONE',  ( 159.9599531637113330, -36.50981547336952104, 39.99999999999999289 ) ) ;
#16466=EDGE_CURVE ( 'NONE', #5287, #7766, #14901, .T. ) ;
#16467=ORIENTED_EDGE ( 'NONE', *, *, #13371, .T. ) ;
#16469=DIRECTION ( 'NONE',  ( 1.000000000000000000, 0.000000000000000000, 0.000000000000000000 ) ) ;
#16471=DIRECTION ( 'NONE',  ( 0.000000000000000000, 0.000000000000000000, 1.000000000000000000 ) ) ;
#16473=ORIENTED_EDGE ( 'NONE', *, *, #6394, .T. ) ;
#16475=LINE ( 'NONE', #3885, #2851 ) ;
#16476=CYLINDRICAL_SURFACE ( 'NONE', #12754, 9.999999999999994671 ) ;
#16478=VERTEX_POINT ( 'NONE', #64 ) ;
#16484=ORIENTED_EDGE ( 'NONE', *, *, #19364, .T. ) ;
#16486=DIRECTION ( 'NONE',  ( -0.9009688679024219216, 0.4338837391175523472, 0.000000000000000000 ) ) ;
#16487=CIRCLE ( 'NONE', #14837, 7.500000000000003553 ) ;
#16489=CARTESIAN_POINT ( 'NONE',  ( 106.9434277525946868, -119.5160896407720941, -3.835367999719689524E-15 ) ) ;
#16490=CARTESIAN_POINT ( 'NONE',  ( -93.97987429417752026, -116.9112352313915295, -8.647211263555981020 ) ) ;
#16492=CARTESIAN_POINT ( 'NONE',  ( -139.9227089858103454, -5.347203697601174532, 23.15800849071695922 ) ) ;
#16495=CARTESIAN_POINT ( 'NONE',  ( -29.99999999999887379, 275.0000000000000000, -2.500000000000847766 ) ) ;
#16503=CARTESIAN_POINT ( 'NONE',  ( 7.500000000000001776, 60.00000000000000000, -105.0000000000000142 ) ) ;
#16504=EDGE_CURVE ( 'NONE', #18380, #14190, #10049, .T. ) ;
#16505=ORIENTED_EDGE ( 'NONE', *, *, #5262, .F. ) ;
#16507=ORIENTED_EDGE ( 'NONE', *, *, #5756, .T. ) ;
#16511=CARTESIAN_POINT ( 'NONE',  ( 130.9868171408399462, -91.88282611735539263, 0.000000000000000000 ) ) ;
#16514=CARTESIAN_POINT ( 'NONE',  ( -99.73767742490161936, -112.0463336856493299, 50.00000000005213963 ) ) ;
#16522=CARTESIAN_POINT ( 'NONE',  ( -132.9399949862640824, -69.60197982539851580, 33.36755373876824393 ) ) ;
#16529=AXIS2_PLACEMENT_3D ( 'NONE', #7220, #6829, #10372 ) ;
#16530=VERTEX_POINT ( 'NONE', #1603 ) ;
#16539=DIRECTION ( 'NONE',  ( 0.000000000000000000, 0.000000000000000000, 1.000000000000000000 ) ) ;
#16543=CARTESIAN_POINT ( 'NONE',  ( -150.0000000000000284, 0.000000000000000000, -10.00000000000000178 ) ) ;
#16545=VECTOR ( 'NONE', #18663, 1000.000000000000000 ) ;
#16559=CARTESIAN_POINT ( 'NONE',  ( 138.2024300533213932, 89.85329105948596862, 39.99999999999999289 ) ) ;
#16561=CARTESIAN_POINT ( 'NONE',  ( -83.87053960371946459, -124.3614079552663441, 38.64581828052915569 ) ) ;
#16562=FACE_OUTER_BOUND ( 'NONE', #5395, .T. ) ;
#16563=DIRECTION ( 'NONE',  ( 0.000000000000000000, -0.000000000000000000, -1.000000000000000000 ) ) ;
#16564=ORIENTED_EDGE ( 'NONE', *, *, #15623, .F. ) ;
#16565=CIRCLE ( 'NONE', #13284, 15.91767397667355155 ) ;
#16566=CARTESIAN_POINT ( 'NONE',  ( -135.1060089022256818, -65.16414933467417825, 30.00000000000000000 ) ) ;
#16569=CARTESIAN_POINT ( 'NONE',  ( 0.000000000000000000, 0.000000000000000000, -9.999999999999987566 ) ) ;
#16578=ORIENTED_EDGE ( 'NONE', *, *, #5787, .T. ) ;
#16582=DIRECTION ( 'NONE',  ( -0.4338837391175523472, -0.9009688679024219216, 0.000000000000000000 ) ) ;
#16584=CYLINDRICAL_SURFACE ( 'NONE', #3449, 40.00000000000000711 ) ;
#16596=VERTEX_POINT ( 'NONE', #7676 ) ;
#16604=CARTESIAN_POINT ( 'NONE',  ( 131.9731329243527398, -88.11278280481133152, 0.2335709844691223058 ) ) ;
#16608=CARTESIAN_POINT ( 'NONE',  ( -106.3851141486743188, -120.5004170265707444, 39.95383784551692941 ) ) ;
#16609=EDGE_CURVE ( 'NONE', #1203, #19359, #8400, .T. ) ;
#16614=CYLINDRICAL_SURFACE ( 'NONE', #8784, 15.91767397667354089 ) ;
#16615=CARTESIAN_POINT ( 'NONE',  ( -128.0922826834541297, -78.05640312850694329, -8.225544806820535015 ) ) ;
#16619=FACE_OUTER_BOUND ( 'NONE', #12917, .T. ) ;
#16624=EDGE_CURVE ( 'NONE', #2833, #19796, #15588, .T. ) ;
#16632=CARTESIAN_POINT ( 'NONE',  ( -97.49999999999997158, -190.0000000000000000, 30.00000000000000000 ) ) ;
#16639=CARTESIAN_POINT ( 'NONE',  ( -159.9599531637108782, -36.50981547337168109, 39.99999999999999289 ) ) ;
#16641=CARTESIAN_POINT ( 'NONE',  ( -134.5752827950141466, -74.04736996659983106, 6.800259422634988837 ) ) ;
#16643=CARTESIAN_POINT ( 'NONE',  ( 126.7530218919796567, -80.25302646197467027, 40.98242217817278998 ) ) ;
#16656=SURFACE_STYLE_USAGE ( .BOTH. , #18187 ) ;
#16657=CARTESIAN_POINT ( 'NONE',  ( 100.7812500000000000, -111.0996833858562525, 49.99999999999999289 ) ) ;
#16665=ADVANCED_FACE ( 'NONE', ( #4510, #10633 ), #15348, .T. ) ;
#16674=LINE ( 'NONE', #1108, #1074 ) ;
#16679=CARTESIAN_POINT ( 'NONE',  ( -82.42180963433014540, -125.3261898519405548, 34.07777747112352529 ) ) ;
#16684=CARTESIAN_POINT ( 'NONE',  ( 95.54273718349524813, -115.6434791701545493, -9.240355742637868630 ) ) ;
#16685=CARTESIAN_POINT ( 'NONE',  ( -96.59694518724896284, -114.7646842535148437, -9.528509010735914941 ) ) ;
#16701=VERTEX_POINT ( 'NONE', #7982 ) ;
#16704=CARTESIAN_POINT ( 'NONE',  ( 134.6416478978700013, -73.54075392783713028, 7.639997785598048097 ) ) ;
#16712=CARTESIAN_POINT ( 'NONE',  ( -133.1515905083418545, -69.19806146153663917, 7.897424385335312103 ) ) ;
#16713=CARTESIAN_POINT ( 'NONE',  ( 133.0181789769776231, -69.32831038615340447, -1.486944123354709824 ) ) ;
#16722=VERTEX_POINT ( 'NONE', #17515 ) ;
#16725=CARTESIAN_POINT ( 'NONE',  ( -101.6421356237309226, -200.0000000000000000, 39.99999999999999289 ) ) ;
#16728=FACE_OUTER_BOUND ( 'NONE', #4421, .T. ) ;
#16730=EDGE_CURVE ( 'NONE', #1702, #3019, #16565, .T. ) ;
#16732=CARTESIAN_POINT ( 'NONE',  ( -100.5012343356710289, 87.83131483863925837, -28.71515701202468662 ) ) ;
#16736=CARTESIAN_POINT ( 'NONE',  ( 126.6692879288199833, -80.35371549669886804, 49.11974464924469430 ) ) ;
#16739=DIRECTION ( 'NONE',  ( 0.000000000000000000, 0.000000000000000000, -1.000000000000000000 ) ) ;
#16741=AXIS2_PLACEMENT_3D ( 'NONE', #13399, #13296, #19650 ) ;
#16745=CARTESIAN_POINT ( 'NONE',  ( -110.0000000000000142, 275.0000000000000000, -94.99999999999997158 ) ) ;
#16747=ORIENTED_EDGE ( 'NONE', *, *, #14869, .F. ) ;
#16755=ADVANCED_FACE ( 'NONE', ( #14335 ), #5785, .T. ) ;
#16756=CARTESIAN_POINT ( 'NONE',  ( -127.1451880273208275, -79.59002392720336161, 48.83712415753068825 ) ) ;
#16765=CARTESIAN_POINT ( 'NONE',  ( -85.67694800211594952, 110.7245732599958359, 30.17800178787670262 ) ) ;
#16769=CIRCLE ( 'NONE', #11845, 42.50000000000000000 ) ;
#16770=VERTEX_POINT ( 'NONE', #9821 ) ;
#16775=CARTESIAN_POINT ( 'NONE',  ( -83.25760956674176327, -124.7743995867136988, 37.25730000191769165 ) ) ;
#16777=ORIENTED_EDGE ( 'NONE', *, *, #13371, .F. ) ;
#16779=CARTESIAN_POINT ( 'NONE',  ( 60.00000000000000711, 6.284666409917639535E-13, -105.0000000000000142 ) ) ;
#16782=CARTESIAN_POINT ( 'NONE',  ( 104.7061264979155055, -123.3530444481632742, 0.3798221288333544221 ) ) ;
#16788=CARTESIAN_POINT ( 'NONE',  ( -109.9999999999983515, 265.0000000000000000, 92.50000000000004263 ) ) ;
#16794=CARTESIAN_POINT ( 'NONE',  ( -110.0000000000000142, 275.0000000000000000, -82.50000000000001421 ) ) ;
#16796=EDGE_LOOP ( 'NONE', ( #15359, #10929, #13970, #5522, #6099 ) ) ;
#16810=LINE ( 'NONE', #7805, #9101 ) ;
#16813=CARTESIAN_POINT ( 'NONE',  ( -134.6725548700739239, -73.30144156569457436, 8.133873478739229057 ) ) ;
#16814=CARTESIAN_POINT ( 'NONE',  ( 124.3929425833901803, -83.83509237772305767, -9.887605300484166193 ) ) ;
#16816=CARTESIAN_POINT ( 'NONE',  ( -7.499999999999583444, -60.00000000000000000, -100.0000000000000000 ) ) ;
#16817=CARTESIAN_POINT ( 'NONE',  ( -134.6061912685141522, -66.19056267105416680, 35.86613249723460228 ) ) ;
#16820=AXIS2_PLACEMENT_3D ( 'NONE', #4999, #8049, #6536 ) ;
#16821=ORIENTED_EDGE ( 'NONE', *, *, #7233, .F. ) ;
#16824=( BOUNDED_CURVE ( )  B_SPLINE_CURVE ( 3, ( #15199, #19909, #7326, #16949 ),
 .UNSPECIFIED., .F., .F. ) 
 B_SPLINE_CURVE_WITH_KNOTS ( ( 4, 4 ),
 ( 1.570796326794896336, 1.920639998745670596 ),
 .UNSPECIFIED. ) 
 CURVE ( )  GEOMETRIC_REPRESENTATION_ITEM ( )  RATIONAL_B_SPLINE_CURVE ( ( 1.000000000000000000, 0.9898267632596812193, 0.9898267632596812193, 1.000000000000000000 ) ) 
 REPRESENTATION_ITEM ( '' )  );
#16825=ORIENTED_EDGE ( 'NONE', *, *, #13442, .T. ) ;
#16827=DIRECTION ( 'NONE',  ( -1.000000000000000000, 0.000000000000000000, -0.000000000000000000 ) ) ;
#16831=CARTESIAN_POINT ( 'NONE',  ( -134.7652707650784407, -31.41120252075685215, -19.73219286542039441 ) ) ;
#16833=ORIENTED_EDGE ( 'NONE', *, *, #649, .F. ) ;
#16848=DIRECTION ( 'NONE',  ( 1.613511099790691498E-16, -1.000000000000000000, -0.000000000000000000 ) ) ;
#16852=CARTESIAN_POINT ( 'NONE',  ( -78.68887634719366986, -147.8252249328922687, 39.99999999999999289 ) ) ;
#16857=VECTOR ( 'NONE', #9337, 1000.000000000000000 ) ;
#16858=ORIENTED_EDGE ( 'NONE', *, *, #16862, .T. ) ;
#16862=EDGE_CURVE ( 'NONE', #9612, #12285, #4461, .T. ) ;
#16863=EDGE_CURVE ( 'NONE', #796, #10476, #11336, .T. ) ;
#16866=CARTESIAN_POINT ( 'NONE',  ( -134.2294018150276429, -76.49442575693799995, 35.55695887397251909 ) ) ;
#16867=DIRECTION ( 'NONE',  ( 1.000000000000000000, 3.320906611023727849E-16, 0.000000000000000000 ) ) ;
#16868=ORIENTED_EDGE ( 'NONE', *, *, #16422, .T. ) ;
#16873=ORIENTED_EDGE ( 'NONE', *, *, #14144, .F. ) ;
#16875=CARTESIAN_POINT ( 'NONE',  ( -97.21757233051278035, -115.5955488200699932, 29.66285830273704605 ) ) ;
#16876=AXIS2_PLACEMENT_3D ( 'NONE', #9784, #18135, #15160 ) ;
#16882=CARTESIAN_POINT ( 'NONE',  ( 100.4512631336869504, -129.9078745865736551, 2.904715523906934216 ) ) ;
#16883=DIRECTION ( 'NONE',  ( 0.000000000000000000, 0.000000000000000000, 1.000000000000000000 ) ) ;
#16885=CIRCLE ( 'NONE', #6448, 7.500000000000000000 ) ;
#16887=CARTESIAN_POINT ( 'NONE',  ( -136.7584521108019260, -24.61299102371015479, -18.63592354355825620 ) ) ;
#16889=FACE_BOUND ( 'NONE', #14459, .T. ) ;
#16890=DIRECTION ( 'NONE',  ( 0.000000000000000000, 0.000000000000000000, 1.000000000000000000 ) ) ;
#16893=CARTESIAN_POINT ( 'NONE',  ( 96.53160196460632392, -115.8699919790352908, 29.79840038410488745 ) ) ;
#16909=LINE ( 'NONE', #10447, #9957 ) ;
#16911=LINE ( 'NONE', #18140, #11061 ) ;
#16913=FACE_OUTER_BOUND ( 'NONE', #12836, .T. ) ;
#16918=CARTESIAN_POINT ( 'NONE',  ( 131.7304022393856258, -71.85445963696412264, 3.108710632514347871 ) ) ;
#16920=CARTESIAN_POINT ( 'NONE',  ( -97.49999999999998579, -133.9542832461881687, 30.00000000000000000 ) ) ;
#16921=CARTESIAN_POINT ( 'NONE',  ( -133.5298479455752840, -80.72596075552313266, 37.84186899868029741 ) ) ;
#16925=AXIS2_PLACEMENT_3D ( 'NONE', #4872, #6204, #14375 ) ;
#16930=CARTESIAN_POINT ( 'NONE',  ( -141.7593571144487044, -18.51227725722888096, 19.71492705251383981 ) ) ;
#16933=VERTEX_POINT ( 'NONE', #17811 ) ;
#16939=CARTESIAN_POINT ( 'NONE',  ( -91.39357229321551301, 100.9612215610973038, -24.64723702058964605 ) ) ;
#16942=CYLINDRICAL_SURFACE ( 'NONE', #15000, 150.0000000000000284 ) ;
#16949=CARTESIAN_POINT ( 'NONE',  ( -176.7850001792984926, -190.0000000000000284, 33.42750952962406075 ) ) ;
#16951=AXIS2_PLACEMENT_3D ( 'NONE', #18712, #4800, #6335 ) ;
#16953=ORIENTED_EDGE ( 'NONE', *, *, #1642, .F. ) ;
#16955=CIRCLE ( 'NONE', #14974, 150.0000000000000284 ) ;
#16968=CIRCLE ( 'NONE', #4543, 150.0000000000000284 ) ;
#16974=VERTEX_POINT ( 'NONE', #713 ) ;
#16975=DIRECTION ( 'NONE',  ( 1.000000000000000000, 0.000000000000000000, 0.000000000000000000 ) ) ;
#16980=EDGE_CURVE ( 'NONE', #9322, #16974, #16475, .T. ) ;
#16985=CARTESIAN_POINT ( 'NONE',  ( -109.9999999999983515, 265.0000000000000000, 85.00000000000001421 ) ) ;
#16988=CARTESIAN_POINT ( 'NONE',  ( 97.58310720701103946, -133.8455726501578908, 8.700002021410107034 ) ) ;
#16991=CARTESIAN_POINT ( 'NONE',  ( -135.7615415765321814, -31.23721399736636428, -16.61340895829727060 ) ) ;
#16998=DIRECTION ( 'NONE',  ( 0.000000000000000000, 0.000000000000000000, 1.000000000000000000 ) ) ;
#17000=CARTESIAN_POINT ( 'NONE',  ( 99.35657680079279430, -131.4542451999401749, 35.80648205613542956 ) ) ;
#17006=EDGE_CURVE ( 'NONE', #383, #9853, #5146, .T. ) ;
#17015=CARTESIAN_POINT ( 'NONE',  ( 166.7850001792985495, -199.9999999999999716, 40.00000000000000000 ) ) ;
#17017=CARTESIAN_POINT ( 'NONE',  ( -100.4512631336862825, -129.9078745865736551, 37.09528447609245916 ) ) ;
#17021=CARTESIAN_POINT ( 'NONE',  ( -133.9967726966432053, -77.99266392030686745, 3.479247166016994353 ) ) ;
#17023=CARTESIAN_POINT ( 'NONE',  ( 128.4532923017994506, -77.52586173742918163, -0.4241867359497863976 ) ) ;
#17026=CARTESIAN_POINT ( 'NONE',  ( -125.0010599886705620, -82.93257931481025480, 40.94260748306679432 ) ) ;
#17029=DIRECTION ( 'NONE',  ( -1.000000000000000000, 0.000000000000000000, 0.000000000000000000 ) ) ;
#17031=ORIENTED_EDGE ( 'NONE', *, *, #7063, .T. ) ;
#17035=EDGE_CURVE ( 'NONE', #2271, #12416, #13474, .T. ) ;
#17046=CARTESIAN_POINT ( 'NONE',  ( -90.37486697571327454, 102.3558818120413321, -23.98309657527855165 ) ) ;
#17051=CARTESIAN_POINT ( 'NONE',  ( 131.8415137303879874, -71.65490762087030419, 36.74244028875413193 ) ) ;
#17068=DIRECTION ( 'NONE',  ( 0.000000000000000000, 1.000000000000000000, 0.000000000000000000 ) ) ;
#17071=DIRECTION ( 'NONE',  ( 0.000000000000000000, 0.000000000000000000, 1.000000000000000000 ) ) ;
#17075=FACE_OUTER_BOUND ( 'NONE', #866, .T. ) ;
#17076=CARTESIAN_POINT ( 'NONE',  ( -77.41967535438791970, 116.6460954727662767, 17.81468430219124244 ) ) ;
#17078=CARTESIAN_POINT ( 'NONE',  ( 148.9554720520395108, -17.67108784863215476, 39.99999999999999289 ) ) ;
#17089=CARTESIAN_POINT ( 'NONE',  ( 82.80829968034944955, -125.0716697069634336, 4.111516946209861523 ) ) ;
#17093=ORIENTED_EDGE ( 'NONE', *, *, #6909, .F. ) ;
#17095=DIRECTION ( 'NONE',  ( 0.000000000000000000, 0.000000000000000000, -1.000000000000000000 ) ) ;
#17098=CARTESIAN_POINT ( 'NONE',  ( 97.50000000000001421, -133.9542832461881687, 30.00000000000000000 ) ) ;
#17110=CARTESIAN_POINT ( 'NONE',  ( 141.8871031824808995, -16.05777877957299538, 39.99999999999999289 ) ) ;
#17111=EDGE_CURVE ( 'NONE', #1300, #18061, #4153, .T. ) ;
#17113=MECHANICAL_DESIGN_GEOMETRIC_PRESENTATION_REPRESENTATION('',(#5053),#3069);
#17114=ORIENTED_EDGE ( 'NONE', *, *, #18155, .F. ) ;
#17117=CARTESIAN_POINT ( 'NONE',  ( 133.3415482518558406, -68.70949856429523095, 40.71953839863250124 ) ) ;
#17118=CARTESIAN_POINT ( 'NONE',  ( -95.45795901651536042, -116.1130648478386291, 32.13249062836397485 ) ) ;
#17119=CARTESIAN_POINT ( 'NONE',  ( -167.4599531637108782, -36.50981547337168109, 39.99999999999999289 ) ) ;
#17124=CARTESIAN_POINT ( 'NONE',  ( 132.9666886943622330, -83.66363014848037949, 1.140117263048182616 ) ) ;
#17129=CARTESIAN_POINT ( 'NONE',  ( -133.6471402512195539, -68.10643054410131469, 39.75618603187317035 ) ) ;
#17132=DIRECTION ( 'NONE',  ( -0.000000000000000000, 0.000000000000000000, -1.000000000000000000 ) ) ;
#17137=EDGE_CURVE ( 'NONE', #7108, #15648, #7423, .T. ) ;
#17140=CARTESIAN_POINT ( 'NONE',  ( -145.0046799159938473, -14.11398466591643341, 5.837281836175630900 ) ) ;
#17144=ORIENTED_EDGE ( 'NONE', *, *, #11490, .F. ) ;
#17146=LINE ( 'NONE', #8225, #1627 ) ;
#17147=CARTESIAN_POINT ( 'NONE',  ( -90.03415420018352222, 102.8177110809194801, -23.74958468013522506 ) ) ;
#17155=PRODUCT_DEFINITION ( 'UNKNOWN', '', #8512, #10076 ) ;
#17157=CARTESIAN_POINT ( 'NONE',  ( 130.7712900376312462, -73.57687123476455326, 38.42272532816287622 ) ) ;
#17160=ORIENTED_EDGE ( 'NONE', *, *, #237, .T. ) ;
#17161=ORIENTED_EDGE ( 'NONE', *, *, #17035, .F. ) ;
#17164=CARTESIAN_POINT ( 'NONE',  ( 148.9554720520395392, -17.67108784863215831, 49.99999999999999289 ) ) ;
#17168=AXIS2_PLACEMENT_3D ( 'NONE', #16465, #4067, #2648 ) ;
#17173=ORIENTED_EDGE ( 'NONE', *, *, #19019, .F. ) ;
#17175=CARTESIAN_POINT ( 'NONE',  ( 67.50000000000000000, 6.284666409917639535E-13, -105.0000000000000142 ) ) ;
#17177=B_SPLINE_CURVE_WITH_KNOTS ( 'NONE', 3,
 ( #18814, #5100, #12952, #180, #15937, #19211, #14499, #1925, #3257, #14400, #11218, #5201, #11015, #3454, #17582, #12758, #4903, #381, #8351, #8251, #11430, #6633, #484, #11326, #12857, #17481 ),
 .UNSPECIFIED., .F., .F.,
 ( 4, 2, 2, 2, 2, 2, 2, 2, 2, 2, 2, 2, 4 ),
 ( 0.000000000000000000, 0.004334419010350961353, 0.006501628515526464147, 0.008668838020701969543, 0.01300325703105293350, 0.01517046653622841808, 0.01733767604140390439, 0.02167209505175490478, 0.02383930455693041364, 0.02600651406210592251, 0.02817372356728143831, 0.03034093307245694718, 0.03467535208280797532 ),
 .UNSPECIFIED. ) ;
#17187=ORIENTED_EDGE ( 'NONE', *, *, #11246, .F. ) ;
#17192=CARTESIAN_POINT ( 'NONE',  ( 82.03125000000004263, -125.5821405433013638, 49.99999999999999289 ) ) ;
#17193=ORIENTED_EDGE ( 'NONE', *, *, #11104, .T. ) ;
#17205=CARTESIAN_POINT ( 'NONE',  ( -159.9599531637108782, -36.50981547337168109, 49.99999999999999289 ) ) ;
#17206=DIRECTION ( 'NONE',  ( 0.000000000000000000, 0.000000000000000000, 1.000000000000000000 ) ) ;
#17209=ORIENTED_EDGE ( 'NONE', *, *, #13900, .T. ) ;
#17212=DIRECTION ( 'NONE',  ( 1.000000000000000000, -2.775557561562892929E-15, 0.000000000000000000 ) ) ;
#17213=ORIENTED_EDGE ( 'NONE', *, *, #13864, .T. ) ;
#17215=CIRCLE ( 'NONE', #6441, 150.0000000000000284 ) ;
#17218=ORIENTED_EDGE ( 'NONE', *, *, #7233, .T. ) ;
#17219=CARTESIAN_POINT ( 'NONE',  ( -106.5742148451189877, -120.1859338240075914, 3.408460579751304959E-15 ) ) ;
#17220=LINE ( 'NONE', #1561, #3806 ) ;
#17224=CARTESIAN_POINT ( 'NONE',  ( -97.49999999999997158, -133.9542832455804273, 9.244933322737061587 ) ) ;
#17227=CARTESIAN_POINT ( 'NONE',  ( -98.61806909068833704, -132.4668554876671180, 34.59818424444248564 ) ) ;
#17228=CARTESIAN_POINT ( 'NONE',  ( -7.500000000000001776, 60.00000000000000000, -105.0000000000000142 ) ) ;
#17229=CARTESIAN_POINT ( 'NONE',  ( -126.6026197240541791, 59.88689088082667666, 35.86430457606912370 ) ) ;
#17230=AXIS2_PLACEMENT_3D ( 'NONE', #19050, #3487, #3390 ) ;
#17231=CARTESIAN_POINT ( 'NONE',  ( 97.50000000000002842, -199.9999999999999716, 10.00000000000000178 ) ) ;
#17234=CARTESIAN_POINT ( 'NONE',  ( -134.3401481871931651, -66.72943863802690601, 37.23267499212099807 ) ) ;
#17235=EDGE_CURVE ( 'NONE', #11160, #10982, #3833, .T. ) ;
#17239=VERTEX_POINT ( 'NONE', #3063 ) ;
#17244=EDGE_CURVE ( 'NONE', #2173, #14190, #88, .T. ) ;
#17247=CARTESIAN_POINT ( 'NONE',  ( -15.91767397667354800, 164.0736214083062805, 39.99999999999999289 ) ) ;
#17250=CARTESIAN_POINT ( 'NONE',  ( -134.7188131032333445, -72.93593548660989256, 10.00000000000000178 ) ) ;
#17254=VECTOR ( 'NONE', #11012, 1000.000000000000000 ) ;
#17255=ADVANCED_FACE ( 'NONE', ( #19025 ), #15741, .T. ) ;
#17258=CARTESIAN_POINT ( 'NONE',  ( 134.6725548700753734, -73.30144156569930658, 31.86612652126208900 ) ) ;
#17259=CARTESIAN_POINT ( 'NONE',  ( 133.1916981995338460, -82.53555109165358772, 38.51379023202792951 ) ) ;
#17261=ORIENTED_EDGE ( 'NONE', *, *, #16132, .T. ) ;
#17265=ADVANCED_FACE ( 'NONE', ( #4805 ), #19121, .T. ) ;
#17266=ORIENTED_EDGE ( 'NONE', *, *, #9967, .F. ) ;
#17275=CARTESIAN_POINT ( 'NONE',  ( 77.50000000000000000, 0.000000000000000000, -100.0000000000000000 ) ) ;
#17276=VERTEX_POINT ( 'NONE', #18925 ) ;
#17277=DIRECTION ( 'NONE',  ( 0.000000000000000000, 0.000000000000000000, 1.000000000000000000 ) ) ;
#17285=CARTESIAN_POINT ( 'NONE',  ( 86.01343624116272224, 31.38211805825951473, 30.00000000000000000 ) ) ;
#17286=DIRECTION ( 'NONE',  ( 0.000000000000000000, 0.000000000000000000, 1.000000000000000000 ) ) ;
#17287=CARTESIAN_POINT ( 'NONE',  ( 92.21618480002784679, -118.3073397699785829, 47.80227178660424414 ) ) ;
#17288=AXIS2_PLACEMENT_3D ( 'NONE', #397, #11034, #6553 ) ;
#17289=CIRCLE ( 'NONE', #7794, 150.0000000000000284 ) ;
#17299=DIRECTION ( 'NONE',  ( 0.000000000000000000, 1.000000000000000000, 0.000000000000000000 ) ) ;
#17301=EDGE_LOOP ( 'NONE', ( #16825, #19228, #10790, #17793 ) ) ;
#17304=CYLINDRICAL_SURFACE ( 'NONE', #3435, 15.91767397667354089 ) ;
#17307=EDGE_CURVE ( 'NONE', #18133, #19595, #9798, .T. ) ;
#17309=DIRECTION ( 'NONE',  ( -0.000000000000000000, -0.000000000000000000, -1.000000000000000000 ) ) ;
#17310=DIRECTION ( 'NONE',  ( 0.000000000000000000, -1.000000000000000000, 0.000000000000000000 ) ) ;
#17312=CARTESIAN_POINT ( 'NONE',  ( -15.91767397667354800, 164.0736214083062805, 39.99999999999999289 ) ) ;
#17316=CARTESIAN_POINT ( 'NONE',  ( 84.44144489238081519, -123.9750712224027467, 39.83491645190957797 ) ) ;
#17319=CARTESIAN_POINT ( 'NONE',  ( -72.27300218572868573, 131.4418965710077885, 18.41322297944785191 ) ) ;
#17320=VERTEX_POINT ( 'NONE', #17591 ) ;
#17324=ORIENTED_EDGE ( 'NONE', *, *, #19059, .T. ) ;
#17328=B_SPLINE_CURVE_WITH_KNOTS ( 'NONE', 3,
 ( #10328, #13195, #2471, #3708, #10237, #9947, #16198, #16492, #8703, #2083 ),
 .UNSPECIFIED., .F., .F.,
 ( 4, 2, 2, 2, 4 ),
 ( -0.03180955504969720099, -0.02385716628727290248, -0.01590477752484860396, -0.007952388762424298513, 6.938893903907228378E-18 ),
 .UNSPECIFIED. ) ;
#17333=CARTESIAN_POINT ( 'NONE',  ( 123.6381990918736449, -84.94542618836281633, 49.99999999999999289 ) ) ;
#17335=CARTESIAN_POINT ( 'NONE',  ( -104.7061264978949708, -123.3530444481632742, 39.62017787115935619 ) ) ;
#17337=CARTESIAN_POINT ( 'NONE',  ( -137.3272859360866676, 27.29364767066081754, 26.87729632077950725 ) ) ;
#17339=CARTESIAN_POINT ( 'NONE',  ( -149.9468681919209700, 4.311564970281852816, 2.773916037623369135 ) ) ;
#17340=CARTESIAN_POINT ( 'NONE',  ( -50.37374754117255549, -141.2886604036510221, 39.99999999999999289 ) ) ;
#17342=CARTESIAN_POINT ( 'NONE',  ( -130.6561114389107274, -73.68416578909176451, 45.68373799725728901 ) ) ;
#17344=DIRECTION ( 'NONE',  ( 0.000000000000000000, 0.000000000000000000, 1.000000000000000000 ) ) ;
#17346=CARTESIAN_POINT ( 'NONE',  ( -82.03124999999998579, -125.5821405433014064, 30.00000000000000000 ) ) ;
#17347=EDGE_LOOP ( 'NONE', ( #15560, #14369, #10943, #15159 ) ) ;
#17348=CIRCLE ( 'NONE', #11754, 9.999999999999994671 ) ;
#17349=ORIENTED_EDGE ( 'NONE', *, *, #11334, .F. ) ;
#17358=DIRECTION ( 'NONE',  ( -0.6234898018587431423, 0.7818314824680221431, 0.000000000000000000 ) ) ;
#17359=CARTESIAN_POINT ( 'NONE',  ( 97.67667160654319503, -133.7228621772585200, 31.88576057819609488 ) ) ;
#17362=ORIENTED_EDGE ( 'NONE', *, *, #12374, .F. ) ;
#17369=CARTESIAN_POINT ( 'NONE',  ( 0.000000000000000000, 0.000000000000000000, -10.00000000000000178 ) ) ;
#17370=AXIS2_PLACEMENT_3D ( 'NONE', #3479, #17508, #5128 ) ;
#17374=EDGE_CURVE ( 'NONE', #13130, #11866, #6421, .T. ) ;
#17375=CARTESIAN_POINT ( 'NONE',  ( -99.75421581617491995, -130.9036673766147771, 36.36146831168105820 ) ) ;
#17383=CARTESIAN_POINT ( 'NONE',  ( -91.75873705015325754, 111.3640350795034237, -30.64689026788566650 ) ) ;
#17387=EDGE_CURVE ( 'NONE', #2503, #5679, #7097, .T. ) ;
#17389=LINE ( 'NONE', #1721, #10442 ) ;
#17395=ORIENTED_EDGE ( 'NONE', *, *, #4478, .T. ) ;
#17396=PLANE ( 'NONE',  #16118 ) ;
#17397=B_SPLINE_CURVE_WITH_KNOTS ( 'NONE', 3,
 ( #15014, #2150, #16165, #10114, #7242, #602, #5709, #11825, #8476, #16561, #4065, #6847, #894, #16362, #13071, #16266, #2541, #2247, #11641, #3677, #6945, #5315, #17897, #18090, #11546, #13461, #14911, #14715, #7150, #8770 ),
 .UNSPECIFIED., .F., .F.,
 ( 4, 2, 2, 2, 2, 2, 2, 2, 2, 2, 2, 2, 2, 2, 4 ),
 ( 0.000000000000000000, 0.002172065812121075617, 0.003258098718181600198, 0.004344131624242125213, 0.008688263248484262569, 0.009774296154544809268, 0.01086032906060535250, 0.01303239487272644069, 0.01520446068484753062, 0.01737652649696861881, 0.02172065812121076397, 0.02389272393333180880, 0.02606478974545285016, 0.03040892136969493634, 0.03475305299393702252 ),
 .UNSPECIFIED. ) ;
#17398=EDGE_LOOP ( 'NONE', ( #6818, #16137 ) ) ;
#17400=EDGE_CURVE ( 'NONE', #2029, #13843, #17784, .T. ) ;
#17416=CARTESIAN_POINT ( 'NONE',  ( 105.2683707665266297, -122.4156632037704071, 39.76425450544135032 ) ) ;
#17418=AXIS2_PLACEMENT_3D ( 'NONE', #2678, #15349, #9212 ) ;
#17422=CARTESIAN_POINT ( 'NONE',  ( -81.44151772932448807, 125.9672356422290562, 33.01992119261491609 ) ) ;
#17430=DIRECTION ( 'NONE',  ( -0.000000000000000000, -0.000000000000000000, -1.000000000000000000 ) ) ;
#17431=CARTESIAN_POINT ( 'NONE',  ( -116.5489102618968360, 94.45925147717298387, 44.49316384199085661 ) ) ;
#17432=EDGE_CURVE ( 'NONE', #9376, #2619, #1230, .T. ) ;
#17438=CARTESIAN_POINT ( 'NONE',  ( -95.41207185104575217, -115.7515782192335365, -9.200900026191284553 ) ) ;
#17443=ADVANCED_FACE ( 'NONE', ( #8661 ), #14898, .F. ) ;
#17446=FACE_BOUND ( 'NONE', #13136, .T. ) ;
#17452=AXIS2_PLACEMENT_3D ( 'NONE', #8759, #10195, #6938 ) ;
#17454=CARTESIAN_POINT ( 'NONE',  ( -144.0189762191472767, -15.32165204522277868, 13.24322322583874367 ) ) ;
#17463=CARTESIAN_POINT ( 'NONE',  ( 97.53517841124886445, -133.9083944458742224, 30.96027505812804748 ) ) ;
#17469=EDGE_LOOP ( 'NONE', ( #1582, #19919 ) ) ;
#17476=CARTESIAN_POINT ( 'NONE',  ( -110.0000000000000000, 88.56916956954178488, -34.99999999999998579 ) ) ;
#17481=CARTESIAN_POINT ( 'NONE',  ( 135.1060089022256818, -65.16414933467422088, 10.00000000000000355 ) ) ;
#17486=AXIS2_PLACEMENT_3D ( 'NONE', #8383, #6761, #12983 ) ;
#17487=DIRECTION ( 'NONE',  ( 0.000000000000000000, 0.000000000000000000, -1.000000000000000000 ) ) ;
#17490=CARTESIAN_POINT ( 'NONE',  ( 90.17913298585700943, -119.8669913176027393, 46.50836399418985678 ) ) ;
#17491=VERTEX_POINT ( 'NONE', #9057 ) ;
#17494=ORIENTED_EDGE ( 'NONE', *, *, #4414, .T. ) ;
#17496=CARTESIAN_POINT ( 'NONE',  ( -152.4599531637108498, -36.50981547337168109, 49.99999999999999289 ) ) ;
#17499=( BOUNDED_SURFACE ( )  B_SPLINE_SURFACE ( 3, 2, ( 
 ( #2401, #7003, #853 ),
 ( #5466, #11499, #13222 ),
 ( #8434, #16322, #6907 ),
 ( #2306, #4026, #13319 ),
 ( #14964, #14677, #4124 ),
 ( #8728, #10354, #5373 ),
 ( #16615, #19674, #19577 ),
 ( #5567, #16419, #15068 ),
 ( #8632, #1047, #11692 ),
 ( #7296, #13525, #5274 ),
 ( #17958, #663, #13120 ),
 ( #19386, #11598, #17850 ),
 ( #3827, #3927, #8926 ),
 ( #5770, #18241, #17021 ),
 ( #1467, #1153, #20080 ),
 ( #18555, #7394, #4229 ),
 ( #10661, #15271, #10452 ),
 ( #4537, #13732, #1258 ),
 ( #5974, #2805, #10769 ),
 ( #19873, #3008, #15170 ),
 ( #5874, #13628, #12299 ),
 ( #9237, #4323, #16813 ),
 ( #11987, #16712, #10557 ),
 ( #2697, #9028, #6079 ),
 ( #3111, #15482, #12088 ),
 ( #18348, #7697, #12406 ) ),
 .UNSPECIFIED., .F., .F., .F. ) 
 B_SPLINE_SURFACE_WITH_KNOTS ( ( 4, 2, 2, 2, 2, 2, 2, 2, 2, 2, 2, 2, 4 ),
 ( 3, 3 ),
 ( 0.01017271576669881265, 0.01464115812291478039, 0.01910960047913074986, 0.02134382165723873459, 0.02357804283534671586, 0.02804648519156268532, 0.03028070636967067006, 0.03251492754777865479, 0.03698336990399461732, 0.03921759108210259859, 0.04145181226021058679, 0.04368603343831857500, 0.04592025461642655626 ),
 ( 0.000000000000000000, 1.000000000000000000 ),
 .UNSPECIFIED. ) 
 GEOMETRIC_REPRESENTATION_ITEM ( )  RATIONAL_B_SPLINE_SURFACE ( (
 ( 1.000000000000000000, 0.7071067811865480168, 1.000000000000000000),
 ( 1.000000000000000000, 0.7196766872559550166, 1.000000000000000000),
 ( 1.000000000000000000, 0.7321324053393495346, 1.000000000000000000),
 ( 1.000000000000000000, 0.7567694315053145049, 1.000000000000000000),
 ( 1.000000000000000000, 0.7689510682428757349, 1.000000000000000000),
 ( 1.000000000000000000, 0.7869757430504373819, 1.000000000000000000),
 ( 1.000000000000000000, 0.7929631687995973843, 1.000000000000000000),
 ( 1.000000000000000000, 0.8046623649470893147, 1.000000000000000000),
 ( 1.000000000000000000, 0.8103917441617300987, 1.000000000000000000),
 ( 1.000000000000000000, 0.8272137286302455594, 1.000000000000000000),
 ( 1.000000000000000000, 0.8379439973090835325, 1.000000000000000000),
 ( 1.000000000000000000, 0.8532330560554255428, 1.000000000000000000),
 ( 1.000000000000000000, 0.8581942001721919455, 1.000000000000000000),
 ( 1.000000000000000000, 0.8678183107920264261, 1.000000000000000000),
 ( 1.000000000000000000, 0.8724301636766464974, 1.000000000000000000),
 ( 1.000000000000000000, 0.8855238771547766508, 1.000000000000000000),
 ( 1.000000000000000000, 0.8933247989485895157, 1.000000000000000000),
 ( 1.000000000000000000, 0.9033218449775582970, 1.000000000000000000),
 ( 1.000000000000000000, 0.9063188098299790330, 1.000000000000000000),
 ( 1.000000000000000000, 0.9115443529210249807, 1.000000000000000000),
 ( 1.000000000000000000, 0.9137831556782001208, 1.000000000000000000),
 ( 1.000000000000000000, 0.9174439670357630305, 1.000000000000000000),
 ( 1.000000000000000000, 0.9188661345744038034, 1.000000000000000000),
 ( 1.000000000000000000, 0.9207385544372965747, 1.000000000000000000),
 ( 1.000000000000000000, 0.9212071352555800674, 1.000000000000000000),
 ( 1.000000000000000000, 0.9212076576725564125, 1.000000000000000000) ) ) 
 REPRESENTATION_ITEM ( '' )  SURFACE ( )  );
#17502=DIRECTION ( 'NONE',  ( -0.000000000000000000, -1.000000000000000000, -0.000000000000000000 ) ) ;
#17506=CARTESIAN_POINT ( 'NONE',  ( 130.9868171408399746, -91.88282611735537841, 50.00000000000000000 ) ) ;
#17508=DIRECTION ( 'NONE',  ( -0.000000000000000000, -1.000000000000000000, -0.000000000000000000 ) ) ;
#17510=AXIS2_PLACEMENT_3D ( 'NONE', #2344, #7151, #16464 ) ;
#17515=CARTESIAN_POINT ( 'NONE',  ( 170.2125097089226529, -199.3942630591406839, 40.00000000000000000 ) ) ;
#17525=ORIENTED_EDGE ( 'NONE', *, *, #11382, .T. ) ;
#17536=CARTESIAN_POINT ( 'NONE',  ( 134.4038851132261243, -66.60439670040142346, 37.04366817629225039 ) ) ;
#17537=ADVANCED_FACE ( 'NONE', ( #11914 ), #18938, .F. ) ;
#17539=CARTESIAN_POINT ( 'NONE',  ( -136.0833144514123774, 32.93923414480397582, 28.34839128100539440 ) ) ;
#17540=CIRCLE ( 'NONE', #10319, 7.500000000000008882 ) ;
#17542=FACE_OUTER_BOUND ( 'NONE', #1664, .T. ) ;
#17544=DIRECTION ( 'NONE',  ( 1.000000000000000000, 0.000000000000000000, -0.000000000000000000 ) ) ;
#17549=ORIENTED_EDGE ( 'NONE', *, *, #13472, .T. ) ;
#17550=CIRCLE ( 'NONE', #18861, 7.500000000000007105 ) ;
#17558=DIRECTION ( 'NONE',  ( 0.000000000000000000, 0.000000000000000000, 1.000000000000000000 ) ) ;
#17559=CARTESIAN_POINT ( 'NONE',  ( -136.4994460260996902, -31.11111111111111782, -9.999999999999987566 ) ) ;
#17563=CARTESIAN_POINT ( 'NONE',  ( -135.1060089022256818, -65.16414933467417825, 30.00000000000000000 ) ) ;
#17568=CARTESIAN_POINT ( 'NONE',  ( 134.5351519296996798, -74.34771143809118144, 33.58511643466852092 ) ) ;
#17575=CARTESIAN_POINT ( 'NONE',  ( -176.7850001792984926, -190.0000000000000284, 33.42750952962406075 ) ) ;
#17577=DIRECTION ( 'NONE',  ( 0.000000000000000000, 0.000000000000000000, -1.000000000000000000 ) ) ;
#17582=CARTESIAN_POINT ( 'NONE',  ( 132.4400928985788539, -70.43137869103952653, -2.824645996396161873 ) ) ;
#17585=EDGE_LOOP ( 'NONE', ( #18200, #8671, #11556, #6096 ) ) ;
#17586=CIRCLE ( 'NONE', #18218, 7.500000000000020428 ) ;
#17587=FACE_OUTER_BOUND ( 'NONE', #7014, .T. ) ;
#17591=CARTESIAN_POINT ( 'NONE',  ( -176.1792632384392050, -186.5724904703759535, 10.00000000000000178 ) ) ;
#17592=CARTESIAN_POINT ( 'NONE',  ( -75.09489825810958052, 118.1556484538405414, 7.611160636458589757 ) ) ;
#17595=ORIENTED_EDGE ( 'NONE', *, *, #11395, .F. ) ;
#17599=VERTEX_POINT ( 'NONE', #15717 ) ;
#17607=AXIS2_PLACEMENT_3D ( 'NONE', #16559, #5810, #13673 ) ;
#17617=CARTESIAN_POINT ( 'NONE',  ( 96.82170812967342499, -114.6249810635733297, 36.57915001187932091 ) ) ;
#17619=EDGE_CURVE ( 'NONE', #3260, #15303, #14635, .T. ) ;
#17621=CARTESIAN_POINT ( 'NONE',  ( -83.84343328673659812, 124.3879646359026623, 35.30785401045157101 ) ) ;
#17632=PLANE ( 'NONE',  #12955 ) ;
#17636=CARTESIAN_POINT ( 'NONE',  ( -98.78543727592952450, -132.2400759706156066, 5.082541774034873505 ) ) ;
#17643=FACE_OUTER_BOUND ( 'NONE', #1168, .T. ) ;
#17647=CARTESIAN_POINT ( 'NONE',  ( -113.8386494799486712, 67.89548654814036865, -29.84279094000235233 ) ) ;
#17649=EDGE_CURVE ( 'NONE', #383, #1323, #2481, .T. ) ;
#17650=ORIENTED_EDGE ( 'NONE', *, *, #19375, .F. ) ;
#17652=VERTEX_POINT ( 'NONE', #8521 ) ;
#17668=CIRCLE ( 'NONE', #1655, 7.500000000000020428 ) ;
#17671=EDGE_CURVE ( 'NONE', #13051, #16478, #17586, .T. ) ;
#17675=DIRECTION ( 'NONE',  ( -1.000000000000000000, 0.000000000000000000, 0.000000000000000000 ) ) ;
#17678=DIRECTION ( 'NONE',  ( 0.000000000000000000, 1.000000000000000000, 0.000000000000000000 ) ) ;
#17683=CIRCLE ( 'NONE', #18984, 150.0000000000000284 ) ;
#17687=CARTESIAN_POINT ( 'NONE',  ( -103.3159608135122767, 96.92777072167388042, -34.47331703024818239 ) ) ;
#17694=CARTESIAN_POINT ( 'NONE',  ( 82.61717615486089983, -125.1974987762634299, 34.97368933229491716 ) ) ;
#17695=EDGE_LOOP ( 'NONE', ( #4363, #16140, #18825, #11894 ) ) ;
#17697=CARTESIAN_POINT ( 'NONE',  ( -110.0000000000000284, 101.9803902718557111, 44.99999999999998579 ) ) ;
#17713=DIRECTION ( 'NONE',  ( -0.2225209339563047894, -0.9749279121818258398, 0.000000000000000000 ) ) ;
#17714=CARTESIAN_POINT ( 'NONE',  ( 95.40880945838065941, -115.7543288757354105, -9.200166993891775391 ) ) ;
#17719=ORIENTED_EDGE ( 'NONE', *, *, #18646, .T. ) ;
#17721=ORIENTED_EDGE ( 'NONE', *, *, #19139, .T. ) ;
#17724=CARTESIAN_POINT ( 'NONE',  ( -125.3183776508946181, 82.47019060060657125, 41.98005522159012770 ) ) ;
#17725=VERTEX_POINT ( 'NONE', #8616 ) ;
#17729=CARTESIAN_POINT ( 'NONE',  ( -96.25554516485779288, -115.9717118653566388, 9.976009158364529839 ) ) ;
#17734=DIRECTION ( 'NONE',  ( -0.000000000000000000, 1.000000000000000000, -0.000000000000000000 ) ) ;
#17737=VECTOR ( 'NONE', #15594, 1000.000000000000114 ) ;
#17745=CARTESIAN_POINT ( 'NONE',  ( -129.2265855148631033, -76.16362387560155867, -7.281016149904609769 ) ) ;
#17751=CARTESIAN_POINT ( 'NONE',  ( -136.3148177136730794, -31.14249925903075678, -13.32260370553848539 ) ) ;
#17756=DIRECTION ( 'NONE',  ( -0.000000000000000000, 0.000000000000000000, -1.000000000000000000 ) ) ;
#17758=CARTESIAN_POINT ( 'NONE',  ( 98.17232476721000012, -133.0668712321317741, 33.62904428466136153 ) ) ;
#17761=AXIS2_PLACEMENT_3D ( 'NONE', #12266, #14009, #4605 ) ;
#17764=VERTEX_POINT ( 'NONE', #7573 ) ;
#17773=CARTESIAN_POINT ( 'NONE',  ( -166.7850001792984926, -200.0000000000000284, 40.00000000000000000 ) ) ;
#17777=DIRECTION ( 'NONE',  ( 0.000000000000000000, 0.000000000000000000, 1.000000000000000000 ) ) ;
#17781=CARTESIAN_POINT ( 'NONE',  ( -101.6560149856525612, 99.01817082827582794, -34.15757780977866531 ) ) ;
#17784=LINE ( 'NONE', #14507, #3525 ) ;
#17792=VERTEX_POINT ( 'NONE', #18745 ) ;
#17793=ORIENTED_EDGE ( 'NONE', *, *, #4503, .F. ) ;
#17797=CARTESIAN_POINT ( 'NONE',  ( -110.0000000000000142, 1.592040838891559450E-14, -49.99999999999999289 ) ) ;
#17810=CARTESIAN_POINT ( 'NONE',  ( 128.2779226595531270, 102.2982297021113141, 39.99999999999999289 ) ) ;
#17811=CARTESIAN_POINT ( 'NONE',  ( 87.10655032386927132, -147.8252249328912740, 39.99999999999999289 ) ) ;
#17813=CIRCLE ( 'NONE', #3747, 140.0000000000000000 ) ;
#17818=ORIENTED_EDGE ( 'NONE', *, *, #15149, .T. ) ;
#17823=CARTESIAN_POINT ( 'NONE',  ( 140.0000000000000000, 0.000000000000000000, 49.99999999999999289 ) ) ;
#17828=CARTESIAN_POINT ( 'NONE',  ( -96.53160196461145404, -115.8699919790248458, 10.20159961589317632 ) ) ;
#17830=CARTESIAN_POINT ( 'NONE',  ( -85.33507189799759374, -123.3618359587738240, -1.358392269459132162 ) ) ;
#17832=CARTESIAN_POINT ( 'NONE',  ( -107.4999999999999716, -118.5063289449133634, 50.00000000000000000 ) ) ;
#17836=AXIS2_PLACEMENT_3D ( 'NONE', #18178, #16739, #19702 ) ;
#17840=ORIENTED_EDGE ( 'NONE', *, *, #3016, .F. ) ;
#17842=DIRECTION ( 'NONE',  ( 0.2225209339563044841, 0.9749279121818258398, 0.000000000000000000 ) ) ;
#17843=CIRCLE ( 'NONE', #12938, 150.0000000000000284 ) ;
#17844=CARTESIAN_POINT ( 'NONE',  ( -133.7387326730402606, -67.93012127445986437, 0.4342299613749713849 ) ) ;
#17849=CARTESIAN_POINT ( 'NONE',  ( 128.2779226595531270, 102.2982297021113141, 39.99999999999999289 ) ) ;
#17850=CARTESIAN_POINT ( 'NONE',  ( -133.7753978164293756, -79.32938232250573662, 2.776447817717049737 ) ) ;
#17853=DIRECTION ( 'NONE',  ( -0.000000000000000000, -0.000000000000000000, 1.000000000000000000 ) ) ;
#17856=B_SPLINE_CURVE_WITH_KNOTS ( 'NONE', 3,
 ( #13466, #14915, #15019, #4174, #5817, #5419, #16756, #15113, #16368, #19527, #803, #2545, #12035, #10501, #8873, #5516, #7246, #2749, #19718, #3970, #17903, #902, #7154, #13372, #18298, #16566 ),
 .UNSPECIFIED., .F., .F.,
 ( 4, 2, 2, 2, 2, 2, 2, 2, 2, 2, 2, 2, 4 ),
 ( 0.000000000000000000, 0.004334419010351028140, 0.006501628515526520526, 0.008668838020702012911, 0.01300325703105300115, 0.01517046653622849614, 0.01733767604140399113, 0.02167209505175500192, 0.02383930455693049691, 0.02600651406210598496, 0.02817372356728147648, 0.03034093307245696453, 0.03467535208280796144 ),
 .UNSPECIFIED. ) ;
#17860=AXIS2_PLACEMENT_3D ( 'NONE', #19863, #17577, #1039 ) ;
#17861=ADVANCED_FACE ( 'NONE', ( #15354 ), #6166, .F. ) ;
#17868=ORIENTED_EDGE ( 'NONE', *, *, #19544, .F. ) ;
#17883=DIRECTION ( 'NONE',  ( 0.000000000000000000, -0.000000000000000000, -1.000000000000000000 ) ) ;
#17886=EDGE_LOOP ( 'NONE', ( #19613, #3573, #571, #10886 ) ) ;
#17895=DIRECTION ( 'NONE',  ( 0.000000000000000000, 0.000000000000000000, 1.000000000000000000 ) ) ;
#17897=CARTESIAN_POINT ( 'NONE',  ( -92.20932192393669879, -118.3126747524536313, 47.79843924115901643 ) ) ;
#17900=DIRECTION ( 'NONE',  ( 0.5742676632334706710, 0.8186676071302499968, 0.000000000000000000 ) ) ;
#17903=CARTESIAN_POINT ( 'NONE',  ( -134.3888575020695271, -66.63121209263866263, 37.00842455669916831 ) ) ;
#17910=CARTESIAN_POINT ( 'NONE',  ( 83.87053960371954986, -124.3614079552663299, 1.354181719470851419 ) ) ;
#17923=DIRECTION ( 'NONE',  ( -0.7818314824680221431, -0.6234898018587431423, -0.000000000000000000 ) ) ;
#17924=ADVANCED_FACE ( 'NONE', ( #3295 ), #1856, .T. ) ;
#17928=CARTESIAN_POINT ( 'NONE',  ( 95.64660831655231732, -115.7365562161967745, 5.860842583562486219 ) ) ;
#17929=CARTESIAN_POINT ( 'NONE',  ( -96.22303100966419720, -115.1714777947517803, 4.442967616989036195 ) ) ;
#17948=EDGE_CURVE ( 'NONE', #8819, #11868, #278, .T. ) ;
#17949=ORIENTED_EDGE ( 'NONE', *, *, #19008, .T. ) ;
#17950=CARTESIAN_POINT ( 'NONE',  ( 52.50000000000000711, 6.293851260911244545E-13, -105.0000000000000142 ) ) ;
#17954=CARTESIAN_POINT ( 'NONE',  ( -71.18887634719365565, -147.8252249328922687, 39.99999999999999289 ) ) ;
#17957=DIRECTION ( 'NONE',  ( -1.000000000000000000, 0.000000000000000000, 0.000000000000000000 ) ) ;
#17958=CARTESIAN_POINT ( 'NONE',  ( -130.6671641404174977, -73.67117004794211255, -5.709326280083561578 ) ) ;
#17961=DIRECTION ( 'NONE',  ( -0.000000000000000000, -1.000000000000000000, -0.000000000000000000 ) ) ;
#17970=CARTESIAN_POINT ( 'NONE',  ( 128.2779226595531270, 102.2982297021113141, 39.99999999999999289 ) ) ;
#17984=CARTESIAN_POINT ( 'NONE',  ( 0.000000000000000000, 0.000000000000000000, -49.99999999999999289 ) ) ;
#17985=CARTESIAN_POINT ( 'NONE',  ( 150.0000000000000284, 1.836970198721029747E-14, 49.99999999999999289 ) ) ;
#17995=FACE_OUTER_BOUND ( 'NONE', #15005, .T. ) ;
#18001=CARTESIAN_POINT ( 'NONE',  ( -107.4999999999999858, -118.5063289449133777, -10.00000000000000000 ) ) ;
#18009=CARTESIAN_POINT ( 'NONE',  ( 93.79892245610579948, -117.0565612855932329, -8.571526395727955716 ) ) ;
#18011=ORIENTED_EDGE ( 'NONE', *, *, #14038, .T. ) ;
#18012=CARTESIAN_POINT ( 'NONE',  ( -100.7812499999999716, -111.0996833858562809, 49.99999999999999289 ) ) ;
#18014=VERTEX_POINT ( 'NONE', #15876 ) ;
#18024=CARTESIAN_POINT ( 'NONE',  ( -85.70335357680858124, -123.1056148428088335, -1.893379215449441988 ) ) ;
#18028=( BOUNDED_CURVE ( )  B_SPLINE_CURVE ( 3, ( #14512, #12871, #14103, #11029 ),
 .UNSPECIFIED., .F., .F. ) 
 B_SPLINE_CURVE_WITH_KNOTS ( ( 4, 4 ),
 ( 3.141592653589794004, 4.712388980384689674 ),
 .UNSPECIFIED. ) 
 CURVE ( )  GEOMETRIC_REPRESENTATION_ITEM ( )  RATIONAL_B_SPLINE_CURVE ( ( 1.000000000000000000, 0.8047378541243652705, 0.8047378541243652705, 1.000000000000000000 ) ) 
 REPRESENTATION_ITEM ( '' )  );
#18030=DIRECTION ( 'NONE',  ( 0.000000000000000000, 0.000000000000000000, 1.000000000000000000 ) ) ;
#18031=DIRECTION ( 'NONE',  ( 0.000000000000000000, 0.000000000000000000, 1.000000000000000000 ) ) ;
#18043=CARTESIAN_POINT ( 'NONE',  ( 134.1070788506805513, -77.29467090009929109, 3.900409095995342135 ) ) ;
#18048=CARTESIAN_POINT ( 'NONE',  ( 110.0000000000000142, 0.000000000000000000, -39.99999999999999289 ) ) ;
#18049=LINE ( 'NONE', #16219, #10968 ) ;
#18050=CARTESIAN_POINT ( 'NONE',  ( 132.3553460543369908, -70.70324312373998055, 4.525982478036794099 ) ) ;
#18055=CARTESIAN_POINT ( 'NONE',  ( 0.000000000000000000, 0.000000000000000000, 50.00000000000000000 ) ) ;
#18056=EDGE_CURVE ( 'NONE', #18133, #2863, #4525, .T. ) ;
#18059=CIRCLE ( 'NONE', #17418, 140.0000000000000000 ) ;
#18061=VERTEX_POINT ( 'NONE', #13088 ) ;
#18062=ORIENTED_EDGE ( 'NONE', *, *, #7352, .T. ) ;
#18067=ORIENTED_EDGE ( 'NONE', *, *, #13785, .F. ) ;
#18069=PLANE ( 'NONE',  #16529 ) ;
#18071=VERTEX_POINT ( 'NONE', #16180 ) ;
#18078=CARTESIAN_POINT ( 'NONE',  ( 133.3574802752771404, -81.67441013337949585, 38.22103175428581778 ) ) ;
#18079=DIRECTION ( 'NONE',  ( 0.000000000000000000, 0.000000000000000000, 1.000000000000000000 ) ) ;
#18090=CARTESIAN_POINT ( 'NONE',  ( -93.26156191356919578, -117.4850166029420677, 48.33165481139338482 ) ) ;
#18093=VERTEX_POINT ( 'NONE', #18012 ) ;
#18098=DIRECTION ( 'NONE',  ( -0.9009688679024212554, 0.4338837391175534575, 0.000000000000000000 ) ) ;
#18102=CARTESIAN_POINT ( 'NONE',  ( 82.33470881469955316, -125.3834122142801277, 6.398087192529462897 ) ) ;
#18111=VECTOR ( 'NONE', #15868, 1000.000000000000000 ) ;
#18116=ORIENTED_EDGE ( 'NONE', *, *, #17671, .F. ) ;
#18120=CARTESIAN_POINT ( 'NONE',  ( -82.61717615486091404, -125.1974987762635152, 5.026310667705078394 ) ) ;
#18121=CARTESIAN_POINT ( 'NONE',  ( -110.0000000000000142, 1.530808498934191876E-14, -39.99999999999999289 ) ) ;
#18133=VERTEX_POINT ( 'NONE', #2457 ) ;
#18135=DIRECTION ( 'NONE',  ( 0.000000000000000000, 0.000000000000000000, 1.000000000000000000 ) ) ;
#18137=CARTESIAN_POINT ( 'NONE',  ( 134.3956174703911017, -75.35551001548425631, 5.362548286559334798 ) ) ;
#18140=CARTESIAN_POINT ( 'NONE',  ( 138.2024300533213932, 89.85329105948596862, 49.99999999999999289 ) ) ;
#18141=CARTESIAN_POINT ( 'NONE',  ( 4.189777606611760026E-13, -60.00000000000000000, -105.0000000000000142 ) ) ;
#18154=EDGE_CURVE ( 'NONE', #1847, #4859, #1010, .T. ) ;
#18155=EDGE_CURVE ( 'NONE', #16933, #870, #5186, .T. ) ;
#18156=ORIENTED_EDGE ( 'NONE', *, *, #8619, .F. ) ;
#18159=EDGE_CURVE ( 'NONE', #6447, #6551, #14926, .T. ) ;
#18169=CARTESIAN_POINT ( 'NONE',  ( -134.2328839869800277, -76.48032294689467392, 4.418921395648128581 ) ) ;
#18171=AXIS2_PLACEMENT_3D ( 'NONE', #7314, #15397, #12423 ) ;
#18172=VECTOR ( 'NONE', #9226, 1000.000000000000000 ) ;
#18176=B_SPLINE_CURVE_WITH_KNOTS ( 'NONE', 3,
 ( #8046, #6327, #14297, #3348, #11322, #4899, #8247, #11112, #3150, #19207, #7840, #17375, #9385, #4790, #9785, #15933, #12753, #12546, #19013, #7942, #15833, #15628, #1616, #9587 ),
 .UNSPECIFIED., .F., .F.,
 ( 4, 2, 2, 2, 2, 2, 2, 2, 2, 2, 2, 4 ),
 ( 0.000000000000000000, 0.005718059174761352254, 0.008577088762142017972, 0.01143611834952268543, 0.01286563314321301742, 0.01429514793690335114, 0.01715417752428397696, 0.01858369231797427773, 0.02001320711166457503, 0.02072796450850974623, 0.02144272190535492090, 0.02287223669904525289 ),
 .UNSPECIFIED. ) ;
#18178=CARTESIAN_POINT ( 'NONE',  ( 60.00000000000000711, 6.284666409917639535E-13, -105.0000000000000142 ) ) ;
#18180=EDGE_LOOP ( 'NONE', ( #8840, #14239, #324, #10418 ) ) ;
#18187=SURFACE_SIDE_STYLE ('',( #12337 ) ) ;
#18189=CARTESIAN_POINT ( 'NONE',  ( 15.91767397667355510, 149.1530343478547138, 49.99999999999999289 ) ) ;
#18200=ORIENTED_EDGE ( 'NONE', *, *, #592, .F. ) ;
#18206=AXIS2_PLACEMENT_3D ( 'NONE', #9082, #10715, #2959 ) ;
#18212=CARTESIAN_POINT ( 'NONE',  ( 97.52493780047066707, -113.9981091059116096, 2.471315604452407388 ) ) ;
#18215=CIRCLE ( 'NONE', #245, 15.91767397667354800 ) ;
#18217=CARTESIAN_POINT ( 'NONE',  ( -110.0000000000000142, 0.000000000000000000, -29.99999999999998224 ) ) ;
#18218=AXIS2_PLACEMENT_3D ( 'NONE', #13404, #10437, #5751 ) ;
#18221=DIRECTION ( 'NONE',  ( -0.6234898018587431423, 0.7818314824680221431, 0.000000000000000000 ) ) ;
#18229=VERTEX_POINT ( 'NONE', #7554 ) ;
#18233=LINE ( 'NONE', #12947, #13260 ) ;
#18234=EDGE_LOOP ( 'NONE', ( #19003, #2161, #16429, #2588 ) ) ;
#18235=CARTESIAN_POINT ( 'NONE',  ( 131.2498835542438655, -90.93927553429132615, -1.384616524445031067E-15 ) ) ;
#18237=CARTESIAN_POINT ( 'NONE',  ( -29.99999999999887379, 265.0000000000000000, 4.999999999999158007 ) ) ;
#18239=ORIENTED_EDGE ( 'NONE', *, *, #8275, .T. ) ;
#18241=CARTESIAN_POINT ( 'NONE',  ( -130.5346569919981334, -73.99347627471406952, 1.284038776032530249 ) ) ;
#18242=EDGE_CURVE ( 'NONE', #11033, #13701, #913, .T. ) ;
#18243=CARTESIAN_POINT ( 'NONE',  ( 130.9868171408399462, -91.88282611735540684, 0.000000000000000000 ) ) ;
#18245=CARTESIAN_POINT ( 'NONE',  ( -176.7850001792984926, -190.0000000000000284, 6.572490470375933036 ) ) ;
#18246=CARTESIAN_POINT ( 'NONE',  ( -148.9554720520393118, -17.67108784863417270, 49.99999999999999289 ) ) ;
#18247=CIRCLE ( 'NONE', #9085, 7.500000000000007105 ) ;
#18248=CYLINDRICAL_SURFACE ( 'NONE', #12897, 7.500000000000000000 ) ;
#18258=ORIENTED_EDGE ( 'NONE', *, *, #1752, .T. ) ;
#18261=CARTESIAN_POINT ( 'NONE',  ( -138.3191304882901420, -25.24048809540655469, 25.56945045193375776 ) ) ;
#18269=DIRECTION ( 'NONE',  ( 0.000000000000000000, 0.000000000000000000, 1.000000000000000000 ) ) ;
#18271=CARTESIAN_POINT ( 'NONE',  ( -133.6066233479225787, -80.29760051435191315, 2.337471363756875586 ) ) ;
#18272=ADVANCED_FACE ( 'NONE', ( #19829 ), #7353, .F. ) ;
#18274=DIRECTION ( 'NONE',  ( -0.4338837391175523472, -0.9009688679024219216, 0.000000000000000000 ) ) ;
#18275=EDGE_CURVE ( 'NONE', #13097, #16122, #14651, .T. ) ;
#18276=ADVANCED_FACE ( 'NONE', ( #1428 ), #12046, .F. ) ;
#18286=ADVANCED_FACE ( 'NONE', ( #10376 ), #781, .T. ) ;
#18288=ADVANCED_FACE ( 'NONE', ( #11713 ), #10285, .T. ) ;
#18293=DIRECTION ( 'NONE',  ( 0.000000000000000000, 0.000000000000000000, -1.000000000000000000 ) ) ;
#18298=CARTESIAN_POINT ( 'NONE',  ( -135.1060089022257102, -65.16414933467419246, 31.46482803569396935 ) ) ;
#18305=FACE_OUTER_BOUND ( 'NONE', #6262, .T. ) ;
#18309=DIRECTION ( 'NONE',  ( -0.000000000000000000, -0.000000000000000000, -1.000000000000000000 ) ) ;
#18316=ORIENTED_EDGE ( 'NONE', *, *, #15855, .F. ) ;
#18317=LINE ( 'NONE', #13390, #10751 ) ;
#18320=CARTESIAN_POINT ( 'NONE',  ( 101.4356266330684662, -128.4750511900865888, 2.021468608508339315 ) ) ;
#18324=CARTESIAN_POINT ( 'NONE',  ( 52.50000000000000711, 6.293851260911244545E-13, -105.0000000000000142 ) ) ;
#18335=ORIENTED_EDGE ( 'NONE', *, *, #3159, .T. ) ;
#18339=ORIENTED_EDGE ( 'NONE', *, *, #13126, .T. ) ;
#18341=CARTESIAN_POINT ( 'NONE',  ( 133.9068821628478929, -78.54443609883627175, 3.174243263777940083 ) ) ;
#18342=LINE ( 'NONE', #15062, #4873 ) ;
#18344=DIRECTION ( 'NONE',  ( -1.000000000000000000, 0.000000000000000000, 0.000000000000000000 ) ) ;
#18345=DIRECTION ( 'NONE',  ( 0.000000000000000000, 0.000000000000000000, 1.000000000000000000 ) ) ;
#18348=CARTESIAN_POINT ( 'NONE',  ( -135.1060089022256818, -65.16414933467422088, 10.00000000000000888 ) ) ;
#18349=CARTESIAN_POINT ( 'NONE',  ( 125.5405970674948719, -82.09774788367153064, -9.558221728786987725 ) ) ;
#18352=CARTESIAN_POINT ( 'NONE',  ( -134.7188131032333729, -72.93593548660994941, 30.00000000000000355 ) ) ;
#18355=CARTESIAN_POINT ( 'NONE',  ( 0.000000000000000000, 0.000000000000000000, 49.99999999999999289 ) ) ;
#18357=ORIENTED_EDGE ( 'NONE', *, *, #18646, .F. ) ;
#18359=EDGE_CURVE ( 'NONE', #2029, #14347, #1069, .T. ) ;
#18362=CARTESIAN_POINT ( 'NONE',  ( -139.9219061313053487, -21.70092091026256753, 23.17206116853662579 ) ) ;
#18364=FACE_OUTER_BOUND ( 'NONE', #5509, .T. ) ;
#18369=CARTESIAN_POINT ( 'NONE',  ( -78.37722339831623231, 116.0043570404596522, -9.999999999999984013 ) ) ;
#18374=CARTESIAN_POINT ( 'NONE',  ( -133.8332678793154003, -78.98710468785296257, 2.945529613542154923 ) ) ;
#18376=DIRECTION ( 'NONE',  ( -0.000000000000000000, 0.000000000000000000, -1.000000000000000000 ) ) ;
#18380=VERTEX_POINT ( 'NONE', #7317 ) ;
#18388=VERTEX_POINT ( 'NONE', #13243 ) ;
#18403=AXIS2_PLACEMENT_3D ( 'NONE', #6179, #30, #9442 ) ;
#18408=DIRECTION ( 'NONE',  ( -0.9009688679024160374, -0.4338837391175646707, 0.000000000000000000 ) ) ;
#18409=CARTESIAN_POINT ( 'NONE',  ( -81.19240997922189251, 114.0563236116805683, 24.94044186044488143 ) ) ;
#18422=EDGE_LOOP ( 'NONE', ( #5291, #7141, #14258, #18929 ) ) ;
#18423=AXIS2_PLACEMENT_3D ( 'NONE', #9379, #15624, #17675 ) ;
#18424=CARTESIAN_POINT ( 'NONE',  ( 84.61443574188869832, -123.8565353992718343, -0.1365201778679814570 ) ) ;
#18428=FACE_OUTER_BOUND ( 'NONE', #19126, .T. ) ;
#18433=CARTESIAN_POINT ( 'NONE',  ( 97.58443926496310894, -133.8443912861144725, 31.49252049683460442 ) ) ;
#18437=ORIENTED_EDGE ( 'NONE', *, *, #346, .T. ) ;
#18439=ORIENTED_EDGE ( 'NONE', *, *, #8667, .F. ) ;
#18444=DIRECTION ( 'NONE',  ( -0.000000000000000000, -0.000000000000000000, -1.000000000000000000 ) ) ;
#18445=CARTESIAN_POINT ( 'NONE',  ( -175.4992877478424873, -40.00000000000000000, -9.999999999999987566 ) ) ;
#18447=CYLINDRICAL_SURFACE ( 'NONE', #2569, 9.999999999999994671 ) ;
#18451=CARTESIAN_POINT ( 'NONE',  ( 134.3287459046948698, -75.81846210760082272, 4.971753820041441507 ) ) ;
#18454=CARTESIAN_POINT ( 'NONE',  ( -128.1750136849898638, -77.98139142652895828, 40.55909899233935079 ) ) ;
#18456=DIRECTION ( 'NONE',  ( 1.613511099790691498E-16, -1.000000000000000000, -0.000000000000000000 ) ) ;
#18459=AXIS2_PLACEMENT_3D ( 'NONE', #19823, #20239, #7547 ) ;
#18466=VECTOR ( 'NONE', #801, 1000.000000000000000 ) ;
#18467=CARTESIAN_POINT ( 'NONE',  ( -138.4146443278754646, -17.45363688215859810, -15.43852953348798707 ) ) ;
#18472=FACE_OUTER_BOUND ( 'NONE', #14762, .T. ) ;
#18476=CARTESIAN_POINT ( 'NONE',  ( 128.0922826834546413, -78.05640312850610485, 48.22554480681662170 ) ) ;
#18478=AXIS2_PLACEMENT_3D ( 'NONE', #14866, #8536, #5670 ) ;
#18481=ORIENTED_EDGE ( 'NONE', *, *, #3411, .T. ) ;
#18488=EDGE_LOOP ( 'NONE', ( #19736, #18335, #10594, #12483 ) ) ;
#18491=( NAMED_UNIT ( * ) PLANE_ANGLE_UNIT ( ) SI_UNIT ( $, .RADIAN. ) );
#18492=DIRECTION ( 'NONE',  ( -0.000000000000000000, -1.000000000000000000, -0.000000000000000000 ) ) ;
#18494=DIRECTION ( 'NONE',  ( -1.734723475976805615E-16, 3.205153653169784876E-16, -1.000000000000000000 ) ) ;
#18495=CARTESIAN_POINT ( 'NONE',  ( -7.500000000000001776, 60.00000000000000000, -105.0000000000000142 ) ) ;
#18496=AXIS2_PLACEMENT_3D ( 'NONE', #6852, #4639, #16171 ) ;
#18502=EDGE_CURVE ( 'NONE', #5679, #3424, #14910, .T. ) ;
#18505=CARTESIAN_POINT ( 'NONE',  ( -134.4452567384424526, -75.00213249385289771, 34.30395834063391902 ) ) ;
#18521=CARTESIAN_POINT ( 'NONE',  ( 98.78819505924182920, -132.2357222602873321, 5.087113913613924510 ) ) ;
#18523=CARTESIAN_POINT ( 'NONE',  ( -141.6670309912509822, -18.66040293829161811, -9.999999999999985789 ) ) ;
#18525=FACE_BOUND ( 'NONE', #1249, .T. ) ;
#18526=CARTESIAN_POINT ( 'NONE',  ( 134.1130761623740568, -69.50842595698583182, 10.00000000000000178 ) ) ;
#18529=EDGE_CURVE ( 'NONE', #13158, #6900, #6608, .T. ) ;
#18531=CARTESIAN_POINT ( 'NONE',  ( 86.68385341650764531, -122.4206889339569528, 43.25796838106919751 ) ) ;
#18535=AXIS2_PLACEMENT_3D ( 'NONE', #16050, #7036, #2135 ) ;
#18553=DIRECTION ( 'NONE',  ( 0.9009688679024158153, 0.4338837391175651703, 0.000000000000000000 ) ) ;
#18555=CARTESIAN_POINT ( 'NONE',  ( -133.2542153457957284, -68.87904111072103319, -0.9529167680878568580 ) ) ;
#18556=CARTESIAN_POINT ( 'NONE',  ( 133.3512892972266854, -81.69145041114401806, 1.787651230699585758 ) ) ;
#18560=CARTESIAN_POINT ( 'NONE',  ( -125.9179923520565865, -81.51769904231002783, 49.42145388281251428 ) ) ;
#18566=VERTEX_POINT ( 'NONE', #353 ) ;
#18567=ORIENTED_EDGE ( 'NONE', *, *, #14038, .F. ) ;
#18577=VECTOR ( 'NONE', #8679, 1000.000000000000000 ) ;
#18582=CARTESIAN_POINT ( 'NONE',  ( 175.7155416004667643, -197.3864744618499856, -6.936210497111005848E-15 ) ) ;
#18591=VECTOR ( 'NONE', #5898, 1000.000000000000000 ) ;
#18610=DIRECTION ( 'NONE',  ( -1.000000000000000000, -1.613511099790693471E-16, 0.000000000000000000 ) ) ;
#18612=CARTESIAN_POINT ( 'NONE',  ( -134.5748517645101856, -74.05062141148572152, 33.20438510682525646 ) ) ;
#18613=CARTESIAN_POINT ( 'NONE',  ( -78.74873325666423796, 115.7553402848426316, 20.84531035572755897 ) ) ;
#18616=ADVANCED_FACE ( 'NONE', ( #19190 ), #3633, .F. ) ;
#18617=CARTESIAN_POINT ( 'NONE',  ( 144.1130761623740568, -69.50842595698583182, 49.99999999999999289 ) ) ;
#18619=ORIENTED_EDGE ( 'NONE', *, *, #10414, .T. ) ;
#18621=EDGE_LOOP ( 'NONE', ( #8690, #2218 ) ) ;
#18624=AXIS2_PLACEMENT_3D ( 'NONE', #14908, #10299, #2342 ) ;
#18631=CARTESIAN_POINT ( 'NONE',  ( 95.76651288690072761, -116.1232671447739051, 9.237827461556257447 ) ) ;
#18639=AXIS2_PLACEMENT_3D ( 'NONE', #8416, #18031, #13500 ) ;
#18643=CARTESIAN_POINT ( 'NONE',  ( 92.41621553528273125, -118.1510961661374637, 47.90971605349847096 ) ) ;
#18646=EDGE_CURVE ( 'NONE', #11485, #11258, #16955, .T. ) ;
#18648=CARTESIAN_POINT ( 'NONE',  ( 52.50000000000000711, 6.293851260911244545E-13, -100.0000000000000000 ) ) ;
#18649=VERTEX_POINT ( 'NONE', #18048 ) ;
#18652=CARTESIAN_POINT ( 'NONE',  ( -102.6608643076872767, -126.6195776799898312, 1.231354163479371433 ) ) ;
#18655=ADVANCED_FACE ( 'NONE', ( #2601 ), #7295, .F. ) ;
#18657=CARTESIAN_POINT ( 'NONE',  ( 97.50000000000001421, -133.9542832461881119, 1.387778780781445676E-14 ) ) ;
#18660=ADVANCED_FACE ( 'NONE', ( #8829 ), #3727, .F. ) ;
#18662=CARTESIAN_POINT ( 'NONE',  ( -90.38423273153478021, -119.7175801288912851, 46.68965822980387514 ) ) ;
#18663=DIRECTION ( 'NONE',  ( -0.000000000000000000, -0.000000000000000000, 1.000000000000000000 ) ) ;
#18667=CARTESIAN_POINT ( 'NONE',  ( 131.5402663983728360, -89.84204999195762298, 0.05619734976503784618 ) ) ;
#18670=CARTESIAN_POINT ( 'NONE',  ( -133.9275976130222432, -67.55320356804372750, 38.83589090172372238 ) ) ;
#18671=ORIENTED_EDGE ( 'NONE', *, *, #14144, .T. ) ;
#18672=CIRCLE ( 'NONE', #11774, 10.00000000000000533 ) ;
#18676=ORIENTED_EDGE ( 'NONE', *, *, #6758, .T. ) ;
#18678=AXIS2_PLACEMENT_3D ( 'NONE', #12814, #8212, #14457 ) ;
#18680=EDGE_CURVE ( 'NONE', #4551, #5660, #5566, .T. ) ;
#18688=CARTESIAN_POINT ( 'NONE',  ( -105.2523856663880366, 80.72709874070729086, -29.68324780735369472 ) ) ;
#18690=CARTESIAN_POINT ( 'NONE',  ( 178.1870518357301023, -192.0755223619200081, 4.142135623730942129 ) ) ;
#18699=DIRECTION ( 'NONE',  ( -1.000000000000000000, 0.000000000000000000, 0.000000000000000000 ) ) ;
#18701=EDGE_LOOP ( 'NONE', ( #18116, #13301 ) ) ;
#18705=CARTESIAN_POINT ( 'NONE',  ( 135.7779226595531270, 102.2982297021113141, 39.99999999999999289 ) ) ;
#18708=DIRECTION ( 'NONE',  ( 0.000000000000000000, 0.000000000000000000, 1.000000000000000000 ) ) ;
#18711=CARTESIAN_POINT ( 'NONE',  ( -73.97516692619829826, 130.4256996493784015, -12.43080227311476449 ) ) ;
#18712=CARTESIAN_POINT ( 'NONE',  ( -86.01343624116279329, 31.38211805825948630, 30.00000000000000000 ) ) ;
#18713=DIRECTION ( 'NONE',  ( -1.613511099790691498E-16, 1.000000000000000000, 0.000000000000000000 ) ) ;
#18718=CARTESIAN_POINT ( 'NONE',  ( -90.12511548116496840, 107.1354966152653390, 33.81810546212673785 ) ) ;
#18724=CARTESIAN_POINT ( 'NONE',  ( 75.91068486117727332, -120.9436655338208340, 39.99999999999999289 ) ) ;
#18726=CARTESIAN_POINT ( 'NONE',  ( -71.18887634719365565, -147.8252249328922687, 49.99999999999999289 ) ) ;
#18729=ORIENTED_EDGE ( 'NONE', *, *, #10587, .T. ) ;
#18730=AXIS2_PLACEMENT_3D ( 'NONE', #808, #16275, #19143 ) ;
#18731=CARTESIAN_POINT ( 'NONE',  ( 97.47038759843226785, -115.4903015188358495, 10.15380083008228596 ) ) ;
#18733=ADVANCED_FACE ( 'NONE', ( #10353 ), #16614, .T. ) ;
#18742=CARTESIAN_POINT ( 'NONE',  ( 102.7654166546833210, -126.4532151214411186, 38.81363406805538574 ) ) ;
#18745=CARTESIAN_POINT ( 'NONE',  ( -79.05640494597939494, -127.4758205975444412, 49.99999999999999289 ) ) ;
#18746=CARTESIAN_POINT ( 'NONE',  ( 0.000000000000000000, 164.0736214083062805, 49.99999999999999289 ) ) ;
#18759=CYLINDRICAL_SURFACE ( 'NONE', #18403, 7.500000000000007105 ) ;
#18761=CARTESIAN_POINT ( 'NONE',  ( -82.03125000082627594, -125.5821405427617066, 8.489866645478734597 ) ) ;
#18763=CARTESIAN_POINT ( 'NONE',  ( -84.12762954502584023, -124.1876770196617343, 39.19636848888279701 ) ) ;
#18764=DIRECTION ( 'NONE',  ( -1.613511099790691498E-16, 1.000000000000000000, -0.000000000000000000 ) ) ;
#18765=CARTESIAN_POINT ( 'NONE',  ( -139.1630865236926695, 15.78015590158507031, 24.36223180621681195 ) ) ;
#18770=CARTESIAN_POINT ( 'NONE',  ( -124.7133609680327311, -83.36099555805665773, 40.87838703930916751 ) ) ;
#18777=EDGE_LOOP ( 'NONE', ( #6299, #2912, #3172, #10077 ) ) ;
#18781=CARTESIAN_POINT ( 'NONE',  ( -142.1121543937410081, -17.96810325432989686, 18.92822252394145011 ) ) ;
#18788=CARTESIAN_POINT ( 'NONE',  ( -167.4599531637108782, -36.50981547337168109, 39.99999999999999289 ) ) ;
#18794=CARTESIAN_POINT ( 'NONE',  ( 131.5110516633172040, -72.14693729182981485, 44.44710436446363389 ) ) ;
#18795=AXIS2_PLACEMENT_3D ( 'NONE', #3881, #5617, #18098 ) ;
#18797=ADVANCED_FACE ( 'NONE', ( #12298 ), #15169, .F. ) ;
#18813=ORIENTED_EDGE ( 'NONE', *, *, #9760, .F. ) ;
#18814=CARTESIAN_POINT ( 'NONE',  ( 122.8001410695374602, -86.14014948502067170, -10.00000000000000178 ) ) ;
#18816=EDGE_LOOP ( 'NONE', ( #4527, #18619, #7485, #6863 ) ) ;
#18817=( BOUNDED_SURFACE ( )  B_SPLINE_SURFACE ( 3, 2, ( 
 ( #5775, #5879, #18352 ),
 ( #10360, #1052, #12201 ),
 ( #5980, #11793, #15174 ),
 ( #15072, #16522, #4329 ),
 ( #2502, #11890, #11991 ),
 ( #16817, #13737, #3664 ),
 ( #9898, #13325, #19581 ),
 ( #17234, #12410, #1369 ),
 ( #18872, #13841, #2910 ),
 ( #18670, #10666, #6493 ),
 ( #15698, #13944, #1471 ),
 ( #17129, #20189, #6192 ),
 ( #7702, #14053, #9138 ),
 ( #10873, #1780, #14257 ),
 ( #7599, #15379, #3318 ),
 ( #20084, #10975, #8011 ),
 ( #9554, #1576, #42 ),
 ( #15799, #4647, #6392 ),
 ( #17342, #3115, #16921 ),
 ( #4752, #6293, #240 ),
 ( #6084, #18454, #9345 ),
 ( #15592, #1680, #7811 ),
 ( #12507, #11078, #4437 ),
 ( #12302, #15487, #3213 ),
 ( #9454, #4542, #3012 ),
 ( #18560, #17026, #9244 ),
 ( #10773, #18770, #7907 ),
 ( #14154, #140, #12610 ),
 ( #4857, #14659, #16203 ),
 ( #1878, #2190, #16099 ) ),
 .UNSPECIFIED., .F., .F., .F. ) 
 B_SPLINE_SURFACE_WITH_KNOTS ( ( 4, 2, 2, 2, 2, 2, 2, 2, 2, 2, 2, 2, 2, 2, 4 ),
 ( 3, 3 ),
 ( 0.01087485647533277880, 0.01538493460406631895, 0.01651245413624970529, 0.01763997366843308989, 0.01989501273279985910, 0.02102253226498324370, 0.02215005179716662831, 0.02440509086153340099, 0.02891516899026694287, 0.03117020805463371208, 0.03342524711900048129, 0.03793532524773401970, 0.04019036431210078891, 0.04244540337646755812, 0.04695548150520110348 ),
 ( 0.000000000000000000, 1.000000000000000000 ),
 .UNSPECIFIED. ) 
 GEOMETRIC_REPRESENTATION_ITEM ( )  RATIONAL_B_SPLINE_SURFACE ( (
 ( 1.000000000000000000, 0.9212076576725557464, 1.000000000000000000),
 ( 1.000000000000000000, 0.9211983545445763255, 1.000000000000000000),
 ( 1.000000000000000000, 0.9192884530626878048, 1.000000000000000000),
 ( 1.000000000000000000, 0.9147257148664106330, 1.000000000000000000),
 ( 1.000000000000000000, 0.9137002753874979843, 1.000000000000000000),
 ( 1.000000000000000000, 0.9114460110780681079, 1.000000000000000000),
 ( 1.000000000000000000, 0.9102239901659594512, 1.000000000000000000),
 ( 1.000000000000000000, 0.9062907615861804933, 1.000000000000000000),
 ( 1.000000000000000000, 0.9033134084428574573, 1.000000000000000000),
 ( 1.000000000000000000, 0.8983619464026600943, 1.000000000000000000),
 ( 1.000000000000000000, 0.8966302762932344406, 1.000000000000000000),
 ( 1.000000000000000000, 0.8930095736512829729, 1.000000000000000000),
 ( 1.000000000000000000, 0.8911146393079628636, 1.000000000000000000),
 ( 1.000000000000000000, 0.8852539528816872894, 1.000000000000000000),
 ( 1.000000000000000000, 0.8811119717501607607, 1.000000000000000000),
 ( 1.000000000000000000, 0.8680569459629184914, 1.000000000000000000),
 ( 1.000000000000000000, 0.8585210289499386471, 1.000000000000000000),
 ( 1.000000000000000000, 0.8431029601255346506, 1.000000000000000000),
 ( 1.000000000000000000, 0.8377859708359541857, 1.000000000000000000),
 ( 1.000000000000000000, 0.8269824639699362434, 1.000000000000000000),
 ( 1.000000000000000000, 0.8214732595401645909, 1.000000000000000000),
 ( 1.000000000000000000, 0.8046428831057845787, 1.000000000000000000),
 ( 1.000000000000000000, 0.7930208592507520526, 1.000000000000000000),
 ( 1.000000000000000000, 0.7750195416465174292, 1.000000000000000000),
 ( 1.000000000000000000, 0.7688986879966103194, 1.000000000000000000),
 ( 1.000000000000000000, 0.7566232400044657913, 1.000000000000000000),
 ( 1.000000000000000000, 0.7504663834238096687, 1.000000000000000000),
 ( 1.000000000000000000, 0.7319497228662610322, 1.000000000000000000),
 ( 1.000000000000000000, 0.7195437534939763680, 1.000000000000000000),
 ( 1.000000000000000000, 0.7071067811865474617, 1.000000000000000000) ) ) 
 REPRESENTATION_ITEM ( '' )  SURFACE ( )  );
#18821=DIRECTION ( 'NONE',  ( 0.000000000000000000, 0.000000000000000000, 1.000000000000000000 ) ) ;
#18824=CARTESIAN_POINT ( 'NONE',  ( 85.33507189799762216, -123.3618359587737672, 41.35839226945913794 ) ) ;
#18825=ORIENTED_EDGE ( 'NONE', *, *, #4389, .F. ) ;
#18830=CARTESIAN_POINT ( 'NONE',  ( 0.000000000000000000, 0.000000000000000000, -9.999999999999994671 ) ) ;
#18831=ORIENTED_EDGE ( 'NONE', *, *, #10357, .T. ) ;
#18833=CARTESIAN_POINT ( 'NONE',  ( -133.9520938386737043, 58.56720361986037915, -27.05300300615894571 ) ) ;
#18834=CARTESIAN_POINT ( 'NONE',  ( -71.18887634719365565, -147.8252249328922687, 39.99999999999999289 ) ) ;
#18836=CARTESIAN_POINT ( 'NONE',  ( 99.15486248080401310, -131.7338018236151527, 4.478766899919759403 ) ) ;
#18841=ORIENTED_EDGE ( 'NONE', *, *, #7746, .F. ) ;
#18844=CARTESIAN_POINT ( 'NONE',  ( -50.37374754117254838, -141.2886604036510505, 49.99999999999999289 ) ) ;
#18845=CARTESIAN_POINT ( 'NONE',  ( 96.93610878393036501, -115.7104363121800077, 29.64800143911388020 ) ) ;
#18848=CARTESIAN_POINT ( 'NONE',  ( -77.10567499969560856, 128.6696624883277309, 27.82549893712029387 ) ) ;
#18853=ORIENTED_EDGE ( 'NONE', *, *, #9894, .F. ) ;
#18855=CARTESIAN_POINT ( 'NONE',  ( -104.1536737562094288, -124.2508859553632306, 0.5727794066519206195 ) ) ;
#18860=CARTESIAN_POINT ( 'NONE',  ( 126.0064496073183307, -81.39031533630308957, 49.41728923137324614 ) ) ;
#18861=AXIS2_PLACEMENT_3D ( 'NONE', #5103, #11433, #11331 ) ;
#18864=CARTESIAN_POINT ( 'NONE',  ( -99.76899065921458032, -130.8788316638204492, 36.35208880440197277 ) ) ;
#18865=CARTESIAN_POINT ( 'NONE',  ( 0.000000000000000000, 0.000000000000000000, 49.99999999999999289 ) ) ;
#18866=CARTESIAN_POINT ( 'NONE',  ( -140.0000000000000568, 2.005623917688350133, 23.02775637731988212 ) ) ;
#18872=CARTESIAN_POINT ( 'NONE',  ( -134.1858200530606950, -67.03963421359212305, 37.88757044792966866 ) ) ;
#18876=ORIENTED_EDGE ( 'NONE', *, *, #19857, .F. ) ;
#18877=VECTOR ( 'NONE', #18492, 1000.000000000000000 ) ;
#18878=ORIENTED_EDGE ( 'NONE', *, *, #8373, .F. ) ;
#18882=CARTESIAN_POINT ( 'NONE',  ( -143.8108380990476576, -15.58935400314438446, -4.058802881218986691 ) ) ;
#18884=EDGE_CURVE ( 'NONE', #269, #11053, #19601, .T. ) ;
#18887=ORIENTED_EDGE ( 'NONE', *, *, #6004, .T. ) ;
#18891=CARTESIAN_POINT ( 'NONE',  ( 71.18887634719571622, -147.8252249328912740, 49.99999999999999289 ) ) ;
#18897=CARTESIAN_POINT ( 'NONE',  ( 133.2712073792189074, -68.96827650324327408, 30.52894171284383873 ) ) ;
#18915=DIRECTION ( 'NONE',  ( -0.000000000000000000, -0.000000000000000000, 1.000000000000000000 ) ) ;
#18916=EDGE_CURVE ( 'NONE', #17599, #19010, #5901, .T. ) ;
#18921=CYLINDRICAL_SURFACE ( 'NONE', #16951, 9.999999999999996447 ) ;
#18925=CARTESIAN_POINT ( 'NONE',  ( -100.7812499999999716, -111.0996833858562809, -10.00000000000000178 ) ) ;
#18926=CARTESIAN_POINT ( 'NONE',  ( -76.32814421828534535, 117.3631207639434564, -4.586678902943767788 ) ) ;
#18929=ORIENTED_EDGE ( 'NONE', *, *, #15534, .F. ) ;
#18930=AXIS2_PLACEMENT_3D ( 'NONE', #8983, #15436, #4286 ) ;
#18933=ORIENTED_EDGE ( 'NONE', *, *, #740, .T. ) ;
#18935=DIRECTION ( 'NONE',  ( 0.9009688679024157043, 0.4338837391175651703, -0.000000000000000000 ) ) ;
#18936=ORIENTED_EDGE ( 'NONE', *, *, #84, .T. ) ;
#18937=CIRCLE ( 'NONE', #1275, 150.0000000000000284 ) ;
#18938=( BOUNDED_SURFACE ( )  B_SPLINE_SURFACE ( 3, 2, ( 
 ( #19699, #5906, #6006 ),
 ( #13865, #2528, #1394 ),
 ( #8755, #13659, #13764 ),
 ( #4355, #7624, #10483 ),
 ( #16736, #1178, #19905 ),
 ( #10583, #2831, #5696 ),
 ( #18476, #16643, #2631 ),
 ( #4458, #8855, #20107 ),
 ( #10690, #7321, #15093 ),
 ( #9164, #11810, #18078 ),
 ( #1075, #13553, #19802 ),
 ( #18794, #9674, #1904 ),
 ( #10897, #13968, #12432 ),
 ( #7830, #1803, #7727 ),
 ( #4674, #17157, #63 ),
 ( #1498, #164, #265 ),
 ( #8138, #17051, #15921 ),
 ( #4566, #1699, #3336 ),
 ( #12638, #14385, #4778 ),
 ( #7930, #14283, #10998 ),
 ( #11202, #12533, #9576 ),
 ( #4885, #6519, #17258 ),
 ( #9271, #6315, #3236 ),
 ( #14182, #6108, #11099 ),
 ( #6214, #18897, #14075 ),
 ( #15822, #9476, #4982 ) ),
 .UNSPECIFIED., .F., .F., .F. ) 
 B_SPLINE_SURFACE_WITH_KNOTS ( ( 4, 2, 2, 2, 2, 2, 2, 2, 2, 2, 2, 2, 4 ),
 ( 3, 3 ),
 ( 0.01017271576669884214, 0.01464115812291480467, 0.01910960047913076720, 0.02134382165723874847, 0.02357804283534672973, 0.02804648519156269226, 0.03028070636967067353, 0.03251492754777865479, 0.03698336990399461732, 0.03921759108210259859, 0.04145181226021057985, 0.04368603343831856112, 0.04592025461642654238 ),
 ( 0.000000000000000000, 1.000000000000000000 ),
 .UNSPECIFIED. ) 
 GEOMETRIC_REPRESENTATION_ITEM ( )  RATIONAL_B_SPLINE_SURFACE ( (
 ( 1.000000000000000000, 0.7071067811865480168, 1.000000000000000000),
 ( 1.000000000000000000, 0.7196766872558925110, 1.000000000000000000),
 ( 1.000000000000000000, 0.7321324053394322462, 1.000000000000000000),
 ( 1.000000000000000000, 0.7567694315052313492, 1.000000000000000000),
 ( 1.000000000000000000, 0.7689510682427085353, 1.000000000000000000),
 ( 1.000000000000000000, 0.7869757430505208706, 1.000000000000000000),
 ( 1.000000000000000000, 0.7929631687998897061, 1.000000000000000000),
 ( 1.000000000000000000, 0.8046623649467963268, 1.000000000000000000),
 ( 1.000000000000000000, 0.8103917441616884654, 1.000000000000000000),
 ( 1.000000000000000000, 0.8272137286303282711, 1.000000000000000000),
 ( 1.000000000000000000, 0.8379439973090003768, 1.000000000000000000),
 ( 1.000000000000000000, 0.8532330560554670651, 1.000000000000000000),
 ( 1.000000000000000000, 0.8581942001722338009, 1.000000000000000000),
 ( 1.000000000000000000, 0.8678183107919841266, 1.000000000000000000),
 ( 1.000000000000000000, 0.8724301636763960310, 1.000000000000000000),
 ( 1.000000000000000000, 0.8855238771552775834, 1.000000000000000000),
 ( 1.000000000000000000, 0.8933247989484205398, 1.000000000000000000),
 ( 1.000000000000000000, 0.9033218449776424519, 1.000000000000000000),
 ( 1.000000000000000000, 0.9063188098300211104, 1.000000000000000000),
 ( 1.000000000000000000, 0.9115443529209835694, 1.000000000000000000),
 ( 1.000000000000000000, 0.9137831556780738884, 1.000000000000000000),
 ( 1.000000000000000000, 0.9174439670358883747, 1.000000000000000000),
 ( 1.000000000000000000, 0.9188661345742781261, 1.000000000000000000),
 ( 1.000000000000000000, 0.9207385544374218078, 1.000000000000000000),
 ( 1.000000000000000000, 0.9212071352554866976, 1.000000000000000000),
 ( 1.000000000000000000, 0.9212076576725557464, 1.000000000000000000) ) ) 
 REPRESENTATION_ITEM ( '' )  SURFACE ( )  );
#18942=EDGE_CURVE ( 'NONE', #9222, #4680, #7553, .T. ) ;
#18946=ADVANCED_FACE ( 'NONE', ( #6689 ), #12500, .T. ) ;
#18947=CARTESIAN_POINT ( 'NONE',  ( 0.000000000000000000, 0.000000000000000000, 40.00000000000000000 ) ) ;
#18949=ORIENTED_EDGE ( 'NONE', *, *, #19375, .T. ) ;
#18953=CARTESIAN_POINT ( 'NONE',  ( 103.0386482854799652, -126.0278359105729606, 38.95485802678353338 ) ) ;
#18956=CARTESIAN_POINT ( 'NONE',  ( -69.98969223978424736, 132.6704322134999074, 5.046636793514642783 ) ) ;
#18964=CARTESIAN_POINT ( 'NONE',  ( -148.0038354016025437, 24.49305880778362976, 17.53332955362975909 ) ) ;
#18969=CARTESIAN_POINT ( 'NONE',  ( -96.32595581636883253, -115.9457815549233572, 29.96624877859731484 ) ) ;
#18972=CARTESIAN_POINT ( 'NONE',  ( 101.0196388379316659, 100.9199429146863167, 39.99999999999999289 ) ) ;
#18973=DIRECTION ( 'NONE',  ( -1.000000000000000000, 0.000000000000000000, 0.000000000000000000 ) ) ;
#18978=CARTESIAN_POINT ( 'NONE',  ( -60.00000000000000000, -2.094888803305880013E-13, -100.0000000000000000 ) ) ;
#18979=ORIENTED_EDGE ( 'NONE', *, *, #19423, .F. ) ;
#18980=CARTESIAN_POINT ( 'NONE',  ( -124.6317628381421088, 51.51696891155003044, -26.79866528532224734 ) ) ;
#18982=CARTESIAN_POINT ( 'NONE',  ( -181.0783081749256382, -200.0000000000000284, 40.00000000000000000 ) ) ;
#18983=ORIENTED_EDGE ( 'NONE', *, *, #4244, .T. ) ;
#18984=AXIS2_PLACEMENT_3D ( 'NONE', #9573, #8231, #8331 ) ;
#18987=CARTESIAN_POINT ( 'NONE',  ( -141.6227766016837961, -18.73072656238141320, -9.999999999999985789 ) ) ;
#18990=DIRECTION ( 'NONE',  ( -0.000000000000000000, -0.000000000000000000, 1.000000000000000000 ) ) ;
#18994=DIRECTION ( 'NONE',  ( 0.6234898018587442525, -0.7818314824680211439, 0.000000000000000000 ) ) ;
#18996=CARTESIAN_POINT ( 'NONE',  ( 99.98080768883885128, -130.5801677638304739, 36.60139651180438847 ) ) ;
#18997=VECTOR ( 'NONE', #15070, 1000.000000000000000 ) ;
#19001=CARTESIAN_POINT ( 'NONE',  ( 134.7188131032333445, -72.93593548660993520, 30.00000000000000000 ) ) ;
#19003=ORIENTED_EDGE ( 'NONE', *, *, #3523, .T. ) ;
#19004=ADVANCED_FACE ( 'NONE', ( #7806 ), #16094, .T. ) ;
#19006=EDGE_CURVE ( 'NONE', #17276, #15881, #6598, .T. ) ;
#19008=EDGE_CURVE ( 'NONE', #7363, #22, #17348, .T. ) ;
#19010=VERTEX_POINT ( 'NONE', #19648 ) ;
#19013=CARTESIAN_POINT ( 'NONE',  ( -97.77735676332854098, -133.5903492488113784, 32.35039215209604890 ) ) ;
#19019=EDGE_CURVE ( 'NONE', #16017, #9870, #6789, .T. ) ;
#19023=DIRECTION ( 'NONE',  ( 0.9009688679024218105, -0.4338837391175526248, 0.000000000000000000 ) ) ;
#19025=FACE_OUTER_BOUND ( 'NONE', #14448, .T. ) ;
#19026=CARTESIAN_POINT ( 'NONE',  ( 82.17818763663345294, -125.4865065810072622, 32.87940362201754851 ) ) ;
#19032=VERTEX_POINT ( 'NONE', #3997 ) ;
#19033=EDGE_CURVE ( 'NONE', #2972, #6720, #13292, .T. ) ;
#19035=DIRECTION ( 'NONE',  ( 0.000000000000000000, 0.000000000000000000, 1.000000000000000000 ) ) ;
#19037=DIRECTION ( 'NONE',  ( 1.000000000000000000, 0.000000000000000000, 0.000000000000000000 ) ) ;
#19039=ORIENTED_EDGE ( 'NONE', *, *, #16109, .T. ) ;
#19050=CARTESIAN_POINT ( 'NONE',  ( 0.000000000000000000, 0.000000000000000000, -9.999999999999994671 ) ) ;
#19056=DIRECTION ( 'NONE',  ( 1.000000000000000000, 0.000000000000000000, 0.000000000000000000 ) ) ;
#19059=EDGE_CURVE ( 'NONE', #4416, #9222, #17328, .T. ) ;
#19063=VECTOR ( 'NONE', #8397, 1000.000000000000000 ) ;
#19064=AXIS2_PLACEMENT_3D ( 'NONE', #3589, #11457, #14530 ) ;
#19067=CARTESIAN_POINT ( 'NONE',  ( -123.2437450313144893, 85.51307700781502774, 42.75112597072239851 ) ) ;
#19068=EDGE_LOOP ( 'NONE', ( #13007, #11242, #19832, #1327 ) ) ;
#19070=DIRECTION ( 'NONE',  ( 0.000000000000000000, 0.000000000000000000, 1.000000000000000000 ) ) ;
#19072=CARTESIAN_POINT ( 'NONE',  ( 129.2265855148630749, -76.16362387560154446, 47.28101614990461599 ) ) ;
#19073=CARTESIAN_POINT ( 'NONE',  ( -114.7901495840402077, 80.24275698007728863, 39.74168176665586572 ) ) ;
#19078=PLANE ( 'NONE',  #7675 ) ;
#19080=CARTESIAN_POINT ( 'NONE',  ( -109.9999999999874376, 73.61623156955475622, -29.99999999999998579 ) ) ;
#19082=ORIENTED_EDGE ( 'NONE', *, *, #16730, .T. ) ;
#19091=LINE ( 'NONE', #566, #5961 ) ;
#19093=DIRECTION ( 'NONE',  ( -0.000000000000000000, -0.000000000000000000, -1.000000000000000000 ) ) ;
#19095=ORIENTED_EDGE ( 'NONE', *, *, #1271, .T. ) ;
#19096=CARTESIAN_POINT ( 'NONE',  ( -60.00000000000000000, -2.094888803305880013E-13, -105.0000000000000142 ) ) ;
#19097=CARTESIAN_POINT ( 'NONE',  ( 131.9720262563627386, -88.11726332927526073, 39.76694218959185179 ) ) ;
#19099=EDGE_LOOP ( 'NONE', ( #16833, #16505 ) ) ;
#19107=CARTESIAN_POINT ( 'NONE',  ( 78.68887634719571622, -147.8252249328912740, 39.99999999999999289 ) ) ;
#19109=DIRECTION ( 'NONE',  ( -1.000000000000000000, 0.000000000000000000, 0.000000000000000000 ) ) ;
#19117=CIRCLE ( 'NONE', #9306, 150.0000000000000284 ) ;
#19121=CYLINDRICAL_SURFACE ( 'NONE', #15940, 77.50000000000000000 ) ;
#19126=EDGE_LOOP ( 'NONE', ( #1859, #15680, #8966 ) ) ;
#19128=EDGE_CURVE ( 'NONE', #14061, #4447, #7567, .T. ) ;
#19130=ORIENTED_EDGE ( 'NONE', *, *, #14000, .T. ) ;
#19137=EDGE_CURVE ( 'NONE', #6494, #17725, #6054, .T. ) ;
#19138=CARTESIAN_POINT ( 'NONE',  ( 128.2779226595531270, 102.2982297021113141, 39.99999999999999289 ) ) ;
#19139=EDGE_CURVE ( 'NONE', #5750, #17792, #10628, .T. ) ;
#19143=DIRECTION ( 'NONE',  ( -1.000000000000000000, 0.000000000000000000, 0.000000000000000000 ) ) ;
#19145=DIRECTION ( 'NONE',  ( -1.000000000000000000, 0.000000000000000000, 0.000000000000000000 ) ) ;
#19146=CARTESIAN_POINT ( 'NONE',  ( 104.7095274995394476, -123.3473593051514712, 39.62101268589415071 ) ) ;
#19149=CARTESIAN_POINT ( 'NONE',  ( -70.15307277190674995, 132.5841624150375537, 1.385989013561256256 ) ) ;
#19157=CARTESIAN_POINT ( 'NONE',  ( -130.4176214210902742, 74.25971850835314569, 39.51174342451745503 ) ) ;
#19160=PLANE ( 'NONE',  #2100 ) ;
#19161=CARTESIAN_POINT ( 'NONE',  ( -97.99247315425149907, -133.3057953413762959, 6.895088020211351143 ) ) ;
#19163=ADVANCED_FACE ( 'NONE', ( #18428 ), #8461, .T. ) ;
#19167=CARTESIAN_POINT ( 'NONE',  ( -137.6931958989253530, 25.38413297918773637, 26.40985621151910223 ) ) ;
#19168=EDGE_CURVE ( 'NONE', #6419, #17764, #17668, .T. ) ;
#19171=CARTESIAN_POINT ( 'NONE',  ( -149.6969151468569237, 9.843262213762972834, -0.07667390253797667921 ) ) ;
#19173=CARTESIAN_POINT ( 'NONE',  ( -156.4179374840092862, -52.02840013024096066, 49.99999999999999289 ) ) ;
#19177=DIRECTION ( 'NONE',  ( -0.000000000000000000, -1.000000000000000000, -0.000000000000000000 ) ) ;
#19183=CARTESIAN_POINT ( 'NONE',  ( -110.0000000000000142, 275.0000000000000000, -75.00000000000000000 ) ) ;
#19185=CARTESIAN_POINT ( 'NONE',  ( -134.9252074077219561, -65.53799637400004485, 6.377149655367134073 ) ) ;
#19189=VERTEX_POINT ( 'NONE', #7978 ) ;
#19190=FACE_OUTER_BOUND ( 'NONE', #12776, .T. ) ;
#19202=ORIENTED_EDGE ( 'NONE', *, *, #1788, .T. ) ;
#19207=CARTESIAN_POINT ( 'NONE',  ( -100.6969204557047846, -129.5542747642292056, 37.33635527552283406 ) ) ;
#19211=CARTESIAN_POINT ( 'NONE',  ( 126.7720928841326042, -80.18313274224124143, -9.038567162788339715 ) ) ;
#19223=CARTESIAN_POINT ( 'NONE',  ( 84.00455766787162304, -124.2712478689755500, 38.95858097086686200 ) ) ;
#19228=ORIENTED_EDGE ( 'NONE', *, *, #10693, .T. ) ;
#19231=EDGE_CURVE ( 'NONE', #3673, #2735, #3483, .T. ) ;
#19245=ADVANCED_FACE ( 'NONE', ( #3385 ), #11100, .F. ) ;
#19247=CARTESIAN_POINT ( 'NONE',  ( 110.0000000000000142, 0.000000000000000000, -49.99999999999999289 ) ) ;
#19251=ORIENTED_EDGE ( 'NONE', *, *, #5654, .T. ) ;
#19253=CARTESIAN_POINT ( 'NONE',  ( -79.73494653235651697, 127.0540928074882459, 31.16759418789822433 ) ) ;
#19258=EDGE_CURVE ( 'NONE', #11724, #19796, #14223, .T. ) ;
#19259=EDGE_CURVE ( 'NONE', #18380, #13478, #2298, .T. ) ;
#19263=AXIS2_PLACEMENT_3D ( 'NONE', #11597, #15067, #17957 ) ;
#19265=ORIENTED_EDGE ( 'NONE', *, *, #10883, .T. ) ;
#19268=CARTESIAN_POINT ( 'NONE',  ( -83.54968581051868171, -124.5775662629353775, 2.083218535794355120 ) ) ;
#19272=DIRECTION ( 'NONE',  ( 1.000000000000000000, 0.000000000000000000, 0.000000000000000000 ) ) ;
#19278=ORIENTED_EDGE ( 'NONE', *, *, #16159, .F. ) ;
#19283=ORIENTED_EDGE ( 'NONE', *, *, #18884, .F. ) ;
#19294=CARTESIAN_POINT ( 'NONE',  ( 99.75239863728837975, -130.9022835076664535, 36.33312741211197761 ) ) ;
#19297=CIRCLE ( 'NONE', #10142, 7.500000000000007105 ) ;
#19298=VECTOR ( 'NONE', #14654, 1000.000000000000000 ) ;
#19328=CARTESIAN_POINT ( 'NONE',  ( 144.1955966362266679, 102.2982297021113141, 39.99999999999999289 ) ) ;
#19332=CYLINDRICAL_SURFACE ( 'NONE', #9328, 150.0000000000000284 ) ;
#19336=CARTESIAN_POINT ( 'NONE',  ( 99.75421581617496258, -130.9036673766147487, 3.638531688318945356 ) ) ;
#19340=FACE_OUTER_BOUND ( 'NONE', #9015, .T. ) ;
#19341=DIRECTION ( 'NONE',  ( 0.000000000000000000, 0.000000000000000000, 1.000000000000000000 ) ) ;
#19350=PRODUCT_CONTEXT ( 'NONE', #9854, 'mechanical' ) ;
#19353=CARTESIAN_POINT ( 'NONE',  ( 32.50000000000000000, 3.980102097228897837E-15, 49.99999999999999289 ) ) ;
#19358=CARTESIAN_POINT ( 'NONE',  ( -82.84981732090430739, -125.0436758660649303, 4.143355716251761578 ) ) ;
#19359=VERTEX_POINT ( 'NONE', #6855 ) ;
#19364=EDGE_CURVE ( 'NONE', #19032, #12392, #4938, .T. ) ;
#19365=( NAMED_UNIT ( * ) SI_UNIT ( $, .STERADIAN. ) SOLID_ANGLE_UNIT ( ) );
#19366=DIRECTION ( 'NONE',  ( -1.000000000000000000, 0.000000000000000000, 0.000000000000000000 ) ) ;
#19373=VECTOR ( 'NONE', #16867, 1000.000000000000000 ) ;
#19375=EDGE_CURVE ( 'NONE', #6851, #6330, #11460, .T. ) ;
#19386=CARTESIAN_POINT ( 'NONE',  ( -131.5110516633150155, -72.14693729183379389, -4.447104364459081083 ) ) ;
#19390=VECTOR ( 'NONE', #9807, 1000.000000000000000 ) ;
#19404=FACE_OUTER_BOUND ( 'NONE', #1730, .T. ) ;
#19410=ORIENTED_EDGE ( 'NONE', *, *, #9541, .F. ) ;
#19412=CARTESIAN_POINT ( 'NONE',  ( 0.000000000000000000, 60.00000000000000000, -105.0000000000000142 ) ) ;
#19423=EDGE_CURVE ( 'NONE', #5032, #3673, #2324, .T. ) ;
#19427=ORIENTED_EDGE ( 'NONE', *, *, #4652, .T. ) ;
#19429=FACE_OUTER_BOUND ( 'NONE', #10346, .T. ) ;
#19436=ORIENTED_EDGE ( 'NONE', *, *, #13137, .F. ) ;
#19438=CARTESIAN_POINT ( 'NONE',  ( 98.02376510503435725, -133.2645000753678630, 6.774075666499015824 ) ) ;
#19441=CARTESIAN_POINT ( 'NONE',  ( 138.2024300533213932, 89.85329105948596862, 39.99999999999999289 ) ) ;
#19443=CARTESIAN_POINT ( 'NONE',  ( 82.06839719201975925, -125.5578986320909678, 8.548731919517461364 ) ) ;
#19448=CARTESIAN_POINT ( 'NONE',  ( 141.8871031824808995, -16.05777877957299538, 39.99999999999999289 ) ) ;
#19457=FACE_OUTER_BOUND ( 'NONE', #7961, .T. ) ;
#19458=CARTESIAN_POINT ( 'NONE',  ( -97.05807359151792468, -115.6610107837965842, 10.36068692573858563 ) ) ;
#19461=( BOUNDED_CURVE ( )  B_SPLINE_CURVE ( 3, ( #9882, #8623, #14858, #13309 ),
 .UNSPECIFIED., .F., .F. ) 
 B_SPLINE_CURVE_WITH_KNOTS ( ( 4, 4 ),
 ( 1.570796326794896336, 1.920639998745670818 ),
 .UNSPECIFIED. ) 
 CURVE ( )  GEOMETRIC_REPRESENTATION_ITEM ( )  RATIONAL_B_SPLINE_CURVE ( ( 1.000000000000000000, 0.9898267632596812193, 0.9898267632596812193, 1.000000000000000000 ) ) 
 REPRESENTATION_ITEM ( '' )  );
#19462=LINE ( 'NONE', #7368, #5683 ) ;
#19468=ORIENTED_EDGE ( 'NONE', *, *, #7253, .F. ) ;
#19470=CARTESIAN_POINT ( 'NONE',  ( 128.2779226595531270, 102.2982297021113141, 39.99999999999999289 ) ) ;
#19477=VECTOR ( 'NONE', #5462, 1000.000000000000000 ) ;
#19486=EDGE_CURVE ( 'NONE', #5706, #12395, #20208, .T. ) ;
#19490=CIRCLE ( 'NONE', #17860, 42.50000000000000000 ) ;
#19497=DIRECTION ( 'NONE',  ( -0.9009688679024160374, -0.4338837391175646707, 0.000000000000000000 ) ) ;
#19515=ORIENTED_EDGE ( 'NONE', *, *, #5783, .F. ) ;
#19517=ORIENTED_EDGE ( 'NONE', *, *, #3690, .T. ) ;
#19526=ORIENTED_EDGE ( 'NONE', *, *, #3109, .T. ) ;
#19527=CARTESIAN_POINT ( 'NONE',  ( -129.8775639978177594, -75.04816271247872805, 46.61694955171623178 ) ) ;
#19535=CARTESIAN_POINT ( 'NONE',  ( 90.16928584620099230, -119.8796671366211939, -6.536607213163578400 ) ) ;
#19536=DIRECTION ( 'NONE',  ( 1.000000000000000000, 0.000000000000000000, 0.000000000000000000 ) ) ;
#19543=ORIENTED_EDGE ( 'NONE', *, *, #13785, .T. ) ;
#19544=EDGE_CURVE ( 'NONE', #7600, #19595, #2966, .T. ) ;
#19546=ORIENTED_EDGE ( 'NONE', *, *, #19128, .T. ) ;
#19547=CARTESIAN_POINT ( 'NONE',  ( 93.96728894854133785, -116.9213660262077781, -8.642061447020635612 ) ) ;
#19548=CARTESIAN_POINT ( 'NONE',  ( -99.15855529360358389, -131.7281685730150684, 4.481768808781215085 ) ) ;
#19549=AXIS2_PLACEMENT_3D ( 'NONE', #6997, #8628, #6805 ) ;
#19553=CARTESIAN_POINT ( 'NONE',  ( -88.72241907111768455, -120.9490000788567130, -5.329395631252526577 ) ) ;
#19564=ORIENTED_EDGE ( 'NONE', *, *, #19885, .F. ) ;
#19567=CARTESIAN_POINT ( 'NONE',  ( 134.7088403748421399, -73.01573503433813528, 9.021076383413966226 ) ) ;
#19569=( BOUNDED_CURVE ( )  B_SPLINE_CURVE ( 3, ( #9160, #18582, #18690, #13861 ),
 .UNSPECIFIED., .F., .F. ) 
 B_SPLINE_CURVE_WITH_KNOTS ( ( 4, 4 ),
 ( -1.776356839400250465E-15, 1.570796326794896336 ),
 .UNSPECIFIED. ) 
 CURVE ( )  GEOMETRIC_REPRESENTATION_ITEM ( )  RATIONAL_B_SPLINE_CURVE ( ( 1.000000000000000000, 0.8047378541243646044, 0.8047378541243646044, 1.000000000000000000 ) ) 
 REPRESENTATION_ITEM ( '' )  );
#19570=CARTESIAN_POINT ( 'NONE',  ( -133.3415482518558122, -68.70949856429524516, -0.7195383986325173398 ) ) ;
#19571=CARTESIAN_POINT ( 'NONE',  ( -7.500000000000006217, 164.0736214083062805, 39.99999999999999289 ) ) ;
#19573=AXIS2_PLACEMENT_3D ( 'NONE', #13592, #1329, #8991 ) ;
#19577=CARTESIAN_POINT ( 'NONE',  ( -132.7526696464364875, -84.67545766722497547, 0.8872275965778846363 ) ) ;
#19581=CARTESIAN_POINT ( 'NONE',  ( -134.5816389422690236, -73.99824545063825099, 33.10625479714592956 ) ) ;
#19595=VERTEX_POINT ( 'NONE', #6313 ) ;
#19601=CIRCLE ( 'NONE', #3919, 7.500000000000008882 ) ;
#19613=ORIENTED_EDGE ( 'NONE', *, *, #9143, .T. ) ;
#19614=ORIENTED_EDGE ( 'NONE', *, *, #272, .F. ) ;
#19623=DIRECTION ( 'NONE',  ( 0.000000000000000000, 0.000000000000000000, -1.000000000000000000 ) ) ;
#19630=CARTESIAN_POINT ( 'NONE',  ( 84.98223365279407915, -123.6049511534864536, -0.7930668616445250008 ) ) ;
#19631=AXIS2_PLACEMENT_3D ( 'NONE', #10973, #13631, #12505 ) ;
#19634=EDGE_CURVE ( 'NONE', #3485, #4464, #17683, .T. ) ;
#19639=AXIS2_PLACEMENT_3D ( 'NONE', #7810, #2809, #7598 ) ;
#19648=CARTESIAN_POINT ( 'NONE',  ( 7.500000000000006217, 164.0736214083062805, 39.99999999999999289 ) ) ;
#19650=DIRECTION ( 'NONE',  ( 0.6234898018587442525, -0.7818314824680211439, 0.000000000000000000 ) ) ;
#19651=EDGE_CURVE ( 'NONE', #3485, #20118, #14179, .T. ) ;
#19657=DIRECTION ( 'NONE',  ( 0.000000000000000000, 0.000000000000000000, -1.000000000000000000 ) ) ;
#19658=EDGE_LOOP ( 'NONE', ( #4032, #18831, #17949, #12007 ) ) ;
#19674=CARTESIAN_POINT ( 'NONE',  ( -126.7530218919690412, -80.25302646196961120, -0.9824221781708450951 ) ) ;
#19675=CARTESIAN_POINT ( 'NONE',  ( 133.2712073793125285, -68.96827650305598922, 10.00000000000000711 ) ) ;
#19679=CARTESIAN_POINT ( 'NONE',  ( -110.0000000000000142, 265.0000000000000000, 44.99999999999998579 ) ) ;
#19685=VECTOR ( 'NONE', #1450, 1000.000000000000000 ) ;
#19687=ORIENTED_EDGE ( 'NONE', *, *, #5367, .T. ) ;
#19690=ORIENTED_EDGE ( 'NONE', *, *, #18916, .F. ) ;
#19696=CARTESIAN_POINT ( 'NONE',  ( 141.8714406926368099, -48.70825716237079916, 39.99999999999999289 ) ) ;
#19697=CARTESIAN_POINT ( 'NONE',  ( -131.9720262563626818, -88.11726332927524652, 0.2330578104081588442 ) ) ;
#19699=CARTESIAN_POINT ( 'NONE',  ( 122.8001410695374886, -86.14014948502062907, 50.00000000000000000 ) ) ;
#19702=DIRECTION ( 'NONE',  ( -1.000000000000000000, 0.000000000000000000, 0.000000000000000000 ) ) ;
#19704=VECTOR ( 'NONE', #10178, 1000.000000000000000 ) ;
#19711=EDGE_CURVE ( 'NONE', #16974, #13478, #4860, .T. ) ;
#19718=CARTESIAN_POINT ( 'NONE',  ( -133.9144309718294892, -67.58001956112551056, 38.90204870918451263 ) ) ;
#19726=CARTESIAN_POINT ( 'NONE',  ( -130.9868171408399462, -91.88282611735537841, 40.00000000000000000 ) ) ;
#19728=ORIENTED_EDGE ( 'NONE', *, *, #1015, .F. ) ;
#19729=ADVANCED_FACE ( 'NONE', ( #14967 ), #13122, .F. ) ;
#19731=CARTESIAN_POINT ( 'NONE',  ( 159.9599531637113330, -36.50981547336952104, 39.99999999999999289 ) ) ;
#19733=ORIENTED_EDGE ( 'NONE', *, *, #9143, .F. ) ;
#19734=CARTESIAN_POINT ( 'NONE',  ( -96.95682486762434849, -115.7027609144189597, 29.61261940427053929 ) ) ;
#19736=ORIENTED_EDGE ( 'NONE', *, *, #2883, .T. ) ;
#19737=CYLINDRICAL_SURFACE ( 'NONE', #645, 9.999999999999994671 ) ;
#19741=ORIENTED_EDGE ( 'NONE', *, *, #10990, .F. ) ;
#19742=ADVANCED_FACE ( 'NONE', ( #5569 ), #11888, .T. ) ;
#19743=CARTESIAN_POINT ( 'NONE',  ( 100.7812500000000284, -111.0996833858562809, -3.469446951953614189E-15 ) ) ;
#19746=VECTOR ( 'NONE', #6433, 1000.000000000000000 ) ;
#19758=ORIENTED_EDGE ( 'NONE', *, *, #3641, .T. ) ;
#19765=EDGE_CURVE ( 'NONE', #14077, #22, #10170, .T. ) ;
#19766=CARTESIAN_POINT ( 'NONE',  ( 133.6084294554693770, -80.28749220512219154, 2.341744974304089233 ) ) ;
#19769=CARTESIAN_POINT ( 'NONE',  ( -100.7812499999999716, -111.0996833858563093, 40.00000000000001421 ) ) ;
#19773=DIRECTION ( 'NONE',  ( 0.000000000000000000, 0.000000000000000000, 1.000000000000000000 ) ) ;
#19774=FACE_BOUND ( 'NONE', #18621, .T. ) ;
#19775=CARTESIAN_POINT ( 'NONE',  ( 125.5830613944035576, -82.05591916721346024, -1.021718221178191222 ) ) ;
#19777=CARTESIAN_POINT ( 'NONE',  ( 97.50000000000002842, -189.9999999999999716, 40.00000000000000000 ) ) ;
#19778=FACE_OUTER_BOUND ( 'NONE', #6992, .T. ) ;
#19779=EDGE_LOOP ( 'NONE', ( #17324, #1858, #68, #16349, #4460, #19526 ) ) ;
#19784=VECTOR ( 'NONE', #2424, 1000.000000000000000 ) ;
#19794=DIRECTION ( 'NONE',  ( 0.2225209339563183342, -0.9749279121818226201, 0.000000000000000000 ) ) ;
#19796=VERTEX_POINT ( 'NONE', #10454 ) ;
#19799=CARTESIAN_POINT ( 'NONE',  ( -130.9868171408399462, -91.88282611735539263, 0.000000000000000000 ) ) ;
#19802=CARTESIAN_POINT ( 'NONE',  ( 133.5342034995476297, -80.71481093439410870, 37.85466313993502041 ) ) ;
#19816=ORIENTED_EDGE ( 'NONE', *, *, #9024, .T. ) ;
#19819=VERTEX_POINT ( 'NONE', #8539 ) ;
#19823=CARTESIAN_POINT ( 'NONE',  ( -71.18887634719365565, -147.8252249328922687, 39.99999999999999289 ) ) ;
#19825=DIRECTION ( 'NONE',  ( 0.000000000000000000, 0.000000000000000000, 1.000000000000000000 ) ) ;
#19826=CARTESIAN_POINT ( 'NONE',  ( -133.1920331248151399, -82.53376026279585176, 38.51313858039918614 ) ) ;
#19829=FACE_OUTER_BOUND ( 'NONE', #19779, .T. ) ;
#19832=ORIENTED_EDGE ( 'NONE', *, *, #9514, .T. ) ;
#19833=CARTESIAN_POINT ( 'NONE',  ( -97.67167802517903397, -133.7293924297442800, 31.85450751873280240 ) ) ;
#19840=CARTESIAN_POINT ( 'NONE',  ( 89.41054993672092621, -120.4453604907671718, -5.957062783365469016 ) ) ;
#19845=DIRECTION ( 'NONE',  ( -0.000000000000000000, -0.000000000000000000, 1.000000000000000000 ) ) ;
#19848=AXIS2_PLACEMENT_3D ( 'NONE', #15151, #20062, #10845 ) ;
#19852=DIRECTION ( 'NONE',  ( -1.000000000000000000, 0.000000000000000000, 0.000000000000000000 ) ) ;
#19857=EDGE_CURVE ( 'NONE', #3067, #19189, #10535, .T. ) ;
#19863=CARTESIAN_POINT ( 'NONE',  ( 0.000000000000000000, 0.000000000000000000, -100.0000000000000000 ) ) ;
#19866=CARTESIAN_POINT ( 'NONE',  ( 134.2294018150276145, -76.49442575693798574, 4.443041126027487131 ) ) ;
#19870=DIRECTION ( 'NONE',  ( 0.000000000000000000, 0.000000000000000000, -1.000000000000000000 ) ) ;
#19873=CARTESIAN_POINT ( 'NONE',  ( -134.6114153021046320, -66.18050771012671873, 4.130514097776864624 ) ) ;
#19874=CARTESIAN_POINT ( 'NONE',  ( 129.0008258633897640, -76.61840651136441238, -0.1009346208872797107 ) ) ;
#19876=CARTESIAN_POINT ( 'NONE',  ( -166.7850001792984926, -190.0000000000000284, 40.00000000000000000 ) ) ;
#19879=CARTESIAN_POINT ( 'NONE',  ( 97.50000000000002842, -195.8578643762690206, 35.85786437626904188 ) ) ;
#19880=AXIS2_PLACEMENT_3D ( 'NONE', #19138, #13077, #16469 ) ;
#19881=ORIENTED_EDGE ( 'NONE', *, *, #7661, .F. ) ;
#19885=EDGE_CURVE ( 'NONE', #7332, #1702, #2907, .T. ) ;
#19893=EDGE_CURVE ( 'NONE', #2847, #4825, #3944, .T. ) ;
#19897=CARTESIAN_POINT ( 'NONE',  ( -167.4599531637108782, -36.50981547337168109, 49.99999999999999289 ) ) ;
#19900=CARTESIAN_POINT ( 'NONE',  ( -108.6450314030896891, 75.64087399529431366, -29.99999999999949196 ) ) ;
#19902=LINE ( 'NONE', #13549, #18591 ) ;
#19905=CARTESIAN_POINT ( 'NONE',  ( 132.2990932590224702, -86.73761849286395886, 39.55987232456632086 ) ) ;
#19906=CARTESIAN_POINT ( 'NONE',  ( 144.1130761623740568, -69.50842595698583182, 49.99999999999999289 ) ) ;
#19907=CIRCLE ( 'NONE', #19573, 15.91767397667354444 ) ;
#19909=CARTESIAN_POINT ( 'NONE',  ( -176.5810126522742394, -187.6736222527391647, 31.17213215707407414 ) ) ;
#19910=ORIENTED_EDGE ( 'NONE', *, *, #5991, .F. ) ;
#19911=ADVANCED_FACE ( 'NONE', ( #9243 ), #7396, .T. ) ;
#19915=DIRECTION ( 'NONE',  ( -0.2225209339563195554, 0.9749279121818223981, 0.000000000000000000 ) ) ;
#19917=CARTESIAN_POINT ( 'NONE',  ( 123.8492616149702741, -72.31991210363503342, 10.00000000000000178 ) ) ;
#19919=ORIENTED_EDGE ( 'NONE', *, *, #9270, .F. ) ;
#19920=AXIS2_PLACEMENT_3D ( 'NONE', #15481, #1152, #7393 ) ;
#19923=ORIENTED_EDGE ( 'NONE', *, *, #11106, .F. ) ;
#19929=CARTESIAN_POINT ( 'NONE',  ( -134.6261364156839591, -73.66016459667358163, 32.57698633332318394 ) ) ;
#19931=ORIENTED_EDGE ( 'NONE', *, *, #10405, .T. ) ;
#19938=EDGE_LOOP ( 'NONE', ( #9893, #15201, #13535, #12586, #190, #7086, #7058, #11271, #8039 ) ) ;
#19944=CARTESIAN_POINT ( 'NONE',  ( 83.97601510867102093, -124.2902204837746893, 1.122958062864681583 ) ) ;
#19948=DIRECTION ( 'NONE',  ( 0.000000000000000000, 0.000000000000000000, 1.000000000000000000 ) ) ;
#19953=CARTESIAN_POINT ( 'NONE',  ( 82.03125000078792084, -125.5821405427867461, 31.51013335451832731 ) ) ;
#19970=CARTESIAN_POINT ( 'NONE',  ( 86.01343624116272224, 31.38211805825951473, 40.00000000000000000 ) ) ;
#19977=CARTESIAN_POINT ( 'NONE',  ( 144.1955966362266679, 102.2982297021113141, 49.99999999999999289 ) ) ;
#19978=CARTESIAN_POINT ( 'NONE',  ( 130.9519479124748784, -73.15688856708820254, -5.283951177996526027 ) ) ;
#19982=FACE_OUTER_BOUND ( 'NONE', #16796, .T. ) ;
#19989=AXIS2_PLACEMENT_3D ( 'NONE', #1989, #8216, #16205 ) ;
#19990=FACE_OUTER_BOUND ( 'NONE', #19938, .T. ) ;
#19996=EDGE_CURVE ( 'NONE', #12285, #1203, #1335, .T. ) ;
#19997=ORIENTED_EDGE ( 'NONE', *, *, #11265, .T. ) ;
#19999=CARTESIAN_POINT ( 'NONE',  ( 60.00000000000000711, 6.284666409917639535E-13, -100.0000000000000000 ) ) ;
#20008=EDGE_CURVE ( 'NONE', #8838, #16933, #14417, .T. ) ;
#20012=ORIENTED_EDGE ( 'NONE', *, *, #9416, .F. ) ;
#20029=CARTESIAN_POINT ( 'NONE',  ( -77.12898346057446020, 127.7594922753211080, -17.80027040494307400 ) ) ;
#20030=LINE ( 'NONE', #7443, #5841 ) ;
#20032=CIRCLE ( 'NONE', #1736, 7.500000000000006217 ) ;
#20036=CARTESIAN_POINT ( 'NONE',  ( -134.2873401242900968, -76.10409495552310943, 35.26608652156301815 ) ) ;
#20037=CARTESIAN_POINT ( 'NONE',  ( -101.1986828041967499, 96.79850148450320546, 38.95247587951536872 ) ) ;
#20044=CARTESIAN_POINT ( 'NONE',  ( -82.03124999999998579, -125.5821405433014348, 30.00000000000001776 ) ) ;
#20047=CARTESIAN_POINT ( 'NONE',  ( -113.9638382236393710, 83.66658905436058546, -34.85447305243185667 ) ) ;
#20048=DIRECTION ( 'NONE',  ( -0.000000000000000000, -0.000000000000000000, -1.000000000000000000 ) ) ;
#20051=CARTESIAN_POINT ( 'NONE',  ( 98.61806909068849336, -132.4668554876670896, 5.401815755557273668 ) ) ;
#20054=CARTESIAN_POINT ( 'NONE',  ( -138.0190094366552387, -24.44405370507808328, -10.87470759034249745 ) ) ;
#20058=DIRECTION ( 'NONE',  ( 0.000000000000000000, 0.000000000000000000, -1.000000000000000000 ) ) ;
#20060=CARTESIAN_POINT ( 'NONE',  ( 95.49560220035800739, -115.9193184531417131, 33.43809937674511445 ) ) ;
#20061=ORIENTED_EDGE ( 'NONE', *, *, #12135, .T. ) ;
#20062=DIRECTION ( 'NONE',  ( 0.000000000000000000, 1.000000000000000000, -0.000000000000000000 ) ) ;
#20064=ORIENTED_EDGE ( 'NONE', *, *, #5007, .T. ) ;
#20068=ORIENTED_EDGE ( 'NONE', *, *, #19033, .T. ) ;
#20069=DIRECTION ( 'NONE',  ( -0.000000000000000000, -0.000000000000000000, -1.000000000000000000 ) ) ;
#20072=CARTESIAN_POINT ( 'NONE',  ( 56.84754764479240663, -154.7316448359447634, 39.99999999999999289 ) ) ;
#20074=LINE ( 'NONE', #19970, #7464 ) ;
#20080=CARTESIAN_POINT ( 'NONE',  ( -134.0645693066666411, -77.56608579646530188, 3.731507865007667846 ) ) ;
#20081=CARTESIAN_POINT ( 'NONE',  ( 130.5436973595105030, -73.98181611796424306, 1.254900387872837531 ) ) ;
#20082=DIRECTION ( 'NONE',  ( 0.000000000000000000, 0.000000000000000000, 1.000000000000000000 ) ) ;
#20083=CARTESIAN_POINT ( 'NONE',  ( 126.5370453525553955, 80.55045718954892209, 49.99999999999999289 ) ) ;
#20084=CARTESIAN_POINT ( 'NONE',  ( -132.3196846491782424, -70.65764850136368125, 43.06549271861968720 ) ) ;
#20087=AXIS2_PLACEMENT_3D ( 'NONE', #17506, #17900, #8279 ) ;
#20096=ORIENTED_EDGE ( 'NONE', *, *, #8554, .F. ) ;
#20098=DIRECTION ( 'NONE',  ( -0.000000000000000000, 0.000000000000000000, -1.000000000000000000 ) ) ;
#20104=DIRECTION ( 'NONE',  ( -1.000000000000000000, 0.000000000000000000, 0.000000000000000000 ) ) ;
#20105=DIRECTION ( 'NONE',  ( 0.000000000000000000, -1.000000000000000000, 0.000000000000000000 ) ) ;
#20107=CARTESIAN_POINT ( 'NONE',  ( 132.9648440817097708, -83.65857578542980377, 38.84409438298517614 ) ) ;
#20109=ORIENTED_EDGE ( 'NONE', *, *, #18159, .T. ) ;
#20118=VERTEX_POINT ( 'NONE', #17340 ) ;
#20127=CIRCLE ( 'NONE', #10654, 99.99999999999997158 ) ;
#20128=ADVANCED_FACE ( 'NONE', ( #17542 ), #8312, .T. ) ;
#20129=CARTESIAN_POINT ( 'NONE',  ( 0.000000000000000000, 0.000000000000000000, -100.0000000000000000 ) ) ;
#20135=CARTESIAN_POINT ( 'NONE',  ( -82.10917641232227027, 113.4001070177828154, 26.20091274746184240 ) ) ;
#20140=ADVANCED_FACE ( 'NONE', ( #12712 ), #6793, .T. ) ;
#20141=AXIS2_PLACEMENT_3D ( 'NONE', #5299, #3659, #11123 ) ;
#20146=CARTESIAN_POINT ( 'NONE',  ( -96.67521566530153621, -115.8170149451950692, 29.68188518566230982 ) ) ;
#20149=CARTESIAN_POINT ( 'NONE',  ( -136.3855242278113735, 54.99785135045119944, -25.06786605331940621 ) ) ;
#20152=CARTESIAN_POINT ( 'NONE',  ( 99.35210738963728261, -131.4612102079554177, 4.192299627536158368 ) ) ;
#20161=PLANE ( 'NONE',  #12154 ) ;
#20162=CARTESIAN_POINT ( 'NONE',  ( 82.03125000000002842, -125.5821405433014064, 30.00000000000000000 ) ) ;
#20168=ORIENTED_EDGE ( 'NONE', *, *, #6018, .T. ) ;
#20172=EDGE_CURVE ( 'NONE', #4825, #15881, #4000, .T. ) ;
#20173=CARTESIAN_POINT ( 'NONE',  ( -103.4088548222096620, -125.4447869035480210, 0.8709733734652972403 ) ) ;
#20178=CARTESIAN_POINT ( 'NONE',  ( -97.49999999999997158, -115.4778303846450029, 10.00000000000000355 ) ) ;
#20181=CARTESIAN_POINT ( 'NONE',  ( -96.21889527877688408, -115.1753595937449575, 35.54861044090515776 ) ) ;
#20186=CARTESIAN_POINT ( 'NONE',  ( 125.0010599886705620, -82.93257931482615675, -0.9426074830654761483 ) ) ;
#20188=LINE ( 'NONE', #8930, #14620 ) ;
#20189=CARTESIAN_POINT ( 'NONE',  ( -131.8276101104381439, -71.67687255337297358, 36.69851420954442744 ) ) ;
#20190=ORIENTED_EDGE ( 'NONE', *, *, #2883, .F. ) ;
#20191=DIRECTION ( 'NONE',  ( -0.000000000000000000, -0.000000000000000000, -1.000000000000000000 ) ) ;
#20194=ORIENTED_EDGE ( 'NONE', *, *, #220, .T. ) ;
#20195=ORIENTED_EDGE ( 'NONE', *, *, #4033, .F. ) ;
#20204=CARTESIAN_POINT ( 'NONE',  ( -96.45829176898665480, 93.78223209612394839, -27.30616533434335480 ) ) ;
#20206=DIRECTION ( 'NONE',  ( -1.000000000000000000, 0.000000000000000000, 0.000000000000000000 ) ) ;
#20208=LINE ( 'NONE', #1002, #14399 ) ;
#20220=FACE_OUTER_BOUND ( 'NONE', #12032, .T. ) ;
#20225=CARTESIAN_POINT ( 'NONE',  ( -71.18887634719365565, -147.8252249328922687, 49.99999999999999289 ) ) ;
#20226=DIRECTION ( 'NONE',  ( -1.000000000000000000, 0.000000000000000000, 0.000000000000000000 ) ) ;
#20229=DIRECTION ( 'NONE',  ( 0.000000000000000000, 0.000000000000000000, 1.000000000000000000 ) ) ;
#20231=( BOUNDED_SURFACE ( )  B_SPLINE_SURFACE ( 3, 2, ( 
 ( #20162, #4512, #17098 ),
 ( #19953, #13917, #4829 ),
 ( #3293, #4410, #18433 ),
 ( #1343, #10637, #14023 ),
 ( #6364, #12582, #4618 ),
 ( #2985, #18845, #10744 ),
 ( #4722, #112, #1447 ),
 ( #12277, #7781, #9321 ),
 ( #10948, #16893, #7883 ),
 ( #5954, #15351, #12173 ),
 ( #17316, #15671, #3087 ),
 ( #2881, #16, #6266 ),
 ( #9528, #1234, #10842 ),
 ( #9213, #7472, #17000 ),
 ( #3189, #13712, #7678 ),
 ( #18531, #12478, #15564 ),
 ( #9426, #9108, #7571 ),
 ( #13814, #20060, #6060 ),
 ( #15457, #1656, #1550 ),
 ( #6163, #12382, #18742 ),
 ( #18643, #8289, #18953 ),
 ( #618, #9824, #9929 ),
 ( #12989, #17617, #5037 ),
 ( #12891, #11154, #19146 ),
 ( #12794, #5137, #17416 ),
 ( #3392, #3593, #314 ),
 ( #4939, #3689, #6671 ),
 ( #5329, #6766, #14229 ) ),
 .UNSPECIFIED., .F., .F., .F. ) 
 B_SPLINE_SURFACE_WITH_KNOTS ( ( 4, 2, 2, 2, 2, 2, 2, 2, 2, 2, 2, 2, 2, 4 ),
 ( 3, 3 ),
 ( 0.01172725363905311943, 0.01619455768277540397, 0.01731138369370597424, 0.01842820970463654451, 0.02066186172649768504, 0.02289551374835882558, 0.02401233975928939585, 0.02512916577021996958, 0.02959646981394225412, 0.03406377385766454213, 0.03629742587952568267, 0.03853107790138682320, 0.04299838194510910427, 0.04746568598883138534 ),
 ( 0.000000000000000000, 1.000000000000000000 ),
 .UNSPECIFIED. ) 
 GEOMETRIC_REPRESENTATION_ITEM ( )  RATIONAL_B_SPLINE_SURFACE ( (
 ( 1.000000000000000000, 0.4759858191164941243, 1.000000000000000000),
 ( 1.000000000000000000, 0.4759956267216851611, 1.000000000000000000),
 ( 1.000000000000000000, 0.4778541562206653492, 1.000000000000000000),
 ( 1.000000000000000000, 0.4823973722703661648, 1.000000000000000000),
 ( 1.000000000000000000, 0.4834178931537515544, 1.000000000000000000),
 ( 1.000000000000000000, 0.4856852555521312120, 1.000000000000000000),
 ( 1.000000000000000000, 0.4869309269815854657, 1.000000000000000000),
 ( 1.000000000000000000, 0.4909487690767815882, 1.000000000000000000),
 ( 1.000000000000000000, 0.4940161083580015822, 1.000000000000000000),
 ( 1.000000000000000000, 0.5008835903390461697, 1.000000000000000000),
 ( 1.000000000000000000, 0.5046839780478526993, 1.000000000000000000),
 ( 1.000000000000000000, 0.5109205925582556151, 1.000000000000000000),
 ( 1.000000000000000000, 0.5130943221001723620, 1.000000000000000000),
 ( 1.000000000000000000, 0.5175691686949387416, 1.000000000000000000),
 ( 1.000000000000000000, 0.5198746620752942027, 1.000000000000000000),
 ( 1.000000000000000000, 0.5317265360217148240, 1.000000000000000000),
 ( 1.000000000000000000, 0.5422380167217139002, 1.000000000000000000),
 ( 1.000000000000000000, 0.5650731438340860224, 1.000000000000000000),
 ( 1.000000000000000000, 0.5770759225151704808, 1.000000000000000000),
 ( 1.000000000000000000, 0.5957780208533433042, 1.000000000000000000),
 ( 1.000000000000000000, 0.6021295156453072561, 1.000000000000000000),
 ( 1.000000000000000000, 0.6150481322455569888, 1.000000000000000000),
 ( 1.000000000000000000, 0.6215784740535582609, 1.000000000000000000),
 ( 1.000000000000000000, 0.6411710492548771123, 1.000000000000000000),
 ( 1.000000000000000000, 0.6543107498257758614, 1.000000000000000000),
 ( 1.000000000000000000, 0.6806663510239792103, 1.000000000000000000),
 ( 1.000000000000000000, 0.6938871677789396619, 1.000000000000000000),
 ( 1.000000000000000000, 0.7071067811865474617, 1.000000000000000000) ) ) 
 REPRESENTATION_ITEM ( '' )  SURFACE ( )  );
#20239=DIRECTION ( 'NONE',  ( 0.000000000000000000, 0.000000000000000000, 1.000000000000000000 ) ) ;
#20242=DIRECTION ( 'NONE',  ( 0.000000000000000000, 0.000000000000000000, -1.000000000000000000 ) ) ;
ENDSEC;
END-ISO-10303-21;
